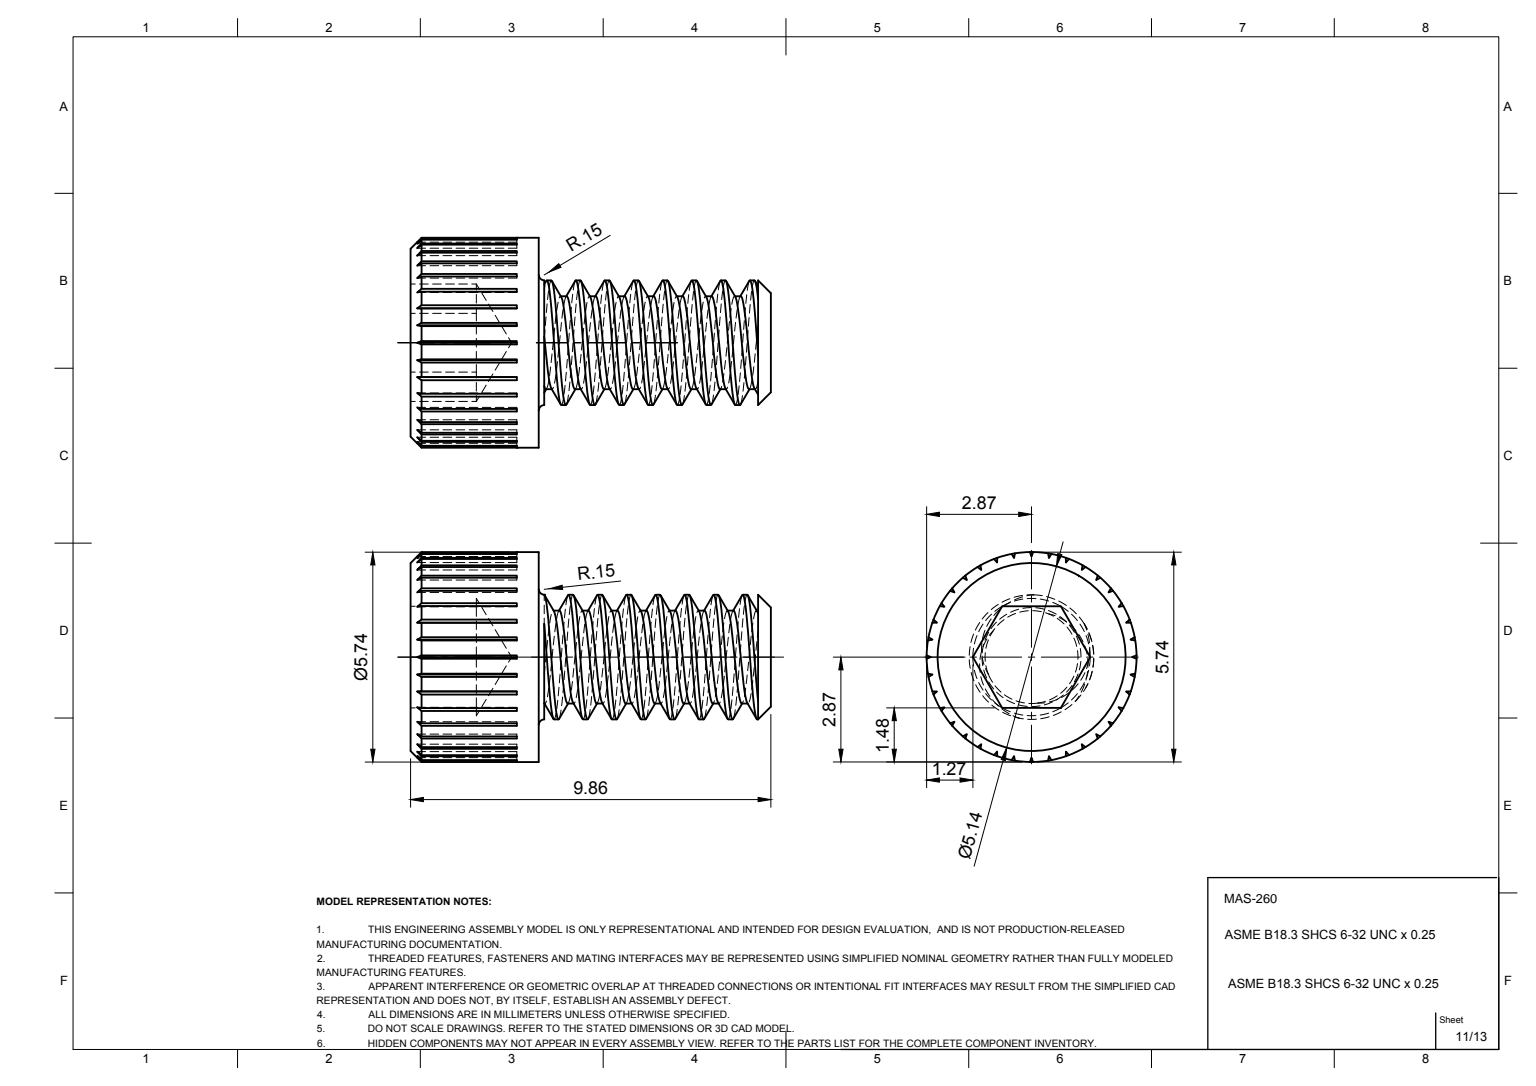
ISO-10303-21;
HEADER;
/* Generated by software containing ST-Developer
 * from STEP Tools, Inc. (www.steptools.com) 
 */

FILE_DESCRIPTION(
/* description */ (''),
/* implementation_level */ '2;1');

FILE_NAME(
/* name */ 'ASME B18.3 SHCS 6-32 UNC x 0.25.step',
/* time_stamp */ '2026-10-15T13:29:10-07:00',
/* author */ (''),
/* organization */ (''),
/* preprocessor_version */ 'ST-DEVELOPER v20.2',
/* originating_system */ 'Autodesk Translation Framework v15.15.0.0',
/* authorisation */ '');

FILE_SCHEMA (('AUTOMOTIVE_DESIGN { 1 0 10303 214 3 1 1 }'));
ENDSEC;

DATA;
#10=MECHANICAL_DESIGN_GEOMETRIC_PRESENTATION_REPRESENTATION('',(#942),#83219);
#281=(
BOUNDED_CURVE()
B_SPLINE_CURVE(2,(#58539,#58540,#58541),.UNSPECIFIED.,.F.,.F.)
B_SPLINE_CURVE_WITH_KNOTS((3,3),(0.,0.0169283274324264),.UNSPECIFIED.)
CURVE()
GEOMETRIC_REPRESENTATION_ITEM()
RATIONAL_B_SPLINE_CURVE((1.,1.00067437544971,1.00082963690249))
REPRESENTATION_ITEM('')
);
#282=(
BOUNDED_CURVE()
B_SPLINE_CURVE(2,(#58546,#58547,#58548),.UNSPECIFIED.,.F.,.F.)
B_SPLINE_CURVE_WITH_KNOTS((3,3),(0.0270544913418749,0.0439828187741895),
 .UNSPECIFIED.)
CURVE()
GEOMETRIC_REPRESENTATION_ITEM()
RATIONAL_B_SPLINE_CURVE((1.00082963691396,1.00067437545903,1.))
REPRESENTATION_ITEM('')
);
#283=(
BOUNDED_CURVE()
B_SPLINE_CURVE(2,(#58555,#58556,#58557),.UNSPECIFIED.,.F.,.F.)
B_SPLINE_CURVE_WITH_KNOTS((3,3),(0.0270544913418551,0.0439828187741901),
 .UNSPECIFIED.)
CURVE()
GEOMETRIC_REPRESENTATION_ITEM()
RATIONAL_B_SPLINE_CURVE((1.0008296369069,1.0006743754533,1.))
REPRESENTATION_ITEM('')
);
#284=(
BOUNDED_CURVE()
B_SPLINE_CURVE(2,(#58561,#58562,#58563),.UNSPECIFIED.,.F.,.F.)
B_SPLINE_CURVE_WITH_KNOTS((3,3),(0.,0.0169283274323742),.UNSPECIFIED.)
CURVE()
GEOMETRIC_REPRESENTATION_ITEM()
RATIONAL_B_SPLINE_CURVE((1.,1.00067437545167,1.0008296369049))
REPRESENTATION_ITEM('')
);
#285=(
BOUNDED_CURVE()
B_SPLINE_CURVE(2,(#58565,#58566,#58567),.UNSPECIFIED.,.F.,.F.)
B_SPLINE_CURVE_WITH_KNOTS((3,3),(0.0270544913418838,0.0439828187741893),
 .UNSPECIFIED.)
CURVE()
GEOMETRIC_REPRESENTATION_ITEM()
RATIONAL_B_SPLINE_CURVE((1.00082963690705,1.00067437545341,1.))
REPRESENTATION_ITEM('')
);
#286=(
BOUNDED_CURVE()
B_SPLINE_CURVE(2,(#58571,#58572,#58573),.UNSPECIFIED.,.F.,.F.)
B_SPLINE_CURVE_WITH_KNOTS((3,3),(0.,0.0169283274323636),.UNSPECIFIED.)
CURVE()
GEOMETRIC_REPRESENTATION_ITEM()
RATIONAL_B_SPLINE_CURVE((1.,1.00067437545192,1.00082963690521))
REPRESENTATION_ITEM('')
);
#287=(
BOUNDED_CURVE()
B_SPLINE_CURVE(2,(#58575,#58576,#58577),.UNSPECIFIED.,.F.,.F.)
B_SPLINE_CURVE_WITH_KNOTS((3,3),(0.0270544913418794,0.0439828187741893),
 .UNSPECIFIED.)
CURVE()
GEOMETRIC_REPRESENTATION_ITEM()
RATIONAL_B_SPLINE_CURVE((1.00082963691317,1.00067437545839,1.))
REPRESENTATION_ITEM('')
);
#288=(
BOUNDED_CURVE()
B_SPLINE_CURVE(2,(#58581,#58582,#58583),.UNSPECIFIED.,.F.,.F.)
B_SPLINE_CURVE_WITH_KNOTS((3,3),(0.,0.0169283274323019),.UNSPECIFIED.)
CURVE()
GEOMETRIC_REPRESENTATION_ITEM()
RATIONAL_B_SPLINE_CURVE((1.,1.0006743754572,1.00082963691171))
REPRESENTATION_ITEM('')
);
#289=(
BOUNDED_CURVE()
B_SPLINE_CURVE(2,(#58585,#58586,#58587),.UNSPECIFIED.,.F.,.F.)
B_SPLINE_CURVE_WITH_KNOTS((3,3),(0.0270544913418195,0.0439828187741896),
 .UNSPECIFIED.)
CURVE()
GEOMETRIC_REPRESENTATION_ITEM()
RATIONAL_B_SPLINE_CURVE((1.00082963691305,1.00067437545829,1.))
REPRESENTATION_ITEM('')
);
#290=(
BOUNDED_CURVE()
B_SPLINE_CURVE(2,(#58591,#58592,#58593),.UNSPECIFIED.,.F.,.F.)
B_SPLINE_CURVE_WITH_KNOTS((3,3),(0.,0.0169283274324256),.UNSPECIFIED.)
CURVE()
GEOMETRIC_REPRESENTATION_ITEM()
RATIONAL_B_SPLINE_CURVE((1.,1.00067437545036,1.00082963690329))
REPRESENTATION_ITEM('')
);
#291=(
BOUNDED_CURVE()
B_SPLINE_CURVE(2,(#58595,#58596,#58597),.UNSPECIFIED.,.F.,.F.)
B_SPLINE_CURVE_WITH_KNOTS((3,3),(0.0270544913418591,0.0439828187741892),
 .UNSPECIFIED.)
CURVE()
GEOMETRIC_REPRESENTATION_ITEM()
RATIONAL_B_SPLINE_CURVE((1.0008296369132,1.00067437545842,1.))
REPRESENTATION_ITEM('')
);
#292=(
BOUNDED_CURVE()
B_SPLINE_CURVE(2,(#58601,#58602,#58603),.UNSPECIFIED.,.F.,.F.)
B_SPLINE_CURVE_WITH_KNOTS((3,3),(0.,0.0169283274324107),.UNSPECIFIED.)
CURVE()
GEOMETRIC_REPRESENTATION_ITEM()
RATIONAL_B_SPLINE_CURVE((1.,1.00067437544792,1.00082963690028))
REPRESENTATION_ITEM('')
);
#293=(
BOUNDED_CURVE()
B_SPLINE_CURVE(2,(#58605,#58606,#58607),.UNSPECIFIED.,.F.,.F.)
B_SPLINE_CURVE_WITH_KNOTS((3,3),(0.0270544913419236,0.0439828187741892),
 .UNSPECIFIED.)
CURVE()
GEOMETRIC_REPRESENTATION_ITEM()
RATIONAL_B_SPLINE_CURVE((1.00082963691831,1.00067437546256,1.))
REPRESENTATION_ITEM('')
);
#294=(
BOUNDED_CURVE()
B_SPLINE_CURVE(2,(#58611,#58612,#58613),.UNSPECIFIED.,.F.,.F.)
B_SPLINE_CURVE_WITH_KNOTS((3,3),(0.,0.0169283274324074),.UNSPECIFIED.)
CURVE()
GEOMETRIC_REPRESENTATION_ITEM()
RATIONAL_B_SPLINE_CURVE((1.,1.00067437544939,1.00082963690209))
REPRESENTATION_ITEM('')
);
#295=(
BOUNDED_CURVE()
B_SPLINE_CURVE(2,(#58615,#58616,#58617),.UNSPECIFIED.,.F.,.F.)
B_SPLINE_CURVE_WITH_KNOTS((3,3),(0.0270544913418797,0.0439828187741898),
 .UNSPECIFIED.)
CURVE()
GEOMETRIC_REPRESENTATION_ITEM()
RATIONAL_B_SPLINE_CURVE((1.00082963691791,1.00067437546225,1.))
REPRESENTATION_ITEM('')
);
#296=(
BOUNDED_CURVE()
B_SPLINE_CURVE(2,(#58621,#58622,#58623),.UNSPECIFIED.,.F.,.F.)
B_SPLINE_CURVE_WITH_KNOTS((3,3),(0.,0.0169283274324609),.UNSPECIFIED.)
CURVE()
GEOMETRIC_REPRESENTATION_ITEM()
RATIONAL_B_SPLINE_CURVE((1.,1.00067437544233,1.00082963689341))
REPRESENTATION_ITEM('')
);
#297=(
BOUNDED_CURVE()
B_SPLINE_CURVE(2,(#58625,#58626,#58627),.UNSPECIFIED.,.F.,.F.)
B_SPLINE_CURVE_WITH_KNOTS((3,3),(0.0270544913417432,0.043982818774189),
 .UNSPECIFIED.)
CURVE()
GEOMETRIC_REPRESENTATION_ITEM()
RATIONAL_B_SPLINE_CURVE((1.00082963689481,1.00067437544347,1.))
REPRESENTATION_ITEM('')
);
#298=(
BOUNDED_CURVE()
B_SPLINE_CURVE(2,(#58631,#58632,#58633),.UNSPECIFIED.,.F.,.F.)
B_SPLINE_CURVE_WITH_KNOTS((3,3),(0.,0.0169283274323957),.UNSPECIFIED.)
CURVE()
GEOMETRIC_REPRESENTATION_ITEM()
RATIONAL_B_SPLINE_CURVE((1.,1.00067437545152,1.00082963690471))
REPRESENTATION_ITEM('')
);
#299=(
BOUNDED_CURVE()
B_SPLINE_CURVE(2,(#58635,#58636,#58637),.UNSPECIFIED.,.F.,.F.)
B_SPLINE_CURVE_WITH_KNOTS((3,3),(0.0270544913418118,0.043982818774189),
 .UNSPECIFIED.)
CURVE()
GEOMETRIC_REPRESENTATION_ITEM()
RATIONAL_B_SPLINE_CURVE((1.0008296369071,1.00067437545346,1.))
REPRESENTATION_ITEM('')
);
#300=(
BOUNDED_CURVE()
B_SPLINE_CURVE(2,(#58641,#58642,#58643),.UNSPECIFIED.,.F.,.F.)
B_SPLINE_CURVE_WITH_KNOTS((3,3),(0.,0.0169283274322737),.UNSPECIFIED.)
CURVE()
GEOMETRIC_REPRESENTATION_ITEM()
RATIONAL_B_SPLINE_CURVE((1.,1.00067437546411,1.00082963692021))
REPRESENTATION_ITEM('')
);
#301=(
BOUNDED_CURVE()
B_SPLINE_CURVE(2,(#58645,#58646,#58647),.UNSPECIFIED.,.F.,.F.)
B_SPLINE_CURVE_WITH_KNOTS((3,3),(0.0270544913418171,0.0439828187741889),
 .UNSPECIFIED.)
CURVE()
GEOMETRIC_REPRESENTATION_ITEM()
RATIONAL_B_SPLINE_CURVE((1.00082963690763,1.00067437545389,1.))
REPRESENTATION_ITEM('')
);
#302=(
BOUNDED_CURVE()
B_SPLINE_CURVE(2,(#58651,#58652,#58653),.UNSPECIFIED.,.F.,.F.)
B_SPLINE_CURVE_WITH_KNOTS((3,3),(0.,0.0169283274324309),.UNSPECIFIED.)
CURVE()
GEOMETRIC_REPRESENTATION_ITEM()
RATIONAL_B_SPLINE_CURVE((1.,1.00067437544897,1.00082963690158))
REPRESENTATION_ITEM('')
);
#303=(
BOUNDED_CURVE()
B_SPLINE_CURVE(2,(#58655,#58656,#58657),.UNSPECIFIED.,.F.,.F.)
B_SPLINE_CURVE_WITH_KNOTS((3,3),(0.0270544913417901,0.0439828187741889),
 .UNSPECIFIED.)
CURVE()
GEOMETRIC_REPRESENTATION_ITEM()
RATIONAL_B_SPLINE_CURVE((1.00082963690151,1.00067437544892,1.))
REPRESENTATION_ITEM('')
);
#304=(
BOUNDED_CURVE()
B_SPLINE_CURVE(2,(#58661,#58662,#58663),.UNSPECIFIED.,.F.,.F.)
B_SPLINE_CURVE_WITH_KNOTS((3,3),(0.,0.0169283274324599),.UNSPECIFIED.)
CURVE()
GEOMETRIC_REPRESENTATION_ITEM()
RATIONAL_B_SPLINE_CURVE((1.,1.00067437544707,1.00082963689925))
REPRESENTATION_ITEM('')
);
#305=(
BOUNDED_CURVE()
B_SPLINE_CURVE(2,(#58665,#58666,#58667),.UNSPECIFIED.,.F.,.F.)
B_SPLINE_CURVE_WITH_KNOTS((3,3),(0.0270544913417598,0.0439828187741897),
 .UNSPECIFIED.)
CURVE()
GEOMETRIC_REPRESENTATION_ITEM()
RATIONAL_B_SPLINE_CURVE((1.00082963689893,1.00067437544681,1.))
REPRESENTATION_ITEM('')
);
#306=(
BOUNDED_CURVE()
B_SPLINE_CURVE(2,(#58671,#58672,#58673),.UNSPECIFIED.,.F.,.F.)
B_SPLINE_CURVE_WITH_KNOTS((3,3),(0.,0.0169283274324799),.UNSPECIFIED.)
CURVE()
GEOMETRIC_REPRESENTATION_ITEM()
RATIONAL_B_SPLINE_CURVE((1.,1.00067437544677,1.00082963689888))
REPRESENTATION_ITEM('')
);
#307=(
BOUNDED_CURVE()
B_SPLINE_CURVE(2,(#58675,#58676,#58677),.UNSPECIFIED.,.F.,.F.)
B_SPLINE_CURVE_WITH_KNOTS((3,3),(0.0270544913418231,0.0439828187741892),
 .UNSPECIFIED.)
CURVE()
GEOMETRIC_REPRESENTATION_ITEM()
RATIONAL_B_SPLINE_CURVE((1.00082963690453,1.00067437545137,1.))
REPRESENTATION_ITEM('')
);
#308=(
BOUNDED_CURVE()
B_SPLINE_CURVE(2,(#58681,#58682,#58683),.UNSPECIFIED.,.F.,.F.)
B_SPLINE_CURVE_WITH_KNOTS((3,3),(0.,0.0169283274323869),.UNSPECIFIED.)
CURVE()
GEOMETRIC_REPRESENTATION_ITEM()
RATIONAL_B_SPLINE_CURVE((1.,1.00067437545224,1.0008296369056))
REPRESENTATION_ITEM('')
);
#309=(
BOUNDED_CURVE()
B_SPLINE_CURVE(2,(#58685,#58686,#58687),.UNSPECIFIED.,.F.,.F.)
B_SPLINE_CURVE_WITH_KNOTS((3,3),(0.0270544913417943,0.0439828187741897),
 .UNSPECIFIED.)
CURVE()
GEOMETRIC_REPRESENTATION_ITEM()
RATIONAL_B_SPLINE_CURVE((1.00082963690791,1.00067437545412,1.))
REPRESENTATION_ITEM('')
);
#310=(
BOUNDED_CURVE()
B_SPLINE_CURVE(2,(#58691,#58692,#58693),.UNSPECIFIED.,.F.,.F.)
B_SPLINE_CURVE_WITH_KNOTS((3,3),(0.,0.0169283274323051),.UNSPECIFIED.)
CURVE()
GEOMETRIC_REPRESENTATION_ITEM()
RATIONAL_B_SPLINE_CURVE((1.,1.00067437546317,1.00082963691906))
REPRESENTATION_ITEM('')
);
#311=(
BOUNDED_CURVE()
B_SPLINE_CURVE(2,(#58695,#58696,#58697),.UNSPECIFIED.,.F.,.F.)
B_SPLINE_CURVE_WITH_KNOTS((3,3),(0.027054491341705,0.0439828187741902),
 .UNSPECIFIED.)
CURVE()
GEOMETRIC_REPRESENTATION_ITEM()
RATIONAL_B_SPLINE_CURVE((1.00082963689389,1.00067437544272,1.))
REPRESENTATION_ITEM('')
);
#312=(
BOUNDED_CURVE()
B_SPLINE_CURVE(2,(#58701,#58702,#58703),.UNSPECIFIED.,.F.,.F.)
B_SPLINE_CURVE_WITH_KNOTS((3,3),(0.,0.0169283274323258),.UNSPECIFIED.)
CURVE()
GEOMETRIC_REPRESENTATION_ITEM()
RATIONAL_B_SPLINE_CURVE((1.,1.00067437545656,1.00082963691092))
REPRESENTATION_ITEM('')
);
#313=(
BOUNDED_CURVE()
B_SPLINE_CURVE(2,(#58705,#58706,#58707),.UNSPECIFIED.,.F.,.F.)
B_SPLINE_CURVE_WITH_KNOTS((3,3),(0.0270544913418574,0.0439828187741888),
 .UNSPECIFIED.)
CURVE()
GEOMETRIC_REPRESENTATION_ITEM()
RATIONAL_B_SPLINE_CURVE((1.00082963691715,1.00067437546163,1.))
REPRESENTATION_ITEM('')
);
#314=(
BOUNDED_CURVE()
B_SPLINE_CURVE(2,(#58711,#58712,#58713),.UNSPECIFIED.,.F.,.F.)
B_SPLINE_CURVE_WITH_KNOTS((3,3),(0.,0.0169283274323776),.UNSPECIFIED.)
CURVE()
GEOMETRIC_REPRESENTATION_ITEM()
RATIONAL_B_SPLINE_CURVE((1.,1.00067437544935,1.00082963690205))
REPRESENTATION_ITEM('')
);
#315=(
BOUNDED_CURVE()
B_SPLINE_CURVE(2,(#58715,#58716,#58717),.UNSPECIFIED.,.F.,.F.)
B_SPLINE_CURVE_WITH_KNOTS((3,3),(0.0270544913418392,0.0439828187741898),
 .UNSPECIFIED.)
CURVE()
GEOMETRIC_REPRESENTATION_ITEM()
RATIONAL_B_SPLINE_CURVE((1.00082963690784,1.00067437545406,1.))
REPRESENTATION_ITEM('')
);
#316=(
BOUNDED_CURVE()
B_SPLINE_CURVE(2,(#58721,#58722,#58723),.UNSPECIFIED.,.F.,.F.)
B_SPLINE_CURVE_WITH_KNOTS((3,3),(0.,0.0169283274323582),.UNSPECIFIED.)
CURVE()
GEOMETRIC_REPRESENTATION_ITEM()
RATIONAL_B_SPLINE_CURVE((1.,1.0006743754544,1.00082963690826))
REPRESENTATION_ITEM('')
);
#317=(
BOUNDED_CURVE()
B_SPLINE_CURVE(2,(#58725,#58726,#58727),.UNSPECIFIED.,.F.,.F.)
B_SPLINE_CURVE_WITH_KNOTS((3,3),(0.0270544913418716,0.0439828187741891),
 .UNSPECIFIED.)
CURVE()
GEOMETRIC_REPRESENTATION_ITEM()
RATIONAL_B_SPLINE_CURVE((1.00082963691279,1.00067437545808,1.))
REPRESENTATION_ITEM('')
);
#318=(
BOUNDED_CURVE()
B_SPLINE_CURVE(2,(#58731,#58732,#58733),.UNSPECIFIED.,.F.,.F.)
B_SPLINE_CURVE_WITH_KNOTS((3,3),(0.,0.0169283274323239),.UNSPECIFIED.)
CURVE()
GEOMETRIC_REPRESENTATION_ITEM()
RATIONAL_B_SPLINE_CURVE((1.,1.00067437545309,1.00082963690665))
REPRESENTATION_ITEM('')
);
#319=(
BOUNDED_CURVE()
B_SPLINE_CURVE(2,(#58735,#58736,#58737),.UNSPECIFIED.,.F.,.F.)
B_SPLINE_CURVE_WITH_KNOTS((3,3),(0.0270544913418909,0.0439828187741894),
 .UNSPECIFIED.)
CURVE()
GEOMETRIC_REPRESENTATION_ITEM()
RATIONAL_B_SPLINE_CURVE((1.00082963691804,1.00067437546234,1.))
REPRESENTATION_ITEM('')
);
#320=(
BOUNDED_CURVE()
B_SPLINE_CURVE(2,(#58741,#58742,#58743),.UNSPECIFIED.,.F.,.F.)
B_SPLINE_CURVE_WITH_KNOTS((3,3),(0.,0.0169283274323187),.UNSPECIFIED.)
CURVE()
GEOMETRIC_REPRESENTATION_ITEM()
RATIONAL_B_SPLINE_CURVE((1.,1.00067437545808,1.00082963691279))
REPRESENTATION_ITEM('')
);
#321=(
BOUNDED_CURVE()
B_SPLINE_CURVE(2,(#58745,#58746,#58747),.UNSPECIFIED.,.F.,.F.)
B_SPLINE_CURVE_WITH_KNOTS((3,3),(0.0270544913417975,0.0439828187741893),
 .UNSPECIFIED.)
CURVE()
GEOMETRIC_REPRESENTATION_ITEM()
RATIONAL_B_SPLINE_CURVE((1.00082963690175,1.00067437544911,1.))
REPRESENTATION_ITEM('')
);
#322=(
BOUNDED_CURVE()
B_SPLINE_CURVE(2,(#58751,#58752,#58753),.UNSPECIFIED.,.F.,.F.)
B_SPLINE_CURVE_WITH_KNOTS((3,3),(0.,0.0169283274323514),.UNSPECIFIED.)
CURVE()
GEOMETRIC_REPRESENTATION_ITEM()
RATIONAL_B_SPLINE_CURVE((1.,1.00067437545079,1.00082963690382))
REPRESENTATION_ITEM('')
);
#323=(
BOUNDED_CURVE()
B_SPLINE_CURVE(2,(#58755,#58756,#58757),.UNSPECIFIED.,.F.,.F.)
B_SPLINE_CURVE_WITH_KNOTS((3,3),(0.0270544913418461,0.043982818774189),
 .UNSPECIFIED.)
CURVE()
GEOMETRIC_REPRESENTATION_ITEM()
RATIONAL_B_SPLINE_CURVE((1.00082963691007,1.00067437545587,1.))
REPRESENTATION_ITEM('')
);
#324=(
BOUNDED_CURVE()
B_SPLINE_CURVE(2,(#58761,#58762,#58763),.UNSPECIFIED.,.F.,.F.)
B_SPLINE_CURVE_WITH_KNOTS((3,3),(0.,0.0169283274323367),.UNSPECIFIED.)
CURVE()
GEOMETRIC_REPRESENTATION_ITEM()
RATIONAL_B_SPLINE_CURVE((1.,1.00067437545527,1.00082963690933))
REPRESENTATION_ITEM('')
);
#325=(
BOUNDED_CURVE()
B_SPLINE_CURVE(2,(#58765,#58766,#58767),.UNSPECIFIED.,.F.,.F.)
B_SPLINE_CURVE_WITH_KNOTS((3,3),(0.0270544913418436,0.0439828187741888),
 .UNSPECIFIED.)
CURVE()
GEOMETRIC_REPRESENTATION_ITEM()
RATIONAL_B_SPLINE_CURVE((1.00082963691215,1.00067437545756,1.))
REPRESENTATION_ITEM('')
);
#326=(
BOUNDED_CURVE()
B_SPLINE_CURVE(2,(#58771,#58772,#58773),.UNSPECIFIED.,.F.,.F.)
B_SPLINE_CURVE_WITH_KNOTS((3,3),(0.,0.0169283274324564),.UNSPECIFIED.)
CURVE()
GEOMETRIC_REPRESENTATION_ITEM()
RATIONAL_B_SPLINE_CURVE((1.,1.00067437544799,1.00082963690037))
REPRESENTATION_ITEM('')
);
#327=(
BOUNDED_CURVE()
B_SPLINE_CURVE(2,(#58775,#58776,#58777),.UNSPECIFIED.,.F.,.F.)
B_SPLINE_CURVE_WITH_KNOTS((3,3),(0.0270544913419147,0.0439828187741882),
 .UNSPECIFIED.)
CURVE()
GEOMETRIC_REPRESENTATION_ITEM()
RATIONAL_B_SPLINE_CURVE((1.00082963691331,1.00067437545851,1.))
REPRESENTATION_ITEM('')
);
#328=(
BOUNDED_CURVE()
B_SPLINE_CURVE(2,(#58781,#58782,#58783),.UNSPECIFIED.,.F.,.F.)
B_SPLINE_CURVE_WITH_KNOTS((3,3),(0.,0.0169283274324423),.UNSPECIFIED.)
CURVE()
GEOMETRIC_REPRESENTATION_ITEM()
RATIONAL_B_SPLINE_CURVE((1.,1.00067437544741,1.00082963689965))
REPRESENTATION_ITEM('')
);
#329=(
BOUNDED_CURVE()
B_SPLINE_CURVE(2,(#58785,#58786,#58787),.UNSPECIFIED.,.F.,.F.)
B_SPLINE_CURVE_WITH_KNOTS((3,3),(0.0270544913418278,0.0439828187741883),
 .UNSPECIFIED.)
CURVE()
GEOMETRIC_REPRESENTATION_ITEM()
RATIONAL_B_SPLINE_CURVE((1.00082963690487,1.00067437545164,1.))
REPRESENTATION_ITEM('')
);
#330=(
BOUNDED_CURVE()
B_SPLINE_CURVE(2,(#58791,#58792,#58793),.UNSPECIFIED.,.F.,.F.)
B_SPLINE_CURVE_WITH_KNOTS((3,3),(0.,0.0169283274324055),.UNSPECIFIED.)
CURVE()
GEOMETRIC_REPRESENTATION_ITEM()
RATIONAL_B_SPLINE_CURVE((1.,1.00067437544812,1.00082963690053))
REPRESENTATION_ITEM('')
);
#331=(
BOUNDED_CURVE()
B_SPLINE_CURVE(2,(#58795,#58796,#58797),.UNSPECIFIED.,.F.,.F.)
B_SPLINE_CURVE_WITH_KNOTS((3,3),(0.0270544913418545,0.0439828187741889),
 .UNSPECIFIED.)
CURVE()
GEOMETRIC_REPRESENTATION_ITEM()
RATIONAL_B_SPLINE_CURVE((1.00082963690979,1.00067437545564,1.))
REPRESENTATION_ITEM('')
);
#332=(
BOUNDED_CURVE()
B_SPLINE_CURVE(2,(#58801,#58802,#58803),.UNSPECIFIED.,.F.,.F.)
B_SPLINE_CURVE_WITH_KNOTS((3,3),(0.,0.016928327432381),.UNSPECIFIED.)
CURVE()
GEOMETRIC_REPRESENTATION_ITEM()
RATIONAL_B_SPLINE_CURVE((1.,1.0006743754549,1.00082963690887))
REPRESENTATION_ITEM('')
);
#333=(
BOUNDED_CURVE()
B_SPLINE_CURVE(2,(#58805,#58806,#58807),.UNSPECIFIED.,.F.,.F.)
B_SPLINE_CURVE_WITH_KNOTS((3,3),(0.0270544913418599,0.043982818774188),
 .UNSPECIFIED.)
CURVE()
GEOMETRIC_REPRESENTATION_ITEM()
RATIONAL_B_SPLINE_CURVE((1.00082963691264,1.00067437545796,1.))
REPRESENTATION_ITEM('')
);
#334=(
BOUNDED_CURVE()
B_SPLINE_CURVE(2,(#58811,#58812,#58813),.UNSPECIFIED.,.F.,.F.)
B_SPLINE_CURVE_WITH_KNOTS((3,3),(0.,0.0169283274323032),.UNSPECIFIED.)
CURVE()
GEOMETRIC_REPRESENTATION_ITEM()
RATIONAL_B_SPLINE_CURVE((1.,1.00067437546434,1.00082963692049))
REPRESENTATION_ITEM('')
);
#335=(
BOUNDED_CURVE()
B_SPLINE_CURVE(2,(#58815,#58816,#58817),.UNSPECIFIED.,.F.,.F.)
B_SPLINE_CURVE_WITH_KNOTS((3,3),(0.0270544913418524,0.0439828187741887),
 .UNSPECIFIED.)
CURVE()
GEOMETRIC_REPRESENTATION_ITEM()
RATIONAL_B_SPLINE_CURVE((1.00082963690961,1.0006743754555,1.))
REPRESENTATION_ITEM('')
);
#336=(
BOUNDED_CURVE()
B_SPLINE_CURVE(2,(#58821,#58822,#58823),.UNSPECIFIED.,.F.,.F.)
B_SPLINE_CURVE_WITH_KNOTS((3,3),(0.,0.0169283274323137),.UNSPECIFIED.)
CURVE()
GEOMETRIC_REPRESENTATION_ITEM()
RATIONAL_B_SPLINE_CURVE((1.,1.00067437546296,1.00082963691879))
REPRESENTATION_ITEM('')
);
#337=(
BOUNDED_CURVE()
B_SPLINE_CURVE(2,(#58825,#58826,#58827),.UNSPECIFIED.,.F.,.F.)
B_SPLINE_CURVE_WITH_KNOTS((3,3),(0.0270544913418263,0.0439828187741885),
 .UNSPECIFIED.)
CURVE()
GEOMETRIC_REPRESENTATION_ITEM()
RATIONAL_B_SPLINE_CURVE((1.00082963691197,1.00067437545741,1.))
REPRESENTATION_ITEM('')
);
#338=(
BOUNDED_CURVE()
B_SPLINE_CURVE(2,(#58832,#58833,#58834),.UNSPECIFIED.,.F.,.F.)
B_SPLINE_CURVE_WITH_KNOTS((3,3),(0.,0.0169283274323449),.UNSPECIFIED.)
CURVE()
GEOMETRIC_REPRESENTATION_ITEM()
RATIONAL_B_SPLINE_CURVE((1.,1.00067437545405,1.00082963690783))
REPRESENTATION_ITEM('')
);
#339=(
BOUNDED_CURVE()
B_SPLINE_CURVE(2,(#58836,#58837,#58838),.UNSPECIFIED.,.F.,.F.)
B_SPLINE_CURVE_WITH_KNOTS((3,3),(0.0270544913417649,0.0439828187741904),
 .UNSPECIFIED.)
CURVE()
GEOMETRIC_REPRESENTATION_ITEM()
RATIONAL_B_SPLINE_CURVE((1.00082963690075,1.0006743754483,1.))
REPRESENTATION_ITEM('')
);
#340=(
BOUNDED_CURVE()
B_SPLINE_CURVE(2,(#58842,#58843,#58844),.UNSPECIFIED.,.F.,.F.)
B_SPLINE_CURVE_WITH_KNOTS((3,3),(0.,0.0169283274323657),.UNSPECIFIED.)
CURVE()
GEOMETRIC_REPRESENTATION_ITEM()
RATIONAL_B_SPLINE_CURVE((1.,1.00067437545132,1.00082963690448))
REPRESENTATION_ITEM('')
);
#341=(
BOUNDED_CURVE()
B_SPLINE_CURVE(2,(#58846,#58847,#58848),.UNSPECIFIED.,.F.,.F.)
B_SPLINE_CURVE_WITH_KNOTS((3,3),(0.0270544913418314,0.0439828187741895),
 .UNSPECIFIED.)
CURVE()
GEOMETRIC_REPRESENTATION_ITEM()
RATIONAL_B_SPLINE_CURVE((1.00082963690259,1.00067437544979,1.))
REPRESENTATION_ITEM('')
);
#342=(
BOUNDED_CURVE()
B_SPLINE_CURVE(2,(#58852,#58853,#58854),.UNSPECIFIED.,.F.,.F.)
B_SPLINE_CURVE_WITH_KNOTS((3,3),(0.,0.0169283274324112),.UNSPECIFIED.)
CURVE()
GEOMETRIC_REPRESENTATION_ITEM()
RATIONAL_B_SPLINE_CURVE((1.,1.00067437544367,1.00082963689506))
REPRESENTATION_ITEM('')
);
#343=(
BOUNDED_CURVE()
B_SPLINE_CURVE(2,(#58856,#58857,#58858),.UNSPECIFIED.,.F.,.F.)
B_SPLINE_CURVE_WITH_KNOTS((3,3),(0.0270544913417055,0.0439828187741905),
 .UNSPECIFIED.)
CURVE()
GEOMETRIC_REPRESENTATION_ITEM()
RATIONAL_B_SPLINE_CURVE((1.00082963689237,1.00067437544149,1.))
REPRESENTATION_ITEM('')
);
#344=(
BOUNDED_CURVE()
B_SPLINE_CURVE(2,(#58862,#58863,#58864),.UNSPECIFIED.,.F.,.F.)
B_SPLINE_CURVE_WITH_KNOTS((3,3),(0.,0.0169283274324376),.UNSPECIFIED.)
CURVE()
GEOMETRIC_REPRESENTATION_ITEM()
RATIONAL_B_SPLINE_CURVE((1.,1.0006743754461,1.00082963689805))
REPRESENTATION_ITEM('')
);
#345=(
BOUNDED_CURVE()
B_SPLINE_CURVE(2,(#58866,#58867,#58868),.UNSPECIFIED.,.F.,.F.)
B_SPLINE_CURVE_WITH_KNOTS((3,3),(0.0270544913417534,0.0439828187741907),
 .UNSPECIFIED.)
CURVE()
GEOMETRIC_REPRESENTATION_ITEM()
RATIONAL_B_SPLINE_CURVE((1.00082963689691,1.00067437544518,1.))
REPRESENTATION_ITEM('')
);
#346=(
BOUNDED_CURVE()
B_SPLINE_CURVE(2,(#58872,#58873,#58874),.UNSPECIFIED.,.F.,.F.)
B_SPLINE_CURVE_WITH_KNOTS((3,3),(0.,0.0169283274323307),.UNSPECIFIED.)
CURVE()
GEOMETRIC_REPRESENTATION_ITEM()
RATIONAL_B_SPLINE_CURVE((1.,1.00067437545699,1.00082963691144))
REPRESENTATION_ITEM('')
);
#347=(
BOUNDED_CURVE()
B_SPLINE_CURVE(2,(#58876,#58877,#58878),.UNSPECIFIED.,.F.,.F.)
B_SPLINE_CURVE_WITH_KNOTS((3,3),(0.0270544913418834,0.0439828187741894),
 .UNSPECIFIED.)
CURVE()
GEOMETRIC_REPRESENTATION_ITEM()
RATIONAL_B_SPLINE_CURVE((1.00082963691786,1.0006743754622,1.))
REPRESENTATION_ITEM('')
);
#348=(
BOUNDED_CURVE()
B_SPLINE_CURVE(2,(#58882,#58883,#58884),.UNSPECIFIED.,.F.,.F.)
B_SPLINE_CURVE_WITH_KNOTS((3,3),(0.,0.0169283274324524),.UNSPECIFIED.)
CURVE()
GEOMETRIC_REPRESENTATION_ITEM()
RATIONAL_B_SPLINE_CURVE((1.,1.000674375448,1.00082963690039))
REPRESENTATION_ITEM('')
);
#349=(
BOUNDED_CURVE()
B_SPLINE_CURVE(2,(#58886,#58887,#58888),.UNSPECIFIED.,.F.,.F.)
B_SPLINE_CURVE_WITH_KNOTS((3,3),(0.027054491341806,0.0439828187741904),
 .UNSPECIFIED.)
CURVE()
GEOMETRIC_REPRESENTATION_ITEM()
RATIONAL_B_SPLINE_CURVE((1.00082963690582,1.00067437545241,1.))
REPRESENTATION_ITEM('')
);
#350=(
BOUNDED_CURVE()
B_SPLINE_CURVE(2,(#58892,#58893,#58894),.UNSPECIFIED.,.F.,.F.)
B_SPLINE_CURVE_WITH_KNOTS((3,3),(0.,0.0169283274324273),.UNSPECIFIED.)
CURVE()
GEOMETRIC_REPRESENTATION_ITEM()
RATIONAL_B_SPLINE_CURVE((1.,1.00067437544657,1.00082963689862))
REPRESENTATION_ITEM('')
);
#351=(
BOUNDED_CURVE()
B_SPLINE_CURVE(2,(#58896,#58897,#58898),.UNSPECIFIED.,.F.,.F.)
B_SPLINE_CURVE_WITH_KNOTS((3,3),(0.0270544913418182,0.04398281877419),
 .UNSPECIFIED.)
CURVE()
GEOMETRIC_REPRESENTATION_ITEM()
RATIONAL_B_SPLINE_CURVE((1.00082963691171,1.0006743754572,1.))
REPRESENTATION_ITEM('')
);
#352=(
BOUNDED_CURVE()
B_SPLINE_CURVE(2,(#58901,#58902,#58903),.UNSPECIFIED.,.F.,.F.)
B_SPLINE_CURVE_WITH_KNOTS((3,3),(0.,0.0169283274324202),.UNSPECIFIED.)
CURVE()
GEOMETRIC_REPRESENTATION_ITEM()
RATIONAL_B_SPLINE_CURVE((1.,1.00067437545079,1.00082963690381))
REPRESENTATION_ITEM('')
);
#505=TOROIDAL_SURFACE('',#28481,1.85434,0.15);
#645=B_SPLINE_CURVE_WITH_KNOTS('',3,(#53163,#53164,#53165,#53166,#53167,
#53168,#53169,#53170,#53171,#53172,#53173,#53174,#53175,#53176,#53177,#53178,
#53179,#53180,#53181,#53182,#53183,#53184,#53185,#53186,#53187,#53188,#53189,
#53190,#53191,#53192,#53193,#53194,#53195,#53196,#53197,#53198,#53199,#53200,
#53201,#53202,#53203,#53204,#53205,#53206,#53207,#53208,#53209,#53210,#53211,
#53212,#53213,#53214,#53215,#53216,#53217,#53218,#53219,#53220,#53221,#53222,
#53223,#53224,#53225,#53226,#53227,#53228,#53229,#53230,#53231,#53232,#53233,
#53234,#53235,#53236,#53237,#53238,#53239,#53240,#53241,#53242,#53243,#53244,
#53245,#53246,#53247,#53248,#53249,#53250,#53251,#53252,#53253,#53254,#53255,
#53256,#53257,#53258,#53259,#53260,#53261,#53262,#53263,#53264,#53265,#53266,
#53267,#53268),.UNSPECIFIED.,.F.,.F.,(4,2,2,2,2,2,2,2,2,2,2,2,2,2,2,2,2,
2,2,2,2,2,2,2,2,2,2,2,2,2,2,2,2,2,2,2,2,2,2,2,2,2,2,2,2,2,2,2,2,2,2,2,4),
(-0.578057800930158,-0.576907658226536,-0.568154833588687,-0.561138999497065,
-0.552272437437979,-0.542064916508128,-0.517889363717969,-0.507443620840254,
-0.5026023411279,-0.498401345318794,-0.491060740642357,-0.469791252118237,
-0.451026489857121,-0.442347794318625,-0.435320724528266,-0.426342970288697,
-0.415944588322965,-0.390451736003233,-0.380837795881047,-0.376307614792867,
-0.371965237536568,-0.363532324173621,-0.350556965963959,-0.324775865056773,
-0.316215461473166,-0.309236126491577,-0.30027545529445,-0.289876340707482,
-0.264214578438879,-0.254775349788872,-0.250280578846039,-0.245883566264983,
-0.237234369709441,-0.223717989369306,-0.199058992042047,-0.190354569511272,
-0.1833018149302,-0.174278579622026,-0.163807016827302,-0.137775149213679,
-0.12869300762222,-0.124216054466084,-0.119638119348461,-0.109986931187581,
-0.0934027038767481,-0.0743184018899234,-0.0656129882769852,-0.0585836505909147,
-0.0494613038761158,-0.0260871743460905,-0.0069322348740228,-0.00303082776048378,
-0.00159986386543374),.UNSPECIFIED.);
#646=B_SPLINE_CURVE_WITH_KNOTS('',3,(#53271,#53272,#53273,#53274,#53275,
#53276,#53277,#53278,#53279,#53280,#53281,#53282,#53283,#53284,#53285,#53286,
#53287,#53288,#53289,#53290,#53291,#53292,#53293,#53294,#53295,#53296,#53297,
#53298,#53299,#53300,#53301,#53302,#53303,#53304,#53305,#53306,#53307,#53308,
#53309,#53310,#53311,#53312,#53313,#53314,#53315,#53316,#53317,#53318,#53319,
#53320,#53321,#53322,#53323,#53324,#53325,#53326,#53327,#53328,#53329,#53330,
#53331,#53332,#53333,#53334,#53335,#53336,#53337,#53338,#53339,#53340,#53341,
#53342,#53343,#53344),.UNSPECIFIED.,.F.,.F.,(4,2,2,2,2,2,2,2,2,2,2,2,2,
2,2,2,2,2,2,2,2,2,2,2,2,2,2,2,2,2,2,2,2,2,2,2,4),(-1.31816221225193,-1.31512894288896,
-1.31135704736811,-1.29605024055882,-1.27729638040057,-1.26581126211065,
-1.25797720490834,-1.2490398174757,-1.2250784758911,-1.20789126545402,-1.20072619108313,
-1.19494117273146,-1.19093691780624,-1.18558492912948,-1.16407570760206,
-1.14133523638755,-1.13327775490148,-1.12654658814491,-1.11792602250525,
-1.09490240366976,-1.07980411050715,-1.07323777199083,-1.06788103747146,
-1.06394552068814,-1.05828956237135,-1.03953710342389,-1.01571751125415,
-1.00661207639585,-0.999520056879496,-0.990771470388567,-0.97089804755582,
-0.954929106573042,-0.945466425191204,-0.940915981340912,-0.936417949046409,
-0.927487378930933,-0.911920807669219),.UNSPECIFIED.);
#647=B_SPLINE_CURVE_WITH_KNOTS('',3,(#53349,#53350,#53351,#53352,#53353,
#53354,#53355,#53356,#53357,#53358,#53359,#53360,#53361,#53362,#53363,#53364,
#53365,#53366,#53367,#53368,#53369,#53370,#53371,#53372,#53373,#53374,#53375,
#53376,#53377,#53378,#53379,#53380,#53381,#53382,#53383,#53384,#53385,#53386,
#53387,#53388,#53389,#53390,#53391,#53392,#53393,#53394,#53395,#53396,#53397,
#53398,#53399,#53400,#53401,#53402,#53403,#53404,#53405,#53406,#53407,#53408,
#53409,#53410,#53411,#53412,#53413,#53414,#53415,#53416,#53417,#53418,#53419,
#53420,#53421,#53422,#53423,#53424,#53425,#53426,#53427,#53428,#53429,#53430,
#53431,#53432,#53433,#53434,#53435,#53436,#53437,#53438,#53439,#53440,#53441,
#53442,#53443,#53444,#53445,#53446,#53447,#53448,#53449,#53450,#53451,#53452,
#53453,#53454,#53455,#53456,#53457,#53458,#53459,#53460,#53461,#53462,#53463,
#53464,#53465,#53466,#53467,#53468,#53469,#53470,#53471,#53472,#53473,#53474,
#53475,#53476,#53477,#53478,#53479,#53480,#53481,#53482,#53483,#53484,#53485,
#53486,#53487,#53488,#53489,#53490,#53491,#53492,#53493,#53494,#53495,#53496),
 .UNSPECIFIED.,.F.,.F.,(4,2,2,2,2,2,2,2,2,2,2,2,2,2,2,2,2,2,2,2,2,2,2,2,
2,2,2,2,2,2,2,2,2,2,2,2,2,2,2,2,2,2,2,2,2,2,2,2,2,2,2,2,2,2,2,2,2,2,2,2,
2,2,2,2,2,2,2,2,2,2,2,2,2,4),(-1.37994316952968,-1.37689311227225,-1.36682573652866,
-1.34228042207965,-1.33202475129869,-1.32313094817597,-1.31611795587767,
-1.30739915888195,-1.28345678192069,-1.26961972562278,-1.26086349964075,
-1.25645905792183,-1.25196785707959,-1.2426230896204,-1.22097924337118,
-1.2087485365401,-1.19879870812078,-1.19171700533154,-1.18367974843681,
-1.1651250047271,-1.14612917760861,-1.13877225267984,-1.13292305703663,
-1.12887646598579,-1.12323947896202,-1.10319838297259,-1.08670439419831,
-1.08108591203388,-1.07194741411961,-1.06492766049471,-1.05641623486836,
-1.03001574518196,-1.01736420210715,-1.00905268906645,-1.00471540075752,
-1.00014327199197,-0.990211241284662,-0.965107144749355,-0.954773421513134,
-0.94583592876078,-0.938822168802323,-0.930143076508692,-0.91133644834229,
-0.890012183713333,-0.882655960278845,-0.878459217734409,-0.873639573360281,
-0.862318089220826,-0.838779608238446,-0.828672057832893,-0.819861300618453,
-0.812847681281455,-0.804045278229529,-0.782707006762665,-0.767297417203463,
-0.760610652389874,-0.755136771563515,-0.751084486821065,-0.745045636921343,
-0.737339368803087,-0.716084657156016,-0.700217472411605,-0.692285062837235,
-0.685183498483941,-0.675005742963352,-0.66834101175725,-0.645395392510605,
-0.633855154214012,-0.628786809333242,-0.624674683771948,-0.617965940192248,
-0.613254767023967,-0.596707640675902,-0.578057800930158),.UNSPECIFIED.);
#648=B_SPLINE_CURVE_WITH_KNOTS('',3,(#53497,#53498,#53499,#53500,#53501,
#53502,#53503,#53504,#53505,#53506,#53507,#53508,#53509,#53510,#53511,#53512,
#53513,#53514,#53515,#53516,#53517,#53518,#53519,#53520,#53521,#53522,#53523,
#53524,#53525,#53526,#53527,#53528,#53529,#53530,#53531,#53532,#53533,#53534,
#53535,#53536,#53537,#53538,#53539,#53540,#53541,#53542,#53543,#53544,#53545,
#53546,#53547,#53548,#53549,#53550,#53551,#53552,#53553,#53554,#53555,#53556,
#53557,#53558,#53559,#53560,#53561,#53562,#53563,#53564,#53565,#53566,#53567,
#53568,#53569,#53570,#53571,#53572,#53573,#53574,#53575,#53576,#53577,#53578,
#53579,#53580,#53581,#53582,#53583,#53584,#53585,#53586,#53587,#53588,#53589,
#53590,#53591,#53592,#53593,#53594,#53595,#53596,#53597,#53598,#53599,#53600,
#53601,#53602,#53603,#53604,#53605,#53606,#53607,#53608,#53609,#53610,#53611,
#53612,#53613,#53614,#53615,#53616,#53617,#53618,#53619,#53620,#53621,#53622,
#53623,#53624,#53625,#53626,#53627,#53628,#53629,#53630,#53631,#53632,#53633,
#53634,#53635,#53636,#53637,#53638,#53639,#53640,#53641,#53642),
 .UNSPECIFIED.,.F.,.F.,(4,2,2,2,2,2,2,2,2,2,2,2,2,2,2,2,2,2,2,2,2,2,2,2,
2,2,2,2,2,2,2,2,2,2,2,2,2,2,2,2,2,2,2,2,2,2,2,2,2,2,2,2,2,2,2,2,2,2,2,2,
2,2,2,2,2,2,2,2,2,2,2,2,4),(-0.911920807669219,-0.90143765389995,-0.886745109987811,
-0.87905985210302,-0.871885995371558,-0.860765107176676,-0.834212388433582,
-0.824970278238165,-0.818140331658867,-0.814012239618955,-0.809013408073738,
-0.796547838803406,-0.774191110932913,-0.767613995717944,-0.757532710564437,
-0.750470423755175,-0.742567775145225,-0.725784833814838,-0.705083680534938,
-0.697460900871011,-0.691472842001079,-0.687435402051852,-0.682064717154924,
-0.659379246119088,-0.638518233901586,-0.629717651584906,-0.622695306396698,
-0.613856573362942,-0.603699302204386,-0.579837876380211,-0.569131574410963,
-0.564259621347492,-0.560074172934118,-0.552823844565205,-0.531588824368177,
-0.512603164050812,-0.503909708727391,-0.496894653818284,-0.487968840160277,
-0.477656051512273,-0.452752791453641,-0.442968809586499,-0.438234994374704,
-0.434001687320285,-0.426379261067704,-0.404707709530608,-0.386580270569894,
-0.377961326143986,-0.370950953858479,-0.361959900002634,-0.351525889175323,
-0.32570200703561,-0.316397229918055,-0.311913413010029,-0.307505901145109,
-0.298730296056676,-0.284840018172648,-0.261030113633416,-0.252304893487327,
-0.245290405886381,-0.236399180714257,-0.22614706440424,-0.201660461140628,
-0.191511997882101,-0.186716411225593,-0.18250846607308,-0.175076221179508,
-0.153660023347993,-0.135060083361694,-0.126397217303569,-0.119382399277055,
-0.110425404253977,-0.109945337718666),.UNSPECIFIED.);
#649=B_SPLINE_CURVE_WITH_KNOTS('',3,(#53648,#53649,#53650,#53651,#53652,
#53653,#53654,#53655,#53656,#53657,#53658,#53659,#53660,#53661,#53662,#53663,
#53664,#53665,#53666,#53667,#53668,#53669,#53670,#53671,#53672,#53673,#53674,
#53675,#53676,#53677,#53678,#53679,#53680,#53681,#53682,#53683,#53684,#53685,
#53686,#53687,#53688,#53689,#53690,#53691,#53692,#53693,#53694,#53695,#53696,
#53697,#53698,#53699,#53700,#53701,#53702,#53703,#53704,#53705,#53706,#53707,
#53708,#53709,#53710,#53711,#53712,#53713,#53714,#53715,#53716,#53717,#53718,
#53719,#53720,#53721,#53722,#53723,#53724,#53725,#53726,#53727,#53728,#53729,
#53730,#53731,#53732,#53733,#53734,#53735,#53736,#53737,#53738,#53739,#53740,
#53741,#53742,#53743,#53744,#53745,#53746,#53747,#53748,#53749,#53750,#53751,
#53752,#53753,#53754,#53755,#53756,#53757,#53758,#53759,#53760,#53761,#53762,
#53763,#53764,#53765,#53766,#53767,#53768,#53769,#53770,#53771,#53772,#53773,
#53774,#53775),.UNSPECIFIED.,.F.,.F.,(4,2,2,2,2,2,2,2,2,2,2,2,2,2,2,2,2,
2,2,2,2,2,2,2,2,2,2,2,2,2,2,2,2,2,2,2,2,2,2,2,2,2,2,2,2,2,2,2,2,2,2,2,2,
2,2,2,2,2,2,2,2,2,2,4),(-0.692748904775942,-0.676235309369303,-0.655372660470089,
-0.650315787459615,-0.646259718221949,-0.640812265724851,-0.634173194557436,
-0.618984651933166,-0.597360118129836,-0.588560296236878,-0.581547764742262,
-0.572737879990665,-0.562630022829078,-0.539120743771452,-0.527740193202501,
-0.522907197061913,-0.518716905154737,-0.511406980074506,-0.490157957161306,
-0.471257269792631,-0.4625702665497,-0.455555889274502,-0.446625224036467,
-0.436302467964124,-0.411315222304172,-0.401241893275841,-0.396650497196789,
-0.392325644017379,-0.384101172600747,-0.371673130043542,-0.344795779003007,
-0.336335971889365,-0.32931121992784,-0.320098782696567,-0.314408949318338,
-0.297552164027685,-0.278092449608793,-0.27244341390756,-0.268396189423533,
-0.262557550460827,-0.255221878535237,-0.236343058018277,-0.217665150549581,
-0.209627240224955,-0.20254426624099,-0.192592103284861,-0.180356641550837,
-0.158693095351688,-0.149324985386529,-0.144829869066863,-0.14042736650238,
-0.131688630949153,-0.117901398543954,-0.093898367928125,-0.0851856038670745,
-0.078170904286919,-0.0692664536942175,-0.0589912320322845,-0.0343493501421503,
-0.0243368999663489,-0.0195631100818421,-0.0157376569658423,-0.0113277168243253,
-0.000354962303461684),.UNSPECIFIED.);
#650=B_SPLINE_CURVE_WITH_KNOTS('',3,(#53776,#53777,#53778,#53779,#53780,
#53781,#53782,#53783,#53784,#53785,#53786,#53787,#53788,#53789,#53790,#53791,
#53792,#53793,#53794,#53795),.UNSPECIFIED.,.F.,.F.,(4,2,2,2,2,2,2,2,2,4),
(-1.48962364885331,-1.45799851151838,-1.44903501640883,-1.44202043222367,
-1.43336373572573,-1.41483556482368,-1.39335690597027,-1.38588751118161,
-1.38167498118498,-1.37994316952968),.UNSPECIFIED.);
#651=B_SPLINE_CURVE_WITH_KNOTS('',3,(#53797,#53798,#53799,#53800,#53801,
#53802,#53803,#53804,#53805,#53806,#53807,#53808,#53809,#53810,#53811,#53812,
#53813,#53814,#53815,#53816,#53817,#53818),.UNSPECIFIED.,.F.,.F.,(4,2,2,
2,2,2,2,2,2,2,4),(-0.109945337718666,-0.10005578303786,-0.0747324452225718,
-0.0649691927664568,-0.0604191866905936,-0.0560641058015071,-0.0476381350691081,
-0.0267483071399664,-0.00932637088096731,-0.00429109630289761,-0.000368170222445954),
 .UNSPECIFIED.);
#652=B_SPLINE_CURVE_WITH_KNOTS('',3,(#53819,#53820,#53821,#53822,#53823,
#53824,#53825,#53826,#53827,#53828,#53829,#53830,#53831,#53832,#53833,#53834,
#53835,#53836,#53837,#53838,#53839,#53840,#53841,#53842,#53843,#53844,#53845,
#53846,#53847,#53848,#53849,#53850,#53851,#53852,#53853,#53854,#53855,#53856,
#53857,#53858,#53859,#53860,#53861,#53862,#53863,#53864,#53865,#53866,#53867,
#53868,#53869,#53870,#53871,#53872,#53873,#53874,#53875,#53876,#53877,#53878,
#53879,#53880,#53881,#53882,#53883,#53884,#53885,#53886,#53887,#53888,#53889,
#53890,#53891,#53892,#53893,#53894,#53895,#53896,#53897,#53898,#53899,#53900,
#53901,#53902,#53903,#53904,#53905,#53906,#53907,#53908,#53909,#53910,#53911,
#53912,#53913,#53914,#53915,#53916,#53917,#53918,#53919,#53920,#53921,#53922,
#53923,#53924,#53925,#53926,#53927,#53928,#53929,#53930,#53931,#53932,#53933,
#53934,#53935,#53936,#53937,#53938,#53939,#53940,#53941,#53942),
 .UNSPECIFIED.,.F.,.F.,(4,2,2,2,2,2,2,2,2,2,2,2,2,2,2,2,2,2,2,2,2,2,2,2,
2,2,2,2,2,2,2,2,2,2,2,2,2,2,2,2,2,2,2,2,2,2,2,2,2,2,2,2,2,2,2,2,2,2,2,2,
2,4),(-1.60425228271969,-1.59886013992911,-1.59205050840229,-1.57668909305917,
-1.55163274571425,-1.54516388062916,-1.53981565161675,-1.53575173853546,
-1.52953672881361,-1.49971361789063,-1.48882279238098,-1.47957891257316,
-1.47255508515753,-1.46412392192429,-1.43695756392477,-1.42463775983764,
-1.41645729461622,-1.41214023795018,-1.4075422475674,-1.39740830220192,
-1.37252090057192,-1.3622183989205,-1.35329913441885,-1.34628765064055,
-1.33759730143691,-1.31863032565473,-1.29739385218365,-1.29010208755001,
-1.28591564218491,-1.28107972329177,-1.27063707299661,-1.24648612495446,
-1.23628861420684,-1.22742829918159,-1.22041800907575,-1.21167392727818,
-1.18819396703073,-1.17410960785412,-1.16526566989882,-1.16084904835453,
-1.15637469403923,-1.14714002177405,-1.12128598147573,-1.11085387246229,
-1.10186259577961,-1.09484992074297,-1.08622397677135,-1.0610803947368,
-1.04785444369528,-1.03932397932077,-1.03495446472101,-1.0304264937904,
-1.02115547325627,-0.999527691664109,-0.987315547425084,-0.977376206019699,
-0.97029781675934,-0.962260986410504,-0.943572063283242,-0.924684858362288,
-0.917347152536238,-0.911889189294514),.UNSPECIFIED.);
#653=B_SPLINE_CURVE_WITH_KNOTS('',3,(#53947,#53948,#53949,#53950,#53951,
#53952,#53953,#53954,#53955,#53956,#53957,#53958,#53959,#53960,#53961,#53962,
#53963,#53964,#53965,#53966,#53967,#53968,#53969,#53970,#53971,#53972,#53973,
#53974,#53975,#53976,#53977,#53978,#53979,#53980,#53981,#53982,#53983,#53984,
#53985,#53986,#53987,#53988,#53989,#53990,#53991,#53992,#53993,#53994,#53995,
#53996,#53997,#53998,#53999,#54000,#54001,#54002,#54003,#54004,#54005,#54006,
#54007,#54008,#54009,#54010,#54011,#54012,#54013,#54014,#54015,#54016,#54017,
#54018,#54019,#54020,#54021,#54022,#54023,#54024,#54025,#54026,#54027,#54028,
#54029,#54030,#54031,#54032,#54033,#54034,#54035,#54036,#54037,#54038,#54039,
#54040,#54041,#54042,#54043,#54044,#54045,#54046,#54047,#54048,#54049,#54050,
#54051,#54052,#54053,#54054,#54055,#54056,#54057,#54058,#54059,#54060,#54061,
#54062,#54063,#54064,#54065,#54066,#54067,#54068,#54069,#54070,#54071,#54072,
#54073,#54074,#54075,#54076,#54077,#54078,#54079,#54080,#54081,#54082,#54083,
#54084,#54085,#54086,#54087,#54088,#54089,#54090),.UNSPECIFIED.,.F.,.F.,
(4,2,2,2,2,2,2,2,2,2,2,2,2,2,2,2,2,2,2,2,2,2,2,2,2,2,2,2,2,2,2,2,2,2,2,
2,2,2,2,2,2,2,2,2,2,2,2,2,2,2,2,2,2,2,2,2,2,2,2,2,2,2,2,2,2,2,2,2,2,2,2,
4),(-1.49476463800755,-1.48836283425702,-1.47815618240204,-1.46928940850674,
-1.46227574437302,-1.45352914248273,-1.43002798940522,-1.41594785976451,
-1.40710406107762,-1.40268609286647,-1.39820862769885,-1.38896181796712,
-1.36311125633698,-1.35267711303315,-1.34368338708279,-1.33666748747283,
-1.32803561667801,-1.30291645266522,-1.2896715676271,-1.28113273027181,
-1.27676060817156,-1.27223100329919,-1.26295809711477,-1.24132188353044,
-1.22910655670356,-1.21916411766478,-1.21208258222925,-1.20404093868875,
-1.18522779054724,-1.16642677328903,-1.15910211910383,-1.15327044009174,
-1.14922358911303,-1.14356877698806,-1.12480200505867,-1.10141500565614,
-1.09228486896798,-1.08526435230261,-1.07674370509638,-1.05042155416237,
-1.03773291367076,-1.029406520026,-1.02506650580339,-1.02049633727313,-1.01058180054215,
-0.985458006045474,-0.975121199619371,-0.96618178387084,-0.959167407854628,
-0.950488622450764,-0.931694661572718,-0.910359596671632,-0.902996519478991,
-0.898798954452685,-0.893983371337442,-0.882678899523297,-0.85910920678493,
-0.848996118363765,-0.840182229711628,-0.833169552047423,-0.824373351557158,
-0.802189847399198,-0.781147227975423,-0.776102968175805,-0.772047802141666,
-0.766586745367916,-0.748623777043322,-0.722381009183814,-0.713858665508179,
-0.706906093943008,-0.69782471877296,-0.692748904775942),.UNSPECIFIED.);
#654=B_SPLINE_CURVE_WITH_KNOTS('',3,(#54091,#54092,#54093,#54094,#54095,
#54096,#54097,#54098,#54099,#54100,#54101,#54102,#54103,#54104,#54105,#54106,
#54107,#54108,#54109,#54110,#54111,#54112,#54113,#54114,#54115,#54116,#54117,
#54118,#54119,#54120,#54121,#54122,#54123,#54124,#54125,#54126,#54127,#54128,
#54129,#54130,#54131,#54132,#54133,#54134,#54135,#54136,#54137,#54138,#54139,
#54140,#54141,#54142,#54143,#54144,#54145,#54146,#54147,#54148,#54149,#54150,
#54151,#54152,#54153,#54154,#54155,#54156,#54157,#54158,#54159,#54160,#54161,
#54162,#54163,#54164,#54165,#54166,#54167,#54168,#54169,#54170,#54171,#54172,
#54173,#54174,#54175,#54176,#54177,#54178,#54179,#54180,#54181,#54182,#54183,
#54184,#54185,#54186,#54187,#54188,#54189,#54190,#54191,#54192,#54193,#54194,
#54195,#54196,#54197,#54198,#54199,#54200,#54201,#54202,#54203,#54204,#54205,
#54206,#54207,#54208,#54209,#54210,#54211,#54212,#54213,#54214,#54215,#54216,
#54217,#54218,#54219,#54220,#54221,#54222,#54223,#54224,#54225,#54226,#54227,
#54228,#54229,#54230,#54231,#54232),.UNSPECIFIED.,.F.,.F.,(4,2,2,2,2,2,
2,2,2,2,2,2,2,2,2,2,2,2,2,2,2,2,2,2,2,2,2,2,2,2,2,2,2,2,2,2,2,2,2,2,2,2,
2,2,2,2,2,2,2,2,2,2,2,2,2,2,2,2,2,2,2,2,2,2,2,2,2,2,2,2,4),(-0.911889189294514,
-0.911509021238188,-0.907463936454965,-0.901820872826992,-0.882103655125236,
-0.865432657612678,-0.859780367354239,-0.850607735719611,-0.843588278481432,
-0.835107194877428,-0.802257725779036,-0.789648542908412,-0.784638848655905,
-0.780511371089536,-0.77367121735012,-0.764396930434076,-0.737911044533359,
-0.726905439794408,-0.719774643262872,-0.712119822207256,-0.697483263531707,
-0.671707457677322,-0.662370562293857,-0.657880924998617,-0.653476747435654,
-0.644720012579152,-0.630880408782948,-0.60698447819079,-0.598267345681839,
-0.591255327990508,-0.582362763519045,-0.572107028998137,-0.547590577072453,
-0.537466800267108,-0.532676157949429,-0.528468360085987,-0.521031249194516,
-0.499609516124549,-0.481025527176616,-0.472364888537303,-0.465351039047699,
-0.456394174244022,-0.446023860311508,-0.420686670931562,-0.410942775532298,
-0.406395765569983,-0.402038832467301,-0.3935991511728,-0.380616214766329,
-0.354985428610164,-0.34640363022741,-0.340089024820618,-0.331461731902421,
-0.311556433860089,-0.287013662178649,-0.28176010244523,-0.277682212034723,
-0.271312588381915,-0.262979796614335,-0.236810207268542,-0.224616300761729,
-0.217259226853215,-0.209810514071386,-0.196906743140633,-0.17756139961699,
-0.162185110323441,-0.156490685368601,-0.15244452025261,-0.146655911311739,
-0.129475000774062,-0.109828012290715),.UNSPECIFIED.);
#655=B_SPLINE_CURVE_WITH_KNOTS('',3,(#54238,#54239,#54240,#54241,#54242,
#54243,#54244,#54245,#54246,#54247,#54248,#54249,#54250,#54251,#54252,#54253,
#54254,#54255,#54256,#54257,#54258,#54259,#54260,#54261,#54262,#54263,#54264,
#54265,#54266,#54267,#54268,#54269,#54270,#54271,#54272,#54273,#54274,#54275,
#54276,#54277,#54278,#54279,#54280,#54281,#54282,#54283,#54284,#54285,#54286,
#54287,#54288,#54289,#54290,#54291,#54292,#54293,#54294,#54295,#54296,#54297,
#54298,#54299,#54300,#54301,#54302,#54303,#54304,#54305,#54306,#54307,#54308,
#54309,#54310,#54311,#54312,#54313,#54314,#54315,#54316,#54317,#54318,#54319,
#54320,#54321,#54322,#54323,#54324,#54325,#54326,#54327,#54328,#54329,#54330,
#54331,#54332,#54333,#54334,#54335,#54336,#54337,#54338,#54339,#54340,#54341,
#54342,#54343,#54344,#54345,#54346,#54347,#54348,#54349,#54350,#54351,#54352,
#54353,#54354,#54355,#54356,#54357),.UNSPECIFIED.,.F.,.F.,(4,2,2,2,2,2,
2,2,2,2,2,2,2,2,2,2,2,2,2,2,2,2,2,2,2,2,2,2,2,2,2,2,2,2,2,2,2,2,2,2,2,2,
2,2,2,2,2,2,2,2,2,2,2,2,2,2,2,2,2,4),(-0.692980815119166,-0.685166320873275,
-0.680335305981931,-0.676143495922616,-0.668825199462455,-0.64756357223643,
-0.628679844563148,-0.619993388537569,-0.612978204666185,-0.604044878487092,
-0.593717982150457,-0.568706253487832,-0.558652593707495,-0.554063412592961,
-0.549736118811309,-0.541497731425997,-0.529035365321838,-0.502232072768898,
-0.493763353775518,-0.486738369859774,-0.477535834761316,-0.45764479787291,
-0.435017091219731,-0.429635808864119,-0.425580845449889,-0.419542627027357,
-0.411840026771538,-0.390626329152909,-0.374776344926731,-0.366816810972062,
-0.359713303272902,-0.349571500041958,-0.328261536242825,-0.309683941244289,
-0.304023235618637,-0.299975454537271,-0.294147216933534,-0.276605034792486,
-0.250865158023303,-0.242290923536331,-0.235338430058862,-0.226314935272215,
-0.215826701332353,-0.189606866256862,-0.180652720165412,-0.176217505888737,
-0.171755875055023,-0.162623290611988,-0.147709817722585,-0.12564556055034,
-0.116846925220763,-0.109831735811192,-0.101013975716215,-0.0908942254530899,
-0.067322851274371,-0.0559813973244607,-0.0511575166530446,-0.0469609964387052,
-0.0396151153015186,-0.000355547063539398),.UNSPECIFIED.);
#656=B_SPLINE_CURVE_WITH_KNOTS('',3,(#54358,#54359,#54360,#54361,#54362,
#54363,#54364,#54365,#54366,#54367,#54368,#54369,#54370,#54371,#54372,#54373,
#54374,#54375,#54376,#54377,#54378,#54379,#54380,#54381),.UNSPECIFIED.,
 .F.,.F.,(4,2,2,2,2,2,2,2,2,2,2,4),(-1.60439037716061,-1.59945122675283,
-1.59462474263139,-1.58821321942477,-1.57953987078498,-1.56057235854575,
-1.53930317729267,-1.53198957109054,-1.5277986145673,-1.52296607692686,
-1.51256007779002,-1.49476463800755),.UNSPECIFIED.);
#657=B_SPLINE_CURVE_WITH_KNOTS('',3,(#54383,#54384,#54385,#54386,#54387,
#54388,#54389,#54390,#54391,#54392,#54393,#54394,#54395,#54396,#54397,#54398,
#54399,#54400,#54401,#54402,#54403,#54404,#54405,#54406),.UNSPECIFIED.,
 .F.,.F.,(4,2,2,2,2,2,2,2,2,2,2,4),(-0.109828012290715,-0.103125880268508,
-0.0946120250454899,-0.0875913270661589,-0.078453506773865,-0.0550782175137834,
-0.0362647231901379,-0.0306079282228981,-0.0265611633896067,-0.0224960035305987,
-0.0162949183073028,-0.0003552119044235),.UNSPECIFIED.);
#658=B_SPLINE_CURVE_WITH_KNOTS('',3,(#54407,#54408,#54409,#54410,#54411,
#54412,#54413,#54414,#54415,#54416,#54417,#54418,#54419,#54420,#54421,#54422,
#54423,#54424,#54425,#54426,#54427,#54428,#54429,#54430,#54431,#54432,#54433,
#54434,#54435,#54436,#54437,#54438,#54439,#54440,#54441,#54442,#54443,#54444,
#54445,#54446,#54447,#54448,#54449,#54450,#54451,#54452,#54453,#54454,#54455,
#54456,#54457,#54458,#54459,#54460,#54461,#54462,#54463,#54464,#54465,#54466,
#54467,#54468,#54469,#54470,#54471,#54472,#54473,#54474,#54475,#54476,#54477,
#54478,#54479,#54480,#54481,#54482,#54483,#54484,#54485,#54486,#54487,#54488,
#54489,#54490,#54491,#54492,#54493,#54494,#54495,#54496,#54497,#54498,#54499,
#54500,#54501,#54502,#54503,#54504,#54505,#54506,#54507,#54508,#54509,#54510,
#54511,#54512,#54513,#54514,#54515,#54516,#54517,#54518,#54519,#54520,#54521,
#54522,#54523,#54524,#54525,#54526,#54527,#54528,#54529,#54530),
 .UNSPECIFIED.,.F.,.F.,(4,2,2,2,2,2,2,2,2,2,2,2,2,2,2,2,2,2,2,2,2,2,2,2,
2,2,2,2,2,2,2,2,2,2,2,2,2,2,2,2,2,2,2,2,2,2,2,2,2,2,2,2,2,2,2,2,2,2,2,2,
2,4),(-1.60450853446915,-1.58099180905865,-1.5741640089589,-1.56713939792466,
-1.55871752412026,-1.53174949229508,-1.51928866589299,-1.51105219965776,
-1.50672667142175,-1.50214046897003,-1.49209775827369,-1.46711358423613,
-1.45679739873521,-1.44787035341194,-1.44085844057041,-1.43217440865226,
-1.4132911845589,-1.39200871903329,-1.38468329509778,-1.38049199984088,
-1.37566688158213,-1.36530537971552,-1.34107119888107,-1.33086132124443,
-1.32199392559381,-1.31498323409782,-1.30624502641982,-1.28265190155576,
-1.2686288158881,-1.25980651665391,-1.25539298921942,-1.25091490543891,
-1.24165527928765,-1.21582764234192,-1.20539870632091,-1.19640907337983,
-1.18939619545903,-1.18076825971048,-1.15564300664585,-1.14240712476105,
-1.13387279165151,-1.12950258089611,-1.12497509223292,-1.11570809322809,
-1.09407805023255,-1.0818629800975,-1.07192199681267,-1.064843194393,-1.05680658619747,
-1.03815591414222,-1.01923797676905,-1.01189493822598,-1.0060538044972,
-1.00200849647931,-0.996367710829674,-0.976494308524129,-0.959911348274805,
-0.954275992030018,-0.945120733533117,-0.93810181209856,-0.929607066178783,
-0.912048462349294),.UNSPECIFIED.);
#659=B_SPLINE_CURVE_WITH_KNOTS('',3,(#54535,#54536,#54537,#54538,#54539,
#54540,#54541,#54542,#54543,#54544,#54545,#54546,#54547,#54548,#54549,#54550,
#54551,#54552,#54553,#54554,#54555,#54556,#54557,#54558,#54559,#54560,#54561,
#54562,#54563,#54564,#54565,#54566,#54567,#54568,#54569,#54570,#54571,#54572,
#54573,#54574,#54575,#54576,#54577,#54578,#54579,#54580,#54581,#54582,#54583,
#54584,#54585,#54586,#54587,#54588,#54589,#54590,#54591,#54592,#54593,#54594,
#54595,#54596,#54597,#54598,#54599,#54600,#54601,#54602,#54603,#54604,#54605,
#54606,#54607,#54608,#54609,#54610,#54611,#54612,#54613,#54614,#54615,#54616,
#54617,#54618,#54619,#54620,#54621,#54622,#54623,#54624,#54625,#54626,#54627,
#54628,#54629,#54630,#54631,#54632,#54633,#54634,#54635,#54636,#54637,#54638,
#54639,#54640,#54641,#54642,#54643,#54644,#54645,#54646,#54647,#54648,#54649,
#54650,#54651,#54652,#54653,#54654,#54655,#54656,#54657,#54658,#54659,#54660,
#54661,#54662,#54663,#54664,#54665,#54666,#54667,#54668,#54669,#54670,#54671,
#54672,#54673,#54674),.UNSPECIFIED.,.F.,.F.,(4,2,2,2,2,2,2,2,2,2,2,2,2,
2,2,2,2,2,2,2,2,2,2,2,2,2,2,2,2,2,2,2,2,2,2,2,2,2,2,2,2,2,2,2,2,2,2,2,2,
2,2,2,2,2,2,2,2,2,2,2,2,2,2,2,2,2,2,2,2,4),(-1.49497804194698,-1.49377195464921,
-1.48497036929973,-1.46340995305725,-1.44815265604888,-1.43890686622161,
-1.43443033816667,-1.43001345969881,-1.42117329002966,-1.39486737521192,
-1.3843759126987,-1.37535090415026,-1.36840089454909,-1.35983388144816,
-1.33401215177245,-1.31650686283038,-1.31068343962577,-1.30663722384223,
-1.30097604987968,-1.27613725998678,-1.26233461622457,-1.25162005754253,
-1.2444531036937,-1.23669429453869,-1.22108752706174,-1.1990978895747,-1.19128289441049,
-1.18518602246255,-1.18112926827002,-1.17579428831105,-1.14908934226767,
-1.13410421406953,-1.12453803673063,-1.11749152266626,-1.10926230799779,
-1.09293905901445,-1.07275516995505,-1.06520694413741,-1.0592535652122,
-1.05520400211965,-1.04976145591368,-1.02211595613978,-1.00876845741215,
-0.999004378077605,-0.991941117995587,-0.983817616971652,-0.953869524717951,
-0.937524458148364,-0.932408008225162,-0.928305601361065,-0.921687567099786,
-0.893160517076821,-0.882040654014953,-0.872672211123954,-0.865639450498399,
-0.857288980716925,-0.829358768559797,-0.811815809226221,-0.806655485712711,
-0.802561595530425,-0.796026524242121,-0.791496544735808,-0.776054627069269,
-0.754798161548612,-0.7459983635543,-0.738985060043492,-0.730173211738306,
-0.720062477091776,-0.696539000238583,-0.692980815119166),.UNSPECIFIED.);
#660=B_SPLINE_CURVE_WITH_KNOTS('',3,(#54675,#54676,#54677,#54678,#54679,
#54680,#54681,#54682,#54683,#54684,#54685,#54686,#54687,#54688,#54689,#54690,
#54691,#54692,#54693,#54694,#54695,#54696,#54697,#54698,#54699,#54700,#54701,
#54702,#54703,#54704,#54705,#54706,#54707,#54708,#54709,#54710,#54711,#54712,
#54713,#54714,#54715,#54716,#54717,#54718,#54719,#54720,#54721,#54722,#54723,
#54724,#54725,#54726,#54727,#54728,#54729,#54730,#54731,#54732,#54733,#54734,
#54735,#54736,#54737,#54738,#54739,#54740,#54741,#54742,#54743,#54744,#54745,
#54746,#54747,#54748,#54749,#54750,#54751,#54752,#54753,#54754,#54755,#54756,
#54757,#54758,#54759,#54760,#54761,#54762,#54763,#54764,#54765,#54766,#54767,
#54768,#54769,#54770,#54771,#54772,#54773,#54774,#54775,#54776,#54777,#54778,
#54779,#54780,#54781,#54782,#54783,#54784,#54785,#54786,#54787,#54788,#54789,
#54790,#54791,#54792,#54793,#54794,#54795,#54796,#54797,#54798,#54799,#54800,
#54801,#54802,#54803,#54804,#54805,#54806,#54807,#54808,#54809,#54810,#54811,
#54812,#54813,#54814,#54815,#54816,#54817,#54818,#54819,#54820,#54821,#54822),
 .UNSPECIFIED.,.F.,.F.,(4,2,2,2,2,2,2,2,2,2,2,2,2,2,2,2,2,2,2,2,2,2,2,2,
2,2,2,2,2,2,2,2,2,2,2,2,2,2,2,2,2,2,2,2,2,2,2,2,2,2,2,2,2,2,2,2,2,2,2,2,
2,2,2,2,2,2,2,2,2,2,2,2,2,4),(-0.912048462349294,-0.896787479541693,-0.887787252805348,
-0.881082056421924,-0.876970859194697,-0.87189978055317,-0.857601215483016,
-0.836619391417323,-0.826932624675712,-0.818361431293804,-0.811346248886324,
-0.802444281552055,-0.779149796069077,-0.759910889932576,-0.754261356548292,
-0.750215936334087,-0.744383568476121,-0.737058159169312,-0.718232648422221,
-0.699495194346949,-0.691459240057477,-0.684379613022506,-0.674435557334175,
-0.662213489616615,-0.640563554921123,-0.631282436702651,-0.626752510710786,
-0.622383498123253,-0.613859410053045,-0.600651412044106,-0.575508713103071,
-0.566885983404994,-0.559872175480125,-0.550874529020405,-0.54043000366026,
-0.514524808438672,-0.50530430098736,-0.500831460454452,-0.496411887490613,
-0.487552143587483,-0.473424108760431,-0.450057615849071,-0.44130968428607,
-0.434298088548766,-0.42543841115686,-0.415241315385748,-0.391130823378256,
-0.380611376633401,-0.375764561833978,-0.371581111540397,-0.364316991885263,
-0.343096210635845,-0.324106430740163,-0.315413171261473,-0.308400108134927,
-0.299479880692613,-0.289175185267792,-0.264315597332995,-0.254503511936039,
-0.249764492364517,-0.245530918965283,-0.237917195827653,-0.216255864773591,
-0.198101576875409,-0.189476678412823,-0.182461121057872,-0.173461239424339,
-0.163014121479963,-0.137102459672032,-0.127879756796657,-0.12340582189053,
-0.118985177997877,-0.110123264679583,-0.110052644177883),.UNSPECIFIED.);
#661=B_SPLINE_CURVE_WITH_KNOTS('',3,(#54828,#54829,#54830,#54831,#54832,
#54833,#54834,#54835,#54836,#54837,#54838,#54839,#54840,#54841,#54842,#54843,
#54844,#54845,#54846,#54847,#54848,#54849,#54850,#54851,#54852,#54853,#54854,
#54855,#54856,#54857,#54858,#54859,#54860,#54861,#54862,#54863,#54864,#54865,
#54866,#54867,#54868,#54869,#54870,#54871,#54872,#54873,#54874,#54875,#54876,
#54877,#54878,#54879,#54880,#54881,#54882,#54883,#54884,#54885,#54886,#54887,
#54888,#54889,#54890,#54891,#54892,#54893,#54894,#54895,#54896,#54897,#54898,
#54899,#54900,#54901,#54902,#54903,#54904,#54905,#54906,#54907,#54908,#54909,
#54910,#54911,#54912,#54913,#54914,#54915,#54916,#54917,#54918,#54919,#54920,
#54921,#54922,#54923,#54924,#54925,#54926,#54927,#54928,#54929,#54930,#54931,
#54932,#54933,#54934,#54935,#54936,#54937,#54938,#54939,#54940,#54941,#54942,
#54943,#54944,#54945,#54946,#54947,#54948,#54949),.UNSPECIFIED.,.F.,.F.,
(4,2,2,2,2,2,2,2,2,2,2,2,2,2,2,2,2,2,2,2,2,2,2,2,2,2,2,2,2,2,2,2,2,2,2,
2,2,2,2,2,2,2,2,2,2,2,2,2,2,2,2,2,2,2,2,2,2,2,2,2,4),(-0.692979258838884,
-0.67118995559551,-0.660866191665037,-0.651947318622327,-0.644970789635518,
-0.636378600644057,-0.60727614293275,-0.591512805470871,-0.586376026649255,
-0.582294060180516,-0.575795283599456,-0.553673671159206,-0.534265136420348,
-0.525531505302177,-0.518506056740535,-0.509590314510271,-0.499297170215878,
-0.474501837439696,-0.464694785347564,-0.459951122221414,-0.455704806824037,
-0.448031472572048,-0.425570280093862,-0.406534368994663,-0.398490632978779,
-0.391405509701558,-0.38145487535463,-0.369225695848239,-0.347565766891165,
-0.338273844980115,-0.333740773740727,-0.329373350516715,-0.32085914220195,
-0.307678112406119,-0.282468280722237,-0.273850874445708,-0.266838378502827,
-0.257839628417611,-0.24739307469677,-0.221482207085166,-0.212252537828199,
-0.207778796289508,-0.203359391533404,-0.194509561142105,-0.180413163659739,
-0.156976605719048,-0.14822795622256,-0.141211741118464,-0.132339867458766,
-0.122123580196769,-0.0978938520951423,-0.0874944227269537,-0.0826613397690077,
-0.0784679677917035,-0.071145027051044,-0.049875874748182,-0.0292982719334265,
-0.021178040717596,-0.0143023234670417,-0.00788979083151709,-0.000367801731532991),
 .UNSPECIFIED.);
#662=B_SPLINE_CURVE_WITH_KNOTS('',3,(#54950,#54951,#54952,#54953,#54954,
#54955,#54956,#54957,#54958,#54959,#54960,#54961,#54962,#54963,#54964,#54965,
#54966,#54967,#54968,#54969),.UNSPECIFIED.,.F.,.F.,(4,2,2,2,2,2,2,2,2,4),
(-1.60445172345304,-1.57087287035435,-1.56356495273178,-1.55937554915346,
-1.55454319912385,-1.54316751778459,-1.51968740073871,-1.5095887286719,
-1.50078343146496,-1.49497804194698),.UNSPECIFIED.);
#663=B_SPLINE_CURVE_WITH_KNOTS('',3,(#54971,#54972,#54973,#54974,#54975,
#54976,#54977,#54978,#54979,#54980,#54981,#54982,#54983,#54984,#54985,#54986,
#54987,#54988,#54989,#54990),.UNSPECIFIED.,.F.,.F.,(4,2,2,2,2,2,2,2,2,4),
(-0.110052644177883,-0.0959917623713727,-0.0726194674722937,-0.0638694112349162,
-0.0568561358282353,-0.0479943818297274,-0.037794935835177,-0.0146164749566909,
-0.00527669761352651,-0.000466613313815364),.UNSPECIFIED.);
#664=B_SPLINE_CURVE_WITH_KNOTS('',3,(#54991,#54992,#54993,#54994,#54995,
#54996,#54997,#54998,#54999,#55000,#55001,#55002,#55003,#55004,#55005,#55006,
#55007,#55008,#55009,#55010,#55011,#55012,#55013,#55014,#55015,#55016,#55017,
#55018,#55019,#55020,#55021,#55022,#55023,#55024,#55025,#55026,#55027,#55028,
#55029,#55030,#55031,#55032,#55033,#55034,#55035,#55036,#55037,#55038,#55039,
#55040,#55041,#55042,#55043,#55044,#55045,#55046,#55047,#55048,#55049,#55050,
#55051,#55052,#55053,#55054,#55055,#55056,#55057,#55058,#55059,#55060,#55061,
#55062,#55063,#55064,#55065,#55066,#55067,#55068,#55069,#55070,#55071,#55072,
#55073,#55074,#55075,#55076,#55077,#55078,#55079,#55080,#55081,#55082,#55083,
#55084,#55085,#55086,#55087,#55088,#55089,#55090,#55091,#55092,#55093,#55094,
#55095,#55096,#55097,#55098,#55099,#55100,#55101,#55102,#55103,#55104,#55105,
#55106,#55107,#55108,#55109,#55110,#55111,#55112),.UNSPECIFIED.,.F.,.F.,
(4,2,2,2,2,2,2,2,2,2,2,2,2,2,2,2,2,2,2,2,2,2,2,2,2,2,2,2,2,2,2,2,2,2,2,
2,2,2,2,2,2,2,2,2,2,2,2,2,2,2,2,2,2,2,2,2,2,2,2,2,4),(0.692945632510061,
0.701098988438348,0.725132570721244,0.745998105385564,0.751049440209536,
0.75510289302239,0.760547994319789,0.779389231545661,0.804529776262318,
0.813157989608204,0.820172689985033,0.829167560916291,0.839605347779739,
0.865502248436985,0.87469308324559,0.879162020220886,0.883586501275583,
0.892480291136297,0.906704758420185,0.929935863909063,0.938693251348128,
0.945703972588875,0.954551776009108,0.964726465256555,0.988716782702821,
0.999327278601534,1.00418418488939,1.008362128598,1.01559230609395,1.03687743233692,
1.05589371707847,1.06458793006142,1.07159922945832,1.08051378430896,1.09080779966496,
1.11563242884667,1.12544384119935,1.1301820351341,1.13441431598638,1.1420247916423,
1.16369368387706,1.18187472676576,1.19050111867402,1.19751519322408,1.20650973554747,
1.21694670810894,1.24282929574475,1.25204297954118,1.25651490592208,1.26093552223229,
1.26980250123599,1.28395001924971,1.307324402572,1.31607576538116,1.32308720435612,
1.33194298256497,1.35611708796313,1.37454359712428,1.38020969133085,1.38295740097097,
1.38531635665395),.UNSPECIFIED.);
#665=B_SPLINE_CURVE_WITH_KNOTS('',3,(#55116,#55117,#55118,#55119,#55120,
#55121,#55122,#55123,#55124,#55125,#55126,#55127,#55128,#55129,#55130,#55131,
#55132,#55133,#55134,#55135,#55136,#55137,#55138,#55139,#55140,#55141,#55142,
#55143,#55144,#55145,#55146,#55147,#55148,#55149,#55150,#55151,#55152,#55153,
#55154,#55155,#55156,#55157,#55158,#55159,#55160,#55161,#55162,#55163,#55164,
#55165,#55166,#55167,#55168,#55169,#55170,#55171,#55172,#55173),
 .UNSPECIFIED.,.F.,.F.,(4,3,3,3,3,3,3,3,3,3,3,3,3,3,3,3,3,3,3,4),(-4.04123713824997,
-3.94225244711282,-3.83273628999188,-3.72323042065973,-3.61400708733206,
-3.50484939767286,-3.39571794529748,-3.28596079280676,-3.17669944235086,
-3.06669438884274,-2.95668933533462,-2.84758449988576,-2.73866222057574,
-2.62984168483314,-2.52108273415307,-2.41234529469343,-2.30351145552693,
-2.19463277712453,-2.08555027678977,-1.98505081481724),.UNSPECIFIED.);
#666=B_SPLINE_CURVE_WITH_KNOTS('',3,(#55177,#55178,#55179,#55180,#55181),
 .UNSPECIFIED.,.F.,.F.,(4,1,4),(0.,0.985563111778209,1.08537753955771),
 .UNSPECIFIED.);
#667=B_SPLINE_CURVE_WITH_KNOTS('',3,(#55183,#55184,#55185,#55186,#55187,
#55188,#55189,#55190,#55191,#55192,#55193,#55194,#55195,#55196,#55197,#55198,
#55199,#55200,#55201,#55202,#55203,#55204,#55205,#55206,#55207,#55208,#55209,
#55210,#55211,#55212,#55213,#55214,#55215,#55216,#55217,#55218,#55219,#55220,
#55221,#55222,#55223,#55224,#55225,#55226,#55227,#55228,#55229,#55230,#55231,
#55232,#55233,#55234,#55235,#55236,#55237,#55238,#55239,#55240,#55241,#55242,
#55243,#55244,#55245,#55246,#55247,#55248,#55249,#55250,#55251,#55252,#55253,
#55254,#55255,#55256,#55257,#55258,#55259,#55260,#55261,#55262,#55263,#55264,
#55265,#55266,#55267,#55268,#55269,#55270,#55271,#55272,#55273,#55274,#55275,
#55276,#55277,#55278,#55279,#55280,#55281,#55282,#55283,#55284,#55285,#55286,
#55287,#55288,#55289,#55290,#55291,#55292,#55293,#55294,#55295,#55296,#55297,
#55298,#55299,#55300,#55301,#55302,#55303,#55304,#55305,#55306,#55307,#55308,
#55309,#55310,#55311,#55312,#55313,#55314,#55315,#55316,#55317,#55318,#55319,
#55320,#55321,#55322,#55323,#55324,#55325,#55326,#55327,#55328,#55329,#55330,
#55331,#55332,#55333,#55334,#55335,#55336,#55337,#55338,#55339,#55340,#55341,
#55342,#55343,#55344,#55345,#55346,#55347,#55348,#55349,#55350,#55351,#55352,
#55353,#55354,#55355,#55356,#55357),.UNSPECIFIED.,.F.,.F.,(4,3,3,3,3,3,
3,3,3,3,3,3,3,3,3,3,3,3,3,3,3,3,3,3,3,3,3,3,3,3,3,3,3,3,3,3,3,3,3,3,3,3,
3,3,3,3,3,3,3,3,3,3,3,3,3,3,3,3,4),(1.08537753955771,1.19609612505755,1.30308901533939,
1.40999021783501,1.51684224978507,1.62368754240906,1.73063567937683,1.83764628072714,
1.94483380370644,1.97112622355641,2.08051853033858,2.19003988096308,2.29913778678197,
2.40816980702691,2.51717555233518,2.62705399808504,2.73619094067904,2.84644013800683,
2.95668933533462,3.06618855596474,3.17569654235825,3.28491288691593,3.39406733753621,
3.50319929489951,3.61296258295283,3.72223356492953,3.83224300602117,3.94225244711282,
4.05148995552414,4.161030655945,4.26997382470323,4.37885158765571,4.48770382649441,
4.59773175959356,4.70671885335743,4.81726720612423,4.92781555889103,5.03716800382292,
5.14669433717871,5.25575579897979,5.3647527746709,5.47372494165427,5.58363837390801,
5.69274576144384,5.80306221605654,5.91337867066923,6.02273158896768,6.13225786315265,
6.24132068816919,6.3503193589255,6.45929355088761,6.56920560877757,6.67831581327472,
6.78862879786108,6.89894178244744,7.01634704840949,7.13200788731664,7.25028536680614,
7.36856284629564),.UNSPECIFIED.);
#668=B_SPLINE_CURVE_WITH_KNOTS('',3,(#55359,#55360,#55361,#55362,#55363,
#55364,#55365,#55366,#55367,#55368,#55369,#55370,#55371,#55372,#55373,#55374,
#55375,#55376,#55377,#55378,#55379,#55380,#55381,#55382,#55383,#55384,#55385,
#55386,#55387,#55388,#55389,#55390,#55391,#55392,#55393,#55394,#55395,#55396,
#55397,#55398,#55399,#55400,#55401,#55402,#55403,#55404,#55405,#55406,#55407,
#55408,#55409,#55410,#55411,#55412,#55413,#55414,#55415,#55416,#55417,#55418,
#55419,#55420,#55421,#55422,#55423,#55424,#55425,#55426,#55427,#55428,#55429,
#55430,#55431,#55432,#55433,#55434,#55435,#55436,#55437,#55438,#55439,#55440,
#55441,#55442,#55443,#55444,#55445,#55446,#55447,#55448,#55449,#55450,#55451,
#55452,#55453,#55454,#55455,#55456,#55457,#55458,#55459,#55460,#55461,#55462,
#55463,#55464,#55465,#55466,#55467,#55468,#55469,#55470,#55471,#55472,#55473,
#55474,#55475,#55476,#55477,#55478,#55479,#55480,#55481,#55482,#55483,#55484,
#55485,#55486,#55487,#55488,#55489,#55490,#55491,#55492,#55493,#55494,#55495,
#55496,#55497,#55498,#55499,#55500,#55501,#55502,#55503,#55504,#55505,#55506,
#55507,#55508,#55509,#55510,#55511,#55512,#55513,#55514,#55515,#55516,#55517,
#55518,#55519,#55520,#55521,#55522,#55523,#55524,#55525,#55526,#55527,#55528,
#55529,#55530,#55531,#55532,#55533),.UNSPECIFIED.,.F.,.F.,(4,3,3,3,3,3,
3,3,3,3,3,3,3,3,3,3,3,3,3,3,3,3,3,3,3,3,3,3,3,3,3,3,3,3,3,3,3,3,3,3,3,3,
3,3,3,3,3,3,3,3,3,3,3,3,3,3,3,3,4),(7.3685628467373,7.48153885872925,7.59477484966834,
7.7081490758396,7.82180510018963,7.88450489422564,7.9938449101036,8.10337279709113,
8.21242191116621,8.3214066065219,8.43036658246054,8.54029193834637,8.6493874997913,
8.75972775289758,8.87006800600385,8.97940661138203,9.08893467468203,9.19798242504892,
9.30696577840231,9.41592443647842,9.52585110680433,9.63494542566003,9.74528827172105,
9.85563111778206,9.96496690329824,10.074495319081,10.183540107565,10.2925204542086,
10.4014760658998,10.5114056068149,10.6204968171082,10.7308455233342,10.8411942295603,
10.9505318783152,11.0600600611931,11.1691067785061,11.2780890730194,11.387046648252,
11.4969743215237,11.6060675109473,11.7164124261429,11.8267573413385,11.9360946581711,
12.0456228825393,12.1546692664882,12.2636512280816,12.3726084714257,12.4825364668485,
12.5916293308537,12.7019748919852,12.8123204531167,12.9200463210862,13.0276280771467,
13.1351078843213,13.2425277495154,13.3499863415123,13.4574600064483,13.5650841670389,
13.6517481535604),.UNSPECIFIED.);
#669=B_SPLINE_CURVE_WITH_KNOTS('',3,(#55535,#55536,#55537,#55538,#55539,
#55540,#55541,#55542,#55543,#55544,#55545,#55546,#55547,#55548,#55549,#55550,
#55551,#55552,#55553,#55554,#55555,#55556,#55557,#55558,#55559,#55560,#55561,
#55562,#55563,#55564,#55565,#55566,#55567,#55568,#55569,#55570,#55571,#55572,
#55573,#55574,#55575,#55576,#55577,#55578,#55579,#55580,#55581,#55582,#55583,
#55584,#55585,#55586,#55587,#55588,#55589,#55590,#55591,#55592,#55593,#55594,
#55595,#55596,#55597,#55598,#55599,#55600,#55601,#55602,#55603,#55604,#55605,
#55606,#55607,#55608,#55609,#55610,#55611,#55612,#55613,#55614,#55615,#55616,
#55617,#55618,#55619,#55620,#55621,#55622,#55623,#55624,#55625,#55626,#55627,
#55628,#55629,#55630,#55631,#55632,#55633,#55634,#55635,#55636,#55637,#55638,
#55639,#55640,#55641,#55642,#55643,#55644,#55645,#55646,#55647,#55648,#55649,
#55650,#55651,#55652,#55653,#55654,#55655,#55656,#55657,#55658,#55659,#55660,
#55661,#55662,#55663,#55664,#55665,#55666,#55667,#55668,#55669,#55670,#55671,
#55672,#55673,#55674,#55675,#55676,#55677,#55678,#55679,#55680,#55681,#55682,
#55683,#55684,#55685,#55686,#55687,#55688,#55689,#55690,#55691,#55692,#55693,
#55694,#55695,#55696,#55697,#55698,#55699,#55700,#55701,#55702,#55703,#55704,
#55705,#55706),.UNSPECIFIED.,.F.,.F.,(4,3,3,3,3,3,3,3,3,3,3,3,3,3,3,3,3,
3,3,3,3,3,3,3,3,3,3,3,3,3,3,3,3,3,3,3,3,3,3,3,3,3,3,3,3,3,3,3,3,3,3,3,3,
3,3,3,3,4),(13.6517481539169,13.7978835648949,13.9072208386646,14.0167490684156,
14.1257954027862,14.2347773124886,14.3437345017137,14.4536625454536,14.5627553504665,
14.6731010135698,14.7834466766731,14.8927838932927,15.0023121301875,15.1113584064312,
15.2203402578103,15.3292973886179,15.4392254885762,15.5483182356278,15.6586640120395,
15.7690097884513,15.8783469822886,15.9878752220312,16.0969214740007,16.2059033006146,
16.3148604062078,16.4247885297132,16.5338812507372,16.6442270754833,16.7545729002295,
16.8639101200874,16.9734383565774,17.0824846356086,17.1914664895968,17.3004236228299,
17.4103517201243,17.5194444691187,17.6297902405632,17.7401360120077,17.8494732232515,
17.9590014608183,18.06804773103,18.1770295761472,18.2859867004733,18.3959148063015,
18.5050075464051,18.6153533350955,18.7256991237859,18.8350363334543,18.944564571218,
19.0536108397158,19.1625926830721,19.271549805593,19.3814779130857,19.4905706512962,
19.6009164434301,19.7112622355641,19.8572147419281,19.9349334610965),
 .UNSPECIFIED.);
#670=B_SPLINE_CURVE_WITH_KNOTS('',3,(#55708,#55709,#55710,#55711,#55712,
#55713,#55714,#55715,#55716,#55717,#55718,#55719,#55720,#55721,#55722,#55723,
#55724,#55725,#55726,#55727,#55728,#55729,#55730,#55731,#55732,#55733,#55734,
#55735,#55736,#55737,#55738,#55739,#55740,#55741,#55742,#55743,#55744,#55745,
#55746,#55747,#55748,#55749,#55750,#55751,#55752,#55753,#55754,#55755,#55756,
#55757,#55758,#55759,#55760,#55761,#55762,#55763,#55764,#55765,#55766,#55767,
#55768,#55769,#55770,#55771,#55772,#55773,#55774,#55775,#55776,#55777,#55778,
#55779,#55780,#55781,#55782,#55783,#55784,#55785,#55786,#55787,#55788,#55789,
#55790,#55791,#55792,#55793,#55794,#55795,#55796,#55797,#55798,#55799,#55800,
#55801,#55802,#55803,#55804,#55805,#55806,#55807,#55808,#55809,#55810,#55811,
#55812,#55813,#55814,#55815,#55816,#55817,#55818,#55819,#55820,#55821,#55822,
#55823,#55824,#55825,#55826,#55827,#55828,#55829,#55830,#55831,#55832,#55833,
#55834,#55835,#55836,#55837,#55838,#55839,#55840,#55841,#55842,#55843,#55844,
#55845,#55846,#55847,#55848,#55849,#55850,#55851,#55852,#55853,#55854,#55855,
#55856,#55857,#55858,#55859,#55860,#55861,#55862,#55863,#55864,#55865,#55866,
#55867,#55868,#55869,#55870,#55871,#55872,#55873,#55874,#55875,#55876,#55877,
#55878,#55879,#55880,#55881,#55882),.UNSPECIFIED.,.F.,.F.,(4,3,3,3,3,3,
3,3,3,3,3,3,3,3,3,3,3,3,3,3,3,3,3,3,3,3,3,3,3,3,3,3,3,3,3,3,3,3,3,3,3,3,
3,3,3,3,3,3,3,3,3,3,3,3,3,3,3,3,4),(19.9349334614217,20.0426247475374,20.15023541793,
20.2578072367367,20.3675617643881,20.4752466720914,20.5860360097169,20.6968253473423,
20.8061625587225,20.9156907962723,21.0247370665719,21.1337189117587,21.2426760361357,
21.3526041418819,21.4616968819895,21.572042670555,21.6823884591205,21.7917256704712,
21.9012539080246,22.0103001782835,22.1192820234254,22.2282391477534,22.3381672535397,
22.4472599935889,22.5576057822438,22.6679515708987,22.7772887825285,22.886817020047,
22.9958632905997,23.10484513604,23.2138022606707,23.3237303661722,23.4328231065306,
23.5431688946038,23.6535146826769,23.7628518941414,23.8723801316806,23.9814264020619,
24.0904082473291,24.1993653717851,24.3092934774526,24.4183862176348,24.5287320060449,
24.6390777944551,24.7484150060951,24.8579432436124,24.9669895141692,25.0759713596114,
25.1849284842416,25.2948565897395,25.4039493300921,25.5142951181627,25.6246409062333,
25.7354821569353,25.8461429057937,25.9566374510624,26.0670349562016,26.1773739290343,
26.2181187682761),.UNSPECIFIED.);
#671=B_SPLINE_CURVE_WITH_KNOTS('',3,(#55884,#55885,#55886,#55887,#55888,
#55889,#55890,#55891,#55892,#55893,#55894,#55895,#55896,#55897,#55898,#55899,
#55900,#55901,#55902,#55903,#55904,#55905,#55906,#55907,#55908,#55909,#55910,
#55911,#55912,#55913,#55914,#55915,#55916,#55917,#55918,#55919,#55920,#55921,
#55922,#55923,#55924,#55925,#55926,#55927,#55928,#55929,#55930,#55931,#55932,
#55933,#55934,#55935,#55936,#55937,#55938,#55939,#55940,#55941,#55942,#55943,
#55944,#55945,#55946,#55947,#55948,#55949,#55950,#55951,#55952,#55953,#55954,
#55955,#55956,#55957,#55958,#55959,#55960,#55961,#55962,#55963,#55964,#55965,
#55966,#55967,#55968,#55969,#55970,#55971,#55972,#55973,#55974,#55975,#55976,
#55977,#55978,#55979,#55980,#55981,#55982,#55983,#55984,#55985,#55986,#55987,
#55988,#55989,#55990,#55991,#55992,#55993,#55994,#55995,#55996,#55997,#55998,
#55999,#56000,#56001,#56002,#56003,#56004,#56005,#56006,#56007,#56008,#56009,
#56010,#56011,#56012,#56013,#56014,#56015,#56016,#56017,#56018,#56019,#56020,
#56021,#56022,#56023,#56024,#56025,#56026,#56027,#56028,#56029,#56030,#56031,
#56032,#56033,#56034,#56035,#56036,#56037,#56038,#56039,#56040,#56041,#56042,
#56043,#56044,#56045,#56046,#56047,#56048,#56049,#56050,#56051,#56052,#56053,
#56054,#56055,#56056,#56057,#56058),.UNSPECIFIED.,.F.,.F.,(4,3,3,3,3,3,
3,3,3,3,3,3,3,3,3,3,3,3,3,3,3,3,3,3,3,3,3,3,3,3,3,3,3,3,3,3,3,3,3,3,3,3,
3,3,3,3,3,3,3,3,3,3,3,3,3,3,3,3,4),(26.2181187686548,26.3384959137195,26.4593174082803,
26.5806968286956,26.6102040180115,26.7195412294059,26.8290694669539,26.9381157372594,
27.047097582449,27.1560547068255,27.2659828125666,27.3750755526661,27.4854213412279,
27.5957671297898,27.7051043424275,27.81463257982,27.9236788513792,28.0326606978225,
28.141617823451,28.2515459279802,28.3606386693125,28.4709844554403,28.581330241568,
28.6906674510535,28.8001956888401,28.9092419572624,29.0182238005836,29.1271809231098,
29.2371090306689,29.3462017689833,29.4565475611647,29.5668933533462,29.676230564775,
29.7857588023187,29.8948050726067,30.0037869177593,30.1127440420799,30.222672147841,
30.3317648878394,30.4421106764819,30.5524564651244,30.6617936853272,30.7713219217741,
30.8803682009476,30.9893500550019,31.0983071882249,31.2082352853943,31.3173280341927,
31.4276738055476,31.5380195769026,31.6469506371475,31.7556960802581,31.8643381430127,
31.9729172904604,32.0814739006531,32.1901241097691,32.2988188835178,32.4077120677762,
32.5013040751382),.UNSPECIFIED.);
#672=B_SPLINE_CURVE_WITH_KNOTS('',3,(#56060,#56061,#56062,#56063,#56064,
#56065,#56066,#56067,#56068,#56069,#56070,#56071,#56072,#56073,#56074,#56075,
#56076,#56077,#56078,#56079,#56080,#56081,#56082,#56083,#56084,#56085,#56086,
#56087,#56088,#56089,#56090,#56091,#56092,#56093,#56094,#56095,#56096,#56097,
#56098,#56099,#56100,#56101,#56102,#56103,#56104,#56105,#56106,#56107,#56108,
#56109,#56110,#56111,#56112,#56113,#56114,#56115,#56116,#56117,#56118,#56119,
#56120,#56121,#56122,#56123,#56124,#56125,#56126,#56127,#56128,#56129,#56130,
#56131,#56132,#56133,#56134,#56135,#56136,#56137,#56138,#56139,#56140,#56141,
#56142,#56143,#56144,#56145,#56146,#56147,#56148,#56149,#56150,#56151,#56152,
#56153,#56154,#56155,#56156,#56157,#56158,#56159,#56160,#56161,#56162,#56163,
#56164,#56165,#56166,#56167,#56168,#56169,#56170,#56171,#56172,#56173,#56174,
#56175,#56176,#56177,#56178,#56179,#56180,#56181,#56182,#56183,#56184,#56185,
#56186,#56187,#56188,#56189,#56190,#56191,#56192,#56193,#56194,#56195,#56196,
#56197,#56198,#56199,#56200,#56201,#56202,#56203,#56204,#56205,#56206,#56207,
#56208,#56209,#56210,#56211,#56212,#56213,#56214,#56215,#56216,#56217,#56218,
#56219,#56220,#56221,#56222,#56223,#56224,#56225,#56226,#56227,#56228,#56229,
#56230,#56231,#56232,#56233,#56234),.UNSPECIFIED.,.F.,.F.,(4,3,3,3,3,3,
3,3,3,3,3,3,3,3,3,3,3,3,3,3,3,3,3,3,3,3,3,3,3,3,3,3,3,3,3,3,3,3,3,3,3,3,
3,3,3,3,3,3,3,3,3,3,3,3,3,3,3,3,4),(32.5013040754556,32.5235826886808,32.6329199073593,
32.7424481439968,32.8514944210897,32.9604762728626,33.0694334036092,33.1793615028216,
33.2884542487017,33.3988000245803,33.509145800459,33.6184830760487,33.7280113055722,
33.8370576406939,33.9460395507448,34.0549967399167,34.1649247829968,34.274017586975,
34.3843632496061,34.4947089122372,34.6040459492957,34.7135742086356,34.8226203053257,
34.9316019776638,35.0405589302422,35.1504872036855,35.2595797765364,35.3699259002759,
35.4802720240154,35.5896093619076,35.6991375836433,35.8081839762799,35.9171659419024,
36.0261231846247,36.136051172417,36.2451440244415,36.3554895801176,36.4658351357936,
36.5751727899969,36.6847009721938,36.7937476917544,36.9027299873101,37.0116875623818,
37.1216152336793,37.2307084200033,37.3410533337875,37.4513982475718,37.5607339329457,
37.6702623612463,37.779307108419,37.8882874359025,37.9972430505506,38.1071726277504,
38.216263895013,38.3266126271815,38.43696135935,38.5625537048142,38.6871198019977,
38.7844893822274),.UNSPECIFIED.);
#673=B_SPLINE_CURVE_WITH_KNOTS('',3,(#56236,#56237,#56238,#56239,#56240,
#56241,#56242,#56243,#56244,#56245,#56246,#56247,#56248,#56249,#56250,#56251,
#56252,#56253,#56254,#56255,#56256,#56257,#56258,#56259,#56260,#56261,#56262,
#56263,#56264,#56265,#56266,#56267,#56268,#56269,#56270,#56271,#56272,#56273,
#56274,#56275,#56276,#56277,#56278,#56279,#56280,#56281,#56282,#56283,#56284,
#56285,#56286,#56287,#56288,#56289,#56290,#56291,#56292,#56293,#56294,#56295,
#56296,#56297,#56298,#56299,#56300,#56301,#56302,#56303,#56304,#56305,#56306,
#56307,#56308,#56309,#56310,#56311,#56312,#56313,#56314,#56315,#56316,#56317,
#56318,#56319,#56320,#56321,#56322,#56323,#56324,#56325,#56326,#56327,#56328,
#56329,#56330,#56331,#56332,#56333,#56334,#56335,#56336,#56337,#56338,#56339,
#56340,#56341,#56342,#56343,#56344,#56345,#56346,#56347,#56348,#56349,#56350,
#56351,#56352,#56353,#56354,#56355,#56356,#56357,#56358,#56359,#56360,#56361,
#56362,#56363,#56364,#56365,#56366,#56367,#56368,#56369,#56370,#56371,#56372,
#56373,#56374,#56375,#56376,#56377,#56378,#56379,#56380,#56381,#56382,#56383,
#56384,#56385,#56386,#56387,#56388,#56389,#56390,#56391,#56392,#56393,#56394,
#56395,#56396,#56397,#56398,#56399,#56400,#56401,#56402,#56403,#56404,#56405,
#56406,#56407,#56408,#56409,#56410),.UNSPECIFIED.,.F.,.F.,(4,3,3,3,3,3,
3,3,3,3,3,3,3,3,3,3,3,3,3,3,3,3,3,3,3,3,3,3,3,3,3,3,3,3,3,3,3,3,3,3,3,3,
3,3,3,3,3,3,3,3,3,3,3,3,3,3,3,3,4),(38.7844893826353,38.8937562439304,39.0030205291665,
39.1124040424951,39.2218467620058,39.3315047765829,39.4225244711282,39.531864446128,
39.6413923382253,39.7504414354374,39.8594261229724,39.9683861001188,40.0783114708157,
40.1874070555165,40.2977473192114,40.4080875829064,40.5174118990146,40.6269417484733,
40.7359751200007,40.8449441019264,40.9538884202333,41.0638289888461,41.1729092104048,
41.2832799525447,41.3936506946846,41.5030054920437,41.6125315313461,41.7215951314652,
41.8305941616126,41.9395682978918,42.0494796750345,42.1585888103856,42.2689013084242,
42.3792138064628,42.4885651699356,42.5980916384737,42.707152654175,42.816149423017,
42.9251216220356,43.035035446087,43.1441434489396,43.2544601835903,43.364776918241,
43.4740090834525,43.5835504517734,43.6924914154099,43.8013681540031,43.9102205474251,
44.0202504180736,44.1292405486958,44.2397902893575,44.3503400300192,44.4588741857476,
44.5672556291874,44.6755255492681,44.7837478551205,44.891939875013,45.0001948129805,
45.0676746898148),.UNSPECIFIED.);
#674=B_SPLINE_CURVE_WITH_KNOTS('',3,(#56412,#56413,#56414,#56415,#56416,
#56417,#56418,#56419,#56420,#56421,#56422,#56423,#56424,#56425,#56426,#56427,
#56428,#56429,#56430,#56431,#56432,#56433,#56434,#56435,#56436,#56437,#56438,
#56439,#56440,#56441,#56442,#56443,#56444,#56445),.UNSPECIFIED.,.F.,.F.,
(4,3,3,3,3,3,3,3,3,3,3,4),(45.0676746902223,45.203625675157,45.3359031417975,
45.4450078827114,45.5539300697693,45.6627505143036,45.7715093749702,45.8802467257635,
45.9890804881181,46.0979590906992,46.2070415430544,46.3075704370366),
 .UNSPECIFIED.);
#675=B_SPLINE_CURVE_WITH_KNOTS('',3,(#56449,#56450,#56451,#56452,#56453,
#56454,#56455),.UNSPECIFIED.,.F.,.F.,(4,3,4),(-48.2925924771321,-48.1551961866216,
-48.0235345953958),.UNSPECIFIED.);
#676=B_SPLINE_CURVE_WITH_KNOTS('',3,(#56457,#56458,#56459,#56460,#56461,
#56462,#56463,#56464,#56465,#56466),.UNSPECIFIED.,.F.,.F.,(4,1,1,1,1,1,
1,4),(-48.0235342885071,-47.3070293653539,-46.3214662535757,-45.3359031417975,
-44.3503400300192,-43.364776918241,-42.3792138064628,-41.7403489813275),
 .UNSPECIFIED.);
#677=B_SPLINE_CURVE_WITH_KNOTS('',3,(#56468,#56469,#56470,#56471,#56472,
#56473,#56474,#56475,#56476,#56477,#56478,#56479,#56480,#56481,#56482,#56483,
#56484,#56485,#56486,#56487,#56488,#56489,#56490,#56491,#56492,#56493,#56494,
#56495,#56496,#56497,#56498,#56499,#56500,#56501,#56502,#56503,#56504,#56505,
#56506,#56507,#56508,#56509,#56510,#56511,#56512,#56513,#56514,#56515,#56516,
#56517,#56518,#56519,#56520,#56521,#56522,#56523,#56524,#56525,#56526,#56527,
#56528,#56529,#56530,#56531,#56532,#56533,#56534,#56535,#56536,#56537,#56538,
#56539,#56540,#56541,#56542,#56543,#56544,#56545,#56546,#56547,#56548,#56549,
#56550,#56551,#56552,#56553,#56554,#56555,#56556,#56557,#56558,#56559,#56560,
#56561,#56562,#56563,#56564,#56565,#56566,#56567,#56568,#56569,#56570,#56571,
#56572,#56573,#56574,#56575,#56576,#56577,#56578,#56579,#56580,#56581,#56582,
#56583,#56584,#56585,#56586,#56587,#56588,#56589,#56590,#56591,#56592,#56593,
#56594,#56595,#56596,#56597,#56598,#56599,#56600,#56601,#56602,#56603,#56604,
#56605,#56606,#56607,#56608,#56609,#56610,#56611,#56612,#56613,#56614,#56615,
#56616,#56617,#56618,#56619,#56620,#56621,#56622,#56623,#56624,#56625,#56626,
#56627,#56628,#56629,#56630,#56631,#56632,#56633,#56634,#56635,#56636,#56637,
#56638,#56639,#56640,#56641,#56642),.UNSPECIFIED.,.F.,.F.,(4,3,3,3,3,3,
3,3,3,3,3,3,3,3,3,3,3,3,3,3,3,3,3,3,3,3,3,3,3,3,3,3,3,3,3,3,3,3,3,3,3,3,
3,3,3,3,3,3,3,3,3,3,3,3,3,3,3,3,4),(-41.7403485560519,-41.615840513558,
-41.4902535416044,-41.3936506946846,-41.284325628528,-41.1747958728253,
-41.0657621949742,-40.9567930737688,-40.8478487829612,-40.7379084829475,
-40.628828696172,-40.5184581395392,-40.4080875829064,-40.2987475649647,
-40.1892196782351,-40.0801705620444,-39.9711858645597,-39.8622258864825,
-39.7523005326439,-39.6432049690615,-39.5328647200948,-39.4225244711282,
-39.3131858654622,-39.2036578021981,-39.0946100515161,-38.9856266978384,
-38.8766680394291,-38.7667413694093,-38.6576470502025,-38.5473042047762,
-38.43696135935,-38.3276255745887,-38.2180971587116,-38.1090523710127,-38.0000720251634,
-37.8911164142742,-37.7811868725986,-37.6720956631173,-37.5617469553446,
-37.4513982475718,-37.3420605984726,-37.2325324156377,-37.1234856979709,
-37.0145034031013,-36.9055458275105,-36.7956181545813,-36.6865249647992,
-36.5761800502964,-36.4658351357936,-36.3564978189441,-36.246969594578,
-36.1379232106088,-36.0289412489942,-35.9199840056274,-35.8100560102244,
-35.700963146194,-35.5906175851047,-35.4802720240154,-35.4571636741479),
 .UNSPECIFIED.);
#678=B_SPLINE_CURVE_WITH_KNOTS('',3,(#56644,#56645,#56646,#56647,#56648,
#56649,#56650,#56651,#56652,#56653,#56654,#56655,#56656,#56657,#56658,#56659,
#56660,#56661,#56662,#56663,#56664,#56665,#56666,#56667,#56668,#56669,#56670,
#56671,#56672,#56673,#56674,#56675,#56676,#56677,#56678,#56679,#56680,#56681,
#56682,#56683,#56684,#56685,#56686,#56687,#56688,#56689,#56690,#56691,#56692,
#56693,#56694,#56695,#56696,#56697,#56698,#56699,#56700,#56701,#56702,#56703,
#56704,#56705,#56706,#56707,#56708,#56709,#56710,#56711,#56712,#56713,#56714,
#56715,#56716,#56717,#56718,#56719,#56720,#56721,#56722,#56723,#56724,#56725,
#56726,#56727,#56728,#56729,#56730,#56731,#56732,#56733,#56734,#56735,#56736,
#56737,#56738,#56739,#56740,#56741,#56742,#56743,#56744,#56745,#56746,#56747,
#56748,#56749,#56750,#56751,#56752,#56753,#56754,#56755,#56756,#56757,#56758,
#56759,#56760,#56761,#56762,#56763,#56764,#56765,#56766,#56767,#56768,#56769,
#56770,#56771,#56772,#56773,#56774,#56775,#56776,#56777,#56778,#56779,#56780,
#56781,#56782,#56783,#56784,#56785,#56786,#56787,#56788,#56789,#56790,#56791,
#56792,#56793,#56794,#56795,#56796,#56797,#56798,#56799,#56800,#56801,#56802,
#56803,#56804,#56805,#56806,#56807,#56808,#56809,#56810,#56811,#56812,#56813,
#56814,#56815,#56816,#56817,#56818),.UNSPECIFIED.,.F.,.F.,(4,3,3,3,3,3,
3,3,3,3,3,3,3,3,3,3,3,3,3,3,3,3,3,3,3,3,3,3,3,3,3,3,3,3,3,3,3,3,3,3,3,3,
3,3,3,3,3,3,3,3,3,3,3,3,3,3,3,3,4),(-35.4571636738398,-35.3482509468301,
-35.2395222303795,-35.1308958950177,-35.0223314563655,-34.9137885159107,
-34.8051505167586,-34.696467014166,-34.5875841193446,-34.4947089122372,
-34.3853716384126,-34.2758434086684,-34.1667970742412,-34.0578151644816,
-33.948857975199,-33.838929931514,-33.7298371264434,-33.6194914634512,-33.509145800459,
-33.3998085838417,-33.2902803469466,-33.1812340707049,-33.0722522193277,
-32.9632950885218,-32.8533669885615,-32.7442742415114,-32.6339284650961,
-32.5235826886808,-32.4142454948571,-32.3047172551128,-32.1956710031575,
-32.0866891765581,-31.9777320709795,-31.8678039474603,-31.7587112264511,
-31.6483654016769,-31.5380195769026,-31.4286823570365,-31.3191541205475,
-31.2101078415077,-31.1011259875108,-30.9921688542689,-30.8822407569828,
-30.7731480079796,-30.662802236552,-30.5524564651244,-30.4431192538816,
-30.3335910163147,-30.2245447461042,-30.1155629009879,-30.0066057766627,
-29.8966776708336,-29.7875849307311,-29.6772391420386,-29.5668933533462,
-29.4456706023087,-29.3248472979377,-29.2046599751121,-29.1739783673454),
 .UNSPECIFIED.);
#679=B_SPLINE_CURVE_WITH_KNOTS('',3,(#56820,#56821,#56822,#56823,#56824,
#56825,#56826,#56827,#56828,#56829,#56830,#56831,#56832,#56833,#56834,#56835,
#56836,#56837,#56838,#56839,#56840,#56841,#56842,#56843,#56844,#56845,#56846,
#56847,#56848,#56849,#56850,#56851,#56852,#56853,#56854,#56855,#56856,#56857,
#56858,#56859,#56860,#56861,#56862,#56863,#56864,#56865,#56866,#56867,#56868,
#56869,#56870,#56871,#56872,#56873,#56874,#56875,#56876,#56877,#56878,#56879,
#56880,#56881,#56882,#56883,#56884,#56885,#56886,#56887,#56888,#56889,#56890,
#56891,#56892,#56893,#56894,#56895,#56896,#56897,#56898,#56899,#56900,#56901,
#56902,#56903,#56904,#56905,#56906,#56907,#56908,#56909,#56910,#56911,#56912,
#56913,#56914,#56915,#56916,#56917,#56918,#56919,#56920,#56921,#56922,#56923,
#56924,#56925,#56926,#56927,#56928,#56929,#56930,#56931,#56932,#56933,#56934,
#56935,#56936,#56937,#56938,#56939,#56940,#56941,#56942,#56943,#56944,#56945,
#56946,#56947,#56948,#56949,#56950,#56951,#56952,#56953,#56954,#56955,#56956,
#56957,#56958,#56959,#56960,#56961,#56962,#56963,#56964,#56965,#56966,#56967,
#56968,#56969,#56970,#56971,#56972,#56973,#56974,#56975,#56976,#56977,#56978,
#56979,#56980,#56981,#56982,#56983,#56984,#56985,#56986,#56987,#56988,#56989,
#56990,#56991,#56992,#56993,#56994),.UNSPECIFIED.,.F.,.F.,(4,3,3,3,3,3,
3,3,3,3,3,3,3,3,3,3,3,3,3,3,3,3,3,3,3,3,3,3,3,3,3,3,3,3,3,3,3,3,3,3,3,3,
3,3,3,3,3,3,3,3,3,3,3,3,3,3,3,3,4),(-29.1739783669683,-29.0636179975722,
-28.9532180437743,-28.8426593424289,-28.732009659386,-28.6211452081831,
-28.581330241568,-28.4719930289838,-28.3624647915845,-28.2534185200467,
-28.1444366736126,-28.0354795479814,-27.9255514434335,-27.8164587020689,
-27.7061129159293,-27.5957671297898,-27.4864299184101,-27.3769016808603,
-27.2678554105611,-27.1588735653748,-27.0499164409984,-26.9399883352517,
-26.8308955951446,-26.7205498065781,-26.6102040180116,-26.5008668066609,
-26.3913385691074,-26.2822922988486,-26.1733104537067,-26.0643533293788,
-25.9544252235924,-25.8453324835434,-25.7349866948883,-25.6246409062333,
-25.5153036946033,-25.4057754570848,-25.2967291865319,-25.1877473410915,
-25.0787902164607,-24.9688621109593,-24.8597693706007,-24.7494235825279,
-24.6390777944551,-24.5297405829907,-24.4202123454515,-24.3111660750705,
-24.2021842298035,-24.0932271053477,-23.98329899968,-23.8742062594979,-23.7638604710874,
-23.6535146826769,-23.545626041452,-23.4378850553064,-23.3302497285488,
-23.2203855614481,-23.112800792144,-23.0017969261448,-22.8907930601457),
 .UNSPECIFIED.);
#680=B_SPLINE_CURVE_WITH_KNOTS('',3,(#56996,#56997,#56998,#56999,#57000,
#57001,#57002,#57003,#57004,#57005,#57006,#57007,#57008,#57009,#57010,#57011,
#57012,#57013,#57014,#57015,#57016,#57017,#57018,#57019,#57020,#57021,#57022,
#57023,#57024,#57025,#57026,#57027,#57028,#57029,#57030,#57031,#57032,#57033,
#57034,#57035,#57036,#57037,#57038,#57039,#57040,#57041,#57042,#57043,#57044,
#57045,#57046,#57047,#57048,#57049,#57050,#57051,#57052,#57053,#57054,#57055,
#57056,#57057,#57058,#57059,#57060,#57061,#57062,#57063,#57064,#57065,#57066,
#57067,#57068,#57069,#57070,#57071,#57072,#57073,#57074,#57075,#57076,#57077,
#57078,#57079,#57080,#57081,#57082,#57083,#57084,#57085,#57086,#57087,#57088,
#57089,#57090,#57091,#57092,#57093,#57094,#57095,#57096,#57097,#57098,#57099,
#57100,#57101,#57102,#57103,#57104,#57105,#57106,#57107,#57108,#57109,#57110,
#57111,#57112,#57113,#57114,#57115,#57116,#57117,#57118,#57119,#57120,#57121,
#57122,#57123,#57124,#57125,#57126,#57127,#57128,#57129,#57130,#57131,#57132,
#57133,#57134,#57135,#57136,#57137,#57138,#57139,#57140,#57141,#57142,#57143,
#57144,#57145,#57146,#57147,#57148,#57149,#57150,#57151,#57152,#57153,#57154,
#57155,#57156,#57157,#57158,#57159,#57160,#57161,#57162,#57163,#57164,#57165,
#57166,#57167),.UNSPECIFIED.,.F.,.F.,(4,3,3,3,3,3,3,3,3,3,3,3,3,3,3,3,3,
3,3,3,3,3,3,3,3,3,3,3,3,3,3,3,3,3,3,3,3,3,3,3,3,3,3,3,3,3,3,3,3,3,3,3,3,
3,3,3,3,4),(-22.8907930597887,-22.7446120253379,-22.6679515708987,-22.5586143595699,
-22.4490861220137,-22.3400398517639,-22.2310580066262,-22.1221008822976,
-22.0121727765033,-21.9030800364417,-21.7927342477811,-21.6823884591205,
-21.5730512477264,-21.4635230101784,-21.3544767398733,-21.2454948946841,
-21.136537770308,-21.0266096645666,-20.9175169244675,-20.8071711359049,
-20.6968253473423,-20.5874881347035,-20.477959897311,-20.3689136257507,
-20.2599317793062,-20.1509746536766,-20.0410465491485,-19.9319538078151,
-19.8216080216896,-19.7112622355641,-19.6019250260803,-19.4923967882935,
-19.3833505198729,-19.2743686765534,-19.1654115540288,-19.0554834464681,
-18.9463907081554,-18.8360449159706,-18.7256991237859,-18.6163619123579,
-18.5068336748142,-18.3977874045272,-18.2888055593755,-18.1798484350559,
-18.0699203292938,-17.9608275892965,-17.8504818006521,-17.7401360120077,
-17.6307987917964,-17.5212705553506,-17.4122242761684,-17.3032424221055,
-17.1942852888741,-17.0843571917129,-16.9752644429062,-16.8649186715678,
-16.7545729002295,-16.6076077526092),.UNSPECIFIED.);
#681=B_SPLINE_CURVE_WITH_KNOTS('',3,(#57169,#57170,#57171,#57172,#57173,
#57174,#57175,#57176,#57177,#57178,#57179,#57180,#57181,#57182,#57183,#57184,
#57185,#57186,#57187,#57188,#57189,#57190,#57191,#57192,#57193,#57194,#57195,
#57196,#57197,#57198,#57199,#57200,#57201,#57202,#57203,#57204,#57205,#57206,
#57207,#57208,#57209,#57210,#57211,#57212,#57213,#57214,#57215,#57216,#57217,
#57218,#57219,#57220,#57221,#57222,#57223,#57224,#57225,#57226,#57227,#57228,
#57229,#57230,#57231,#57232,#57233,#57234,#57235,#57236,#57237,#57238,#57239,
#57240,#57241,#57242,#57243,#57244,#57245,#57246,#57247,#57248,#57249,#57250,
#57251,#57252,#57253,#57254,#57255,#57256,#57257,#57258,#57259,#57260,#57261,
#57262,#57263,#57264,#57265,#57266,#57267,#57268,#57269,#57270,#57271,#57272,
#57273,#57274,#57275,#57276,#57277,#57278,#57279,#57280,#57281,#57282,#57283,
#57284,#57285,#57286,#57287,#57288,#57289,#57290,#57291,#57292,#57293,#57294,
#57295,#57296,#57297,#57298,#57299,#57300,#57301,#57302,#57303,#57304,#57305,
#57306,#57307,#57308,#57309,#57310,#57311,#57312,#57313,#57314,#57315,#57316,
#57317,#57318,#57319,#57320,#57321,#57322,#57323,#57324,#57325,#57326,#57327,
#57328,#57329,#57330,#57331,#57332,#57333,#57334,#57335,#57336,#57337,#57338,
#57339,#57340,#57341,#57342,#57343),.UNSPECIFIED.,.F.,.F.,(4,3,3,3,3,3,
3,3,3,3,3,3,3,3,3,3,3,3,3,3,3,3,3,3,3,3,3,3,3,3,3,3,3,3,3,3,3,3,3,3,3,3,
3,3,3,3,3,3,3,3,3,3,3,3,3,3,3,3,4),(-16.6076077522586,-16.4999871317891,
-16.3924795284533,-16.2850428992939,-16.1776353106626,-16.0701415239761,
-15.9626061582257,-15.8548783947035,-15.7690097884513,-15.6596725697738,
-15.5501443331362,-15.4410980560447,-15.3321162042733,-15.2231590735284,
-15.1132309743146,-15.0041382284364,-14.8937924525548,-14.7834466766731,
-14.6741094010268,-14.5645811715103,-14.4555348363317,-14.3465529262237,
-14.2375957369949,-14.1276676939699,-14.0185748899357,-13.9082292274153,
-13.7978835648949,-13.6885465279501,-13.579018268596,-13.4699721720189,
-13.3609904997933,-13.2520335473263,-13.1421052737739,-13.0330127010316,
-12.9226665770742,-12.8123204531167,-12.7029831151977,-12.5934548934653,
-12.4844085008043,-12.3754265351588,-12.2664692924144,-12.1565413046455,
-12.0474484526016,-11.93710289697,-11.8267573413385,-11.7174196867805,-11.6078915046279,
-11.4988447847093,-11.3898624887953,-11.2809049133659,-11.1709772424145,
-11.061884055738,-10.9515391426491,-10.8411942295603,-10.7275265913945,
-10.6141543120805,-10.5009590036298,-10.3879603830256,-10.3244224454296),
 .UNSPECIFIED.);
#682=B_SPLINE_CURVE_WITH_KNOTS('',3,(#57344,#57345,#57346,#57347,#57348,
#57349,#57350,#57351,#57352,#57353,#57354,#57355,#57356,#57357,#57358,#57359,
#57360,#57361,#57362,#57363,#57364,#57365,#57366,#57367,#57368,#57369,#57370,
#57371,#57372,#57373,#57374,#57375,#57376,#57377,#57378,#57379,#57380,#57381,
#57382,#57383,#57384,#57385,#57386,#57387,#57388,#57389,#57390,#57391,#57392,
#57393,#57394,#57395,#57396,#57397,#57398,#57399,#57400,#57401,#57402,#57403,
#57404,#57405,#57406,#57407,#57408,#57409,#57410,#57411,#57412,#57413,#57414,
#57415,#57416,#57417,#57418,#57419,#57420,#57421,#57422,#57423,#57424,#57425,
#57426,#57427,#57428,#57429,#57430,#57431,#57432,#57433,#57434,#57435,#57436,
#57437,#57438,#57439,#57440,#57441,#57442,#57443,#57444,#57445,#57446,#57447,
#57448,#57449,#57450,#57451,#57452,#57453,#57454,#57455,#57456,#57457,#57458,
#57459,#57460,#57461,#57462,#57463,#57464,#57465,#57466,#57467,#57468,#57469,
#57470,#57471,#57472,#57473,#57474,#57475,#57476,#57477,#57478,#57479,#57480,
#57481,#57482,#57483,#57484,#57485,#57486,#57487,#57488,#57489,#57490,#57491,
#57492,#57493,#57494,#57495,#57496,#57497,#57498,#57499,#57500,#57501,#57502,
#57503,#57504,#57505,#57506,#57507,#57508,#57509,#57510,#57511,#57512,#57513,
#57514,#57515,#57516,#57517,#57518),.UNSPECIFIED.,.F.,.F.,(4,3,3,3,3,3,
3,3,3,3,3,3,3,3,3,3,3,3,3,3,3,3,3,3,3,3,3,3,3,3,3,3,3,3,3,3,3,3,3,3,3,3,
3,3,3,3,3,3,3,3,3,3,3,3,3,3,3,3,4),(-10.3244224449722,-10.2072246131747,
-10.09165085566,-9.97364098672105,-9.85563111778205,-9.74629230873417,-9.63676427089288,
-9.52771643631158,-9.41873304372302,-9.30977439132236,-9.19984779499273,
-9.09075359148984,-8.98041079874685,-8.87006800600385,-8.76072802889233,
-8.651200137059,-8.5421510377115,-8.43316634803825,-8.32420636875443,-8.21428100012223,
-8.10518541331124,-7.99484515376844,-7.88450489422564,-7.7751805834152,
-7.66565073329423,-7.55661736705702,-7.44764839040374,-7.33870407734288,
-7.22876350361902,-7.11968328718189,-7.00931253481466,-6.89894178244744,
-6.78958698223486,-6.68006094328916,-6.57099734040682,-6.46199830753732,
-6.35302416858155,-6.24311279410347,-6.13400365621582,-6.02369116344252,
-5.91337867066923,-5.80402729489106,-5.69450082789106,-5.58543979974154,
-5.47644301843349,-5.36747080695317,-5.25755699493764,-5.14844897977771,
-5.03813226933437,-4.92781555889103,-4.81699325636299,-4.70927521869757,
-4.60165774558959,-4.49409900115545,-4.3865572407147,-4.27893084714527,
-4.17125183227785,-4.06341456574977,-4.04123713866671),.UNSPECIFIED.);
#683=B_SPLINE_CURVE_WITH_KNOTS('',3,(#57521,#57522,#57523,#57524,#57525,
#57526,#57527,#57528,#57529,#57530,#57531,#57532,#57533,#57534,#57535,#57536,
#57537,#57538,#57539,#57540,#57541,#57542,#57543,#57544,#57545,#57546,#57547,
#57548,#57549,#57550,#57551,#57552,#57553,#57554,#57555,#57556,#57557,#57558,
#57559,#57560,#57561,#57562,#57563,#57564,#57565,#57566,#57567,#57568,#57569,
#57570,#57571,#57572,#57573,#57574,#57575,#57576,#57577,#57578,#57579,#57580,
#57581,#57582,#57583,#57584,#57585,#57586,#57587,#57588,#57589,#57590,#57591,
#57592,#57593,#57594,#57595,#57596,#57597,#57598,#57599,#57600,#57601,#57602,
#57603,#57604,#57605,#57606,#57607,#57608,#57609,#57610,#57611,#57612,#57613,
#57614,#57615,#57616,#57617,#57618,#57619,#57620,#57621,#57622,#57623,#57624,
#57625,#57626,#57627,#57628,#57629,#57630,#57631,#57632,#57633,#57634,#57635,
#57636,#57637,#57638,#57639,#57640,#57641,#57642,#57643,#57644,#57645,#57646,
#57647,#57648),.UNSPECIFIED.,.F.,.F.,(4,2,2,2,2,2,2,2,2,2,2,2,2,2,2,2,2,
2,2,2,2,2,2,2,2,2,2,2,2,2,2,2,2,2,2,2,2,2,2,2,2,2,2,2,2,2,2,2,2,2,2,2,2,
2,2,2,2,2,2,2,2,2,2,4),(0.00160705595523008,0.00303069816735615,0.00693180054122098,
0.0260766323320663,0.049420593346507,0.0585609139609525,0.0656560107037017,
0.0743798200061914,0.0937641513165261,0.110101325445735,0.116979872190794,
0.122577131094358,0.12669519364253,0.131828585845873,0.150504578641132,
0.171476070898076,0.181712855199548,0.188854962153091,0.196843599860368,
0.212713122807251,0.234001272043188,0.241725383518611,0.247779851098417,
0.251833409216635,0.257185321475974,0.279991783609909,0.300899892154916,
0.309621683637536,0.316596312965283,0.325374349979552,0.347715335888014,
0.362524271249563,0.366943856318463,0.373364630364573,0.377399670873743,
0.382562133593276,0.407999153711683,0.422135731944411,0.43300947728638,
0.440204992883985,0.447938215265115,0.463241281223814,0.485457419866072,
0.493300190134225,0.499414348024838,0.503479248067671,0.508826310319265,
0.520139301900781,0.542675515758242,0.549285889728129,0.559413689495879,
0.566515011404271,0.574479153561681,0.590378227251692,0.61154715707313,
0.619242701470622,0.625276697613685,0.629328686156107,0.634703608039514,
0.661162014958273,0.676255444956648,0.685857530307112,0.692902189979643,
0.692945632510061),.UNSPECIFIED.);
#684=B_SPLINE_CURVE_WITH_KNOTS('',3,(#57651,#57652,#57653,#57654,#57655,
#57656,#57657,#57658,#57659,#57660,#57661,#57662,#57663,#57664,#57665,#57666,
#57667,#57668,#57669,#57670,#57671,#57672,#57673,#57674,#57675,#57676,#57677,
#57678,#57679,#57680,#57681,#57682,#57683,#57684,#57685,#57686,#57687,#57688,
#57689,#57690,#57691,#57692,#57693,#57694,#57695,#57696,#57697,#57698,#57699,
#57700,#57701,#57702,#57703,#57704,#57705,#57706,#57707,#57708,#57709,#57710,
#57711,#57712,#57713,#57714,#57715,#57716,#57717,#57718,#57719,#57720,#57721,
#57722,#57723,#57724,#57725,#57726,#57727,#57728,#57729,#57730,#57731,#57732,
#57733,#57734,#57735,#57736,#57737,#57738,#57739,#57740,#57741,#57742,#57743,
#57744,#57745,#57746),.UNSPECIFIED.,.F.,.F.,(4,2,2,2,2,2,2,2,2,2,2,2,2,
2,2,2,2,2,2,2,2,2,2,2,2,2,2,2,2,2,2,2,2,2,2,2,2,2,2,2,2,2,2,2,2,2,2,4),
(-1.21411811178252,-1.2110857626649,-1.20731545990233,-1.19202931788252,
-1.17330458064623,-1.16179203960238,-1.15395453653068,-1.14502478488769,
-1.12157541088363,-1.10401260242507,-1.09677384268193,-1.09094703605413,
-1.08731588903907,-1.08218585926128,-1.05768297439084,-1.03820959597564,
-1.02983271989945,-1.02311177806054,-1.01470975413155,-0.987446417451232,
-0.969965930718606,-0.964241892128248,-0.960312323131805,-0.955083467613174,
-0.930824734090043,-0.910628930123118,-0.901912198549083,-0.895527290220546,
-0.88680947190823,-0.867508963456092,-0.851083530299997,-0.844187046522863,
-0.83858083305714,-0.834463814367659,-0.829339717316834,-0.809974114266387,
-0.793130709011167,-0.787441919427184,-0.77821947502899,-0.771161585226906,
-0.762622592226985,-0.736096321326291,-0.723439689399553,-0.715117650593693,
-0.71077175182725,-0.706217361616685,-0.696338002095026,-0.692979258838884),
 .UNSPECIFIED.);
#685=B_SPLINE_CURVE_WITH_KNOTS('',3,(#57751,#57752,#57753,#57754,#57755,
#57756,#57757,#57758,#57759,#57760,#57761,#57762,#57763,#57764,#57765,#57766,
#57767,#57768,#57769,#57770,#57771,#57772,#57773,#57774,#57775,#57776,#57777,
#57778,#57779,#57780,#57781,#57782,#57783,#57784,#57785,#57786,#57787,#57788,
#57789,#57790,#57791,#57792,#57793,#57794,#57795,#57796,#57797,#57798,#57799,
#57800,#57801,#57802,#57803,#57804,#57805,#57806,#57807,#57808,#57809,#57810,
#57811,#57812,#57813,#57814,#57815,#57816,#57817,#57818,#57819,#57820,#57821,
#57822,#57823,#57824,#57825,#57826,#57827,#57828,#57829),.UNSPECIFIED.,
 .F.,.F.,(4,3,3,3,3,3,3,3,3,3,3,3,3,3,3,3,3,3,3,3,3,3,3,3,3,3,4),(-0.295872322228609,
-0.295800390457621,-0.276373981843977,-0.263250378750487,-0.258528391455822,
-0.239527378274684,-0.226792705152952,-0.222168728339882,-0.218676032022988,
-0.200352145245616,-0.182496347188838,-0.171319424938723,-0.161265355966744,
-0.15793468747543,-0.140841510700994,-0.137688493100165,-0.120125890536754,
-0.104799833849173,-0.101813032456204,-0.0849744272046009,-0.0684432950696122,
-0.0520509361631049,-0.0483399571277156,-0.032301942455842,-0.0162639277839685,
-0.00121618693710043,0.),.UNSPECIFIED.);
#686=B_SPLINE_CURVE_WITH_KNOTS('',3,(#57831,#57832,#57833,#57834),
 .UNSPECIFIED.,.F.,.F.,(4,4),(0.,0.00985912010464335),.UNSPECIFIED.);
#687=B_SPLINE_CURVE_WITH_KNOTS('',3,(#57835,#57836,#57837,#57838,#57839,
#57840,#57841,#57842,#57843,#57844,#57845,#57846,#57847,#57848,#57849,#57850,
#57851,#57852,#57853,#57854,#57855,#57856,#57857,#57858,#57859,#57860,#57861,
#57862,#57863,#57864,#57865,#57866,#57867,#57868,#57869,#57870,#57871,#57872,
#57873,#57874,#57875,#57876,#57877,#57878,#57879,#57880,#57881,#57882,#57883,
#57884,#57885,#57886,#57887,#57888,#57889,#57890,#57891,#57892,#57893,#57894,
#57895,#57896,#57897,#57898,#57899,#57900,#57901,#57902,#57903,#57904,#57905,
#57906,#57907,#57908,#57909,#57910,#57911,#57912,#57913,#57914,#57915,#57916,
#57917,#57918,#57919),.UNSPECIFIED.,.F.,.F.,(4,3,3,3,3,3,3,3,3,3,3,3,3,
3,3,3,3,3,3,3,3,3,3,3,3,3,3,3,4),(-0.300067541140097,-0.298264687041868,
-0.283066149434729,-0.274573360236698,-0.270084926663162,-0.266149262121986,
-0.250029687161801,-0.240714412789918,-0.236187237775089,-0.219496198515433,
-0.202395854960078,-0.191718287929847,-0.186414128238179,-0.183367582668388,
-0.165564985377019,-0.159558822602046,-0.142340885891246,-0.133217270038284,
-0.128037713880546,-0.12353774143095,-0.105513692533452,-0.086987532383811,
-0.0684672685495456,-0.0648082422231501,-0.0612577277857387,-0.0420101474320933,
-0.0227205645652813,-0.00360078115333159,0.),.UNSPECIFIED.);
#688=B_SPLINE_CURVE_WITH_KNOTS('',3,(#58129,#58130,#58131,#58132),
 .UNSPECIFIED.,.F.,.F.,(4,4),(-0.0228279319091498,0.),.UNSPECIFIED.);
#689=B_SPLINE_CURVE_WITH_KNOTS('',3,(#58134,#58135,#58136,#58137,#58138,
#58139,#58140,#58141,#58142,#58143,#58144,#58145,#58146,#58147,#58148,#58149,
#58150,#58151,#58152,#58153,#58154,#58155,#58156,#58157,#58158,#58159,#58160,
#58161,#58162,#58163,#58164,#58165,#58166,#58167,#58168,#58169,#58170,#58171,
#58172,#58173,#58174,#58175,#58176,#58177,#58178,#58179,#58180,#58181,#58182,
#58183,#58184,#58185,#58186,#58187,#58188,#58189,#58190,#58191,#58192,#58193,
#58194,#58195,#58196,#58197,#58198,#58199,#58200,#58201,#58202,#58203,#58204,
#58205,#58206,#58207,#58208,#58209,#58210,#58211,#58212,#58213,#58214,#58215,
#58216,#58217,#58218),.UNSPECIFIED.,.F.,.F.,(4,3,3,3,3,3,3,3,3,3,3,3,3,
3,3,3,3,3,3,3,3,3,3,3,3,3,3,3,4),(-0.300067541140124,-0.298264687041895,
-0.28306614612428,-0.274573356605969,-0.270084902423893,-0.266149257077711,
-0.250012130634623,-0.240714394402588,-0.236187236421063,-0.219545451825803,
-0.202445276722714,-0.191718285618554,-0.186414122583878,-0.183367577486661,
-0.165564980231119,-0.159558822602065,-0.14234088543558,-0.133217269957808,
-0.128037714183407,-0.123537741563047,-0.105564719399351,-0.0870159929477358,
-0.0684672664961207,-0.0648082516194149,-0.0612577300642884,-0.0419353127656361,
-0.022623645419663,-0.00360078661868575,0.),.UNSPECIFIED.);
#690=B_SPLINE_CURVE_WITH_KNOTS('',3,(#58219,#58220,#58221,#58222),
 .UNSPECIFIED.,.F.,.F.,(4,4),(-0.0098305480153634,0.),.UNSPECIFIED.);
#691=B_SPLINE_CURVE_WITH_KNOTS('',3,(#58227,#58228,#58229,#58230,#58231,
#58232,#58233,#58234,#58235,#58236,#58237,#58238,#58239,#58240,#58241,#58242,
#58243,#58244,#58245,#58246,#58247,#58248,#58249,#58250,#58251,#58252,#58253,
#58254,#58255,#58256,#58257,#58258,#58259,#58260,#58261,#58262,#58263,#58264,
#58265,#58266,#58267,#58268,#58269,#58270,#58271,#58272,#58273,#58274,#58275,
#58276,#58277,#58278,#58279,#58280,#58281,#58282,#58283,#58284,#58285,#58286,
#58287,#58288,#58289,#58290,#58291,#58292,#58293,#58294,#58295,#58296,#58297,
#58298,#58299,#58300,#58301,#58302,#58303,#58304,#58305),.UNSPECIFIED.,
 .F.,.F.,(4,3,3,3,3,3,3,3,3,3,3,3,3,3,3,3,3,3,3,3,3,3,3,3,3,3,4),(-0.295872351833489,
-0.295800390457537,-0.276036403287862,-0.263250379555454,-0.258528391470647,
-0.239521878863702,-0.226792705643256,-0.222168753783715,-0.21867604574408,
-0.200368561394637,-0.18251252301445,-0.171319438031604,-0.1612653787683,
-0.157934691378101,-0.140841517786507,-0.137688493100138,-0.120477431462621,
-0.104799834548055,-0.101813033019031,-0.0849850954960385,-0.0683039566266225,
-0.0520509292305863,-0.0483399545671687,-0.0325278496633223,-0.0162639248316611,
-0.00121617927212471,0.),.UNSPECIFIED.);
#692=B_SPLINE_CURVE_WITH_KNOTS('',3,(#58515,#58516,#58517,#58518),
 .UNSPECIFIED.,.F.,.F.,(4,4),(-0.0228763908153357,0.),.UNSPECIFIED.);
#899=B_SPLINE_SURFACE_WITH_KNOTS('',3,3,((#57921,#57922,#57923,#57924,#57925,
#57926,#57927,#57928,#57929,#57930,#57931,#57932,#57933,#57934,#57935,#57936,
#57937,#57938,#57939,#57940,#57941,#57942,#57943,#57944,#57945,#57946,#57947,
#57948,#57949,#57950,#57951,#57952,#57953,#57954,#57955,#57956,#57957,#57958,
#57959,#57960,#57961,#57962,#57963,#57964,#57965,#57966,#57967,#57968,#57969,
#57970,#57971,#57972),(#57973,#57974,#57975,#57976,#57977,#57978,#57979,
#57980,#57981,#57982,#57983,#57984,#57985,#57986,#57987,#57988,#57989,#57990,
#57991,#57992,#57993,#57994,#57995,#57996,#57997,#57998,#57999,#58000,#58001,
#58002,#58003,#58004,#58005,#58006,#58007,#58008,#58009,#58010,#58011,#58012,
#58013,#58014,#58015,#58016,#58017,#58018,#58019,#58020,#58021,#58022,#58023,
#58024),(#58025,#58026,#58027,#58028,#58029,#58030,#58031,#58032,#58033,
#58034,#58035,#58036,#58037,#58038,#58039,#58040,#58041,#58042,#58043,#58044,
#58045,#58046,#58047,#58048,#58049,#58050,#58051,#58052,#58053,#58054,#58055,
#58056,#58057,#58058,#58059,#58060,#58061,#58062,#58063,#58064,#58065,#58066,
#58067,#58068,#58069,#58070,#58071,#58072,#58073,#58074,#58075,#58076),
(#58077,#58078,#58079,#58080,#58081,#58082,#58083,#58084,#58085,#58086,
#58087,#58088,#58089,#58090,#58091,#58092,#58093,#58094,#58095,#58096,#58097,
#58098,#58099,#58100,#58101,#58102,#58103,#58104,#58105,#58106,#58107,#58108,
#58109,#58110,#58111,#58112,#58113,#58114,#58115,#58116,#58117,#58118,#58119,
#58120,#58121,#58122,#58123,#58124,#58125,#58126,#58127,#58128)),
 .UNSPECIFIED.,.F.,.F.,.F.,(4,4),(4,1,1,1,1,1,1,1,1,1,1,1,1,1,1,1,1,1,1,
1,1,1,1,1,1,1,1,1,1,1,1,1,1,1,1,1,1,1,1,1,1,1,1,1,1,1,1,1,1,4),(-0.000256380190589609,
0.0503983527946267),(8.33940042121162,9.32496353298982,10.310526644768,
11.2960897565462,12.2816528683244,13.2672159801026,14.2527790918808,15.2383422036591,
16.2239053154373,17.2094684272155,18.1950315389937,19.1805946507719,20.1661577625501,
21.1517208743283,22.1372839861065,23.1228470978847,24.1084102096629,25.0939733214411,
26.0795364332193,27.0650995449975,28.0506626567757,29.0362257685539,30.0217888803321,
31.0073519921103,31.9929151038885,32.9784782156668,33.964041327445,34.9496044392232,
35.9351675510014,36.9207306627796,37.9062937745578,38.891856886336,39.8774199981142,
40.8629831098924,41.8485462216706,42.8341093334488,43.819672445227,44.8052355570052,
45.7907986687834,46.7763617805616,47.7619248923398,48.747488004118,49.7330511158962,
50.7186142276745,51.7041773394527,52.6897404512309,53.6753035630091,54.6608666747873,
55.6464297865655,56.6322492785343),.UNSPECIFIED.);
#900=B_SPLINE_SURFACE_WITH_KNOTS('',3,3,((#58307,#58308,#58309,#58310,#58311,
#58312,#58313,#58314,#58315,#58316,#58317,#58318,#58319,#58320,#58321,#58322,
#58323,#58324,#58325,#58326,#58327,#58328,#58329,#58330,#58331,#58332,#58333,
#58334,#58335,#58336,#58337,#58338,#58339,#58340,#58341,#58342,#58343,#58344,
#58345,#58346,#58347,#58348,#58349,#58350,#58351,#58352,#58353,#58354,#58355,
#58356,#58357,#58358),(#58359,#58360,#58361,#58362,#58363,#58364,#58365,
#58366,#58367,#58368,#58369,#58370,#58371,#58372,#58373,#58374,#58375,#58376,
#58377,#58378,#58379,#58380,#58381,#58382,#58383,#58384,#58385,#58386,#58387,
#58388,#58389,#58390,#58391,#58392,#58393,#58394,#58395,#58396,#58397,#58398,
#58399,#58400,#58401,#58402,#58403,#58404,#58405,#58406,#58407,#58408,#58409,
#58410),(#58411,#58412,#58413,#58414,#58415,#58416,#58417,#58418,#58419,
#58420,#58421,#58422,#58423,#58424,#58425,#58426,#58427,#58428,#58429,#58430,
#58431,#58432,#58433,#58434,#58435,#58436,#58437,#58438,#58439,#58440,#58441,
#58442,#58443,#58444,#58445,#58446,#58447,#58448,#58449,#58450,#58451,#58452,
#58453,#58454,#58455,#58456,#58457,#58458,#58459,#58460,#58461,#58462),
(#58463,#58464,#58465,#58466,#58467,#58468,#58469,#58470,#58471,#58472,
#58473,#58474,#58475,#58476,#58477,#58478,#58479,#58480,#58481,#58482,#58483,
#58484,#58485,#58486,#58487,#58488,#58489,#58490,#58491,#58492,#58493,#58494,
#58495,#58496,#58497,#58498,#58499,#58500,#58501,#58502,#58503,#58504,#58505,
#58506,#58507,#58508,#58509,#58510,#58511,#58512,#58513,#58514)),
 .UNSPECIFIED.,.F.,.F.,.F.,(4,4),(4,1,1,1,1,1,1,1,1,1,1,1,1,1,1,1,1,1,1,
1,1,1,1,1,1,1,1,1,1,1,1,1,1,1,1,1,1,1,1,1,1,1,1,1,1,1,1,1,1,4),(-0.000235021283989965,
0.05040963628664),(11.6664697565963,12.6522892414772,13.6378523532554,14.6234154650336,
15.6089785768118,16.59454168859,17.5801048003682,18.5656679121464,19.5512310239246,
20.5367941357028,21.522357247481,22.5079203592592,23.4934834710374,24.4790465828156,
25.4646096945938,26.450172806372,27.4357359181503,28.4212990299285,29.4068621417067,
30.3924252534849,31.3779883652631,32.3635514770413,33.3491145888195,34.3346777005977,
35.3202408123759,36.3058039241541,37.2913670359323,38.2769301477105,39.2624932594887,
40.2480563712669,41.2336194830451,42.2191825948233,43.2047457066015,44.1903088183797,
45.175871930158,46.1614350419362,47.1469981537144,48.1325612654926,49.1181243772708,
50.103687489049,51.0892506008272,52.0748137126054,53.0603768243836,54.0459399361618,
55.03150304794,56.0170661597182,57.0026292714964,57.9881923832746,58.9737554950528,
59.959318606831),.UNSPECIFIED.);
#914=SHAPE_REPRESENTATION_RELATIONSHIP('SRR','None',#83309,#928);
#928=ADVANCED_BREP_SHAPE_REPRESENTATION('',(#956),#83214);
#942=STYLED_ITEM('',(#83388),#956);
#956=MANIFOLD_SOLID_BREP('Body1',#26938);
#1111=FACE_BOUND('',#4821,.T.);
#1112=FACE_BOUND('',#4935,.T.);
#1755=PLANE('',#28475);
#1756=PLANE('',#28478);
#1757=PLANE('',#28484);
#1758=PLANE('',#28488);
#1759=PLANE('',#28489);
#1760=PLANE('',#28490);
#1761=PLANE('',#28491);
#1762=PLANE('',#28531);
#1763=PLANE('',#28532);
#1764=PLANE('',#28533);
#1765=PLANE('',#28535);
#1766=PLANE('',#28536);
#1767=PLANE('',#28537);
#1768=PLANE('',#28539);
#1769=PLANE('',#28540);
#1770=PLANE('',#28541);
#1771=PLANE('',#28543);
#1772=PLANE('',#28544);
#1773=PLANE('',#28545);
#1774=PLANE('',#28547);
#1775=PLANE('',#28548);
#1776=PLANE('',#28549);
#1777=PLANE('',#28551);
#1778=PLANE('',#28552);
#1779=PLANE('',#28553);
#1780=PLANE('',#28555);
#1781=PLANE('',#28556);
#1782=PLANE('',#28557);
#1783=PLANE('',#28559);
#1784=PLANE('',#28560);
#1785=PLANE('',#28561);
#1786=PLANE('',#28564);
#1787=PLANE('',#28565);
#1788=PLANE('',#28566);
#1789=PLANE('',#28568);
#1790=PLANE('',#28569);
#1791=PLANE('',#28570);
#1792=PLANE('',#28572);
#1793=PLANE('',#28573);
#1794=PLANE('',#28574);
#1795=PLANE('',#28576);
#1796=PLANE('',#28577);
#1797=PLANE('',#28578);
#1798=PLANE('',#28580);
#1799=PLANE('',#28581);
#1800=PLANE('',#28582);
#1801=PLANE('',#28584);
#1802=PLANE('',#28585);
#1803=PLANE('',#28586);
#1804=PLANE('',#28588);
#1805=PLANE('',#28589);
#1806=PLANE('',#28590);
#1807=PLANE('',#28592);
#1808=PLANE('',#28593);
#1809=PLANE('',#28594);
#1810=PLANE('',#28596);
#1811=PLANE('',#28597);
#1812=PLANE('',#28598);
#1813=PLANE('',#28600);
#1814=PLANE('',#28601);
#1815=PLANE('',#28602);
#1816=PLANE('',#28604);
#1817=PLANE('',#28605);
#1818=PLANE('',#28606);
#1819=PLANE('',#28608);
#1820=PLANE('',#28609);
#1821=PLANE('',#28610);
#1822=PLANE('',#28612);
#1823=PLANE('',#28613);
#1824=PLANE('',#28614);
#1825=PLANE('',#28616);
#1826=PLANE('',#28617);
#1827=PLANE('',#28618);
#1828=PLANE('',#28620);
#1829=PLANE('',#28621);
#1830=PLANE('',#28622);
#1831=PLANE('',#28624);
#1832=PLANE('',#28625);
#1833=PLANE('',#28626);
#1834=PLANE('',#28628);
#1835=PLANE('',#28629);
#1836=PLANE('',#28630);
#1837=PLANE('',#28632);
#1838=PLANE('',#28633);
#1839=PLANE('',#28634);
#1840=PLANE('',#28636);
#1841=PLANE('',#28637);
#1842=PLANE('',#28638);
#1843=PLANE('',#28640);
#1844=PLANE('',#28641);
#1845=PLANE('',#28642);
#1846=PLANE('',#28644);
#1847=PLANE('',#28645);
#1848=PLANE('',#28646);
#1849=PLANE('',#28648);
#1850=PLANE('',#28649);
#1851=PLANE('',#28650);
#1852=PLANE('',#28652);
#1853=PLANE('',#28653);
#1854=PLANE('',#28654);
#1855=PLANE('',#28656);
#1856=PLANE('',#28657);
#1857=PLANE('',#28658);
#1858=PLANE('',#28660);
#1859=PLANE('',#28661);
#1860=PLANE('',#28662);
#1861=PLANE('',#28664);
#1862=PLANE('',#28665);
#1863=PLANE('',#28666);
#1864=PLANE('',#28668);
#1865=PLANE('',#28669);
#1866=PLANE('',#28670);
#1867=PLANE('',#28673);
#1868=PLANE('',#28674);
#1869=PLANE('',#28676);
#1870=PLANE('',#28678);
#1871=PLANE('',#28680);
#1872=PLANE('',#28682);
#1873=PLANE('',#28684);
#1874=PLANE('',#28687);
#1875=PLANE('',#28688);
#1876=PLANE('',#28689);
#1877=PLANE('',#28690);
#1878=PLANE('',#28691);
#1879=PLANE('',#28692);
#2308=CYLINDRICAL_SURFACE('',#28462,1.27);
#2309=CYLINDRICAL_SURFACE('',#28464,1.27);
#2310=CYLINDRICAL_SURFACE('',#28465,1.27);
#2311=CYLINDRICAL_SURFACE('',#28466,1.27);
#2312=CYLINDRICAL_SURFACE('',#28467,1.27);
#2313=CYLINDRICAL_SURFACE('',#28468,1.27);
#2314=CYLINDRICAL_SURFACE('',#28469,1.27);
#2315=CYLINDRICAL_SURFACE('',#28470,1.70434);
#2316=CYLINDRICAL_SURFACE('',#28473,1.27);
#2317=CYLINDRICAL_SURFACE('',#28672,2.8702);
#3277=FACE_OUTER_BOUND('',#4806,.T.);
#3278=FACE_OUTER_BOUND('',#4807,.T.);
#3279=FACE_OUTER_BOUND('',#4808,.T.);
#3280=FACE_OUTER_BOUND('',#4809,.T.);
#3281=FACE_OUTER_BOUND('',#4810,.T.);
#3282=FACE_OUTER_BOUND('',#4811,.T.);
#3283=FACE_OUTER_BOUND('',#4812,.T.);
#3284=FACE_OUTER_BOUND('',#4813,.T.);
#3285=FACE_OUTER_BOUND('',#4814,.T.);
#3286=FACE_OUTER_BOUND('',#4815,.T.);
#3287=FACE_OUTER_BOUND('',#4816,.T.);
#3288=FACE_OUTER_BOUND('',#4817,.T.);
#3289=FACE_OUTER_BOUND('',#4818,.T.);
#3290=FACE_OUTER_BOUND('',#4819,.T.);
#3291=FACE_OUTER_BOUND('',#4820,.T.);
#3292=FACE_OUTER_BOUND('',#4822,.T.);
#3293=FACE_OUTER_BOUND('',#4823,.T.);
#3294=FACE_OUTER_BOUND('',#4824,.T.);
#3295=FACE_OUTER_BOUND('',#4825,.T.);
#3296=FACE_OUTER_BOUND('',#4826,.T.);
#3297=FACE_OUTER_BOUND('',#4827,.T.);
#3298=FACE_OUTER_BOUND('',#4828,.T.);
#3299=FACE_OUTER_BOUND('',#4829,.T.);
#3300=FACE_OUTER_BOUND('',#4830,.T.);
#3301=FACE_OUTER_BOUND('',#4831,.T.);
#3302=FACE_OUTER_BOUND('',#4832,.T.);
#3303=FACE_OUTER_BOUND('',#4833,.T.);
#3304=FACE_OUTER_BOUND('',#4834,.T.);
#3305=FACE_OUTER_BOUND('',#4835,.T.);
#3306=FACE_OUTER_BOUND('',#4836,.T.);
#3307=FACE_OUTER_BOUND('',#4837,.T.);
#3308=FACE_OUTER_BOUND('',#4838,.T.);
#3309=FACE_OUTER_BOUND('',#4839,.T.);
#3310=FACE_OUTER_BOUND('',#4840,.T.);
#3311=FACE_OUTER_BOUND('',#4841,.T.);
#3312=FACE_OUTER_BOUND('',#4842,.T.);
#3313=FACE_OUTER_BOUND('',#4843,.T.);
#3314=FACE_OUTER_BOUND('',#4844,.T.);
#3315=FACE_OUTER_BOUND('',#4845,.T.);
#3316=FACE_OUTER_BOUND('',#4846,.T.);
#3317=FACE_OUTER_BOUND('',#4847,.T.);
#3318=FACE_OUTER_BOUND('',#4848,.T.);
#3319=FACE_OUTER_BOUND('',#4849,.T.);
#3320=FACE_OUTER_BOUND('',#4850,.T.);
#3321=FACE_OUTER_BOUND('',#4851,.T.);
#3322=FACE_OUTER_BOUND('',#4852,.T.);
#3323=FACE_OUTER_BOUND('',#4853,.T.);
#3324=FACE_OUTER_BOUND('',#4854,.T.);
#3325=FACE_OUTER_BOUND('',#4855,.T.);
#3326=FACE_OUTER_BOUND('',#4856,.T.);
#3327=FACE_OUTER_BOUND('',#4857,.T.);
#3328=FACE_OUTER_BOUND('',#4858,.T.);
#3329=FACE_OUTER_BOUND('',#4859,.T.);
#3330=FACE_OUTER_BOUND('',#4860,.T.);
#3331=FACE_OUTER_BOUND('',#4861,.T.);
#3332=FACE_OUTER_BOUND('',#4862,.T.);
#3333=FACE_OUTER_BOUND('',#4863,.T.);
#3334=FACE_OUTER_BOUND('',#4864,.T.);
#3335=FACE_OUTER_BOUND('',#4865,.T.);
#3336=FACE_OUTER_BOUND('',#4866,.T.);
#3337=FACE_OUTER_BOUND('',#4867,.T.);
#3338=FACE_OUTER_BOUND('',#4868,.T.);
#3339=FACE_OUTER_BOUND('',#4869,.T.);
#3340=FACE_OUTER_BOUND('',#4870,.T.);
#3341=FACE_OUTER_BOUND('',#4871,.T.);
#3342=FACE_OUTER_BOUND('',#4872,.T.);
#3343=FACE_OUTER_BOUND('',#4873,.T.);
#3344=FACE_OUTER_BOUND('',#4874,.T.);
#3345=FACE_OUTER_BOUND('',#4875,.T.);
#3346=FACE_OUTER_BOUND('',#4876,.T.);
#3347=FACE_OUTER_BOUND('',#4877,.T.);
#3348=FACE_OUTER_BOUND('',#4878,.T.);
#3349=FACE_OUTER_BOUND('',#4879,.T.);
#3350=FACE_OUTER_BOUND('',#4880,.T.);
#3351=FACE_OUTER_BOUND('',#4881,.T.);
#3352=FACE_OUTER_BOUND('',#4882,.T.);
#3353=FACE_OUTER_BOUND('',#4883,.T.);
#3354=FACE_OUTER_BOUND('',#4884,.T.);
#3355=FACE_OUTER_BOUND('',#4885,.T.);
#3356=FACE_OUTER_BOUND('',#4886,.T.);
#3357=FACE_OUTER_BOUND('',#4887,.T.);
#3358=FACE_OUTER_BOUND('',#4888,.T.);
#3359=FACE_OUTER_BOUND('',#4889,.T.);
#3360=FACE_OUTER_BOUND('',#4890,.T.);
#3361=FACE_OUTER_BOUND('',#4891,.T.);
#3362=FACE_OUTER_BOUND('',#4892,.T.);
#3363=FACE_OUTER_BOUND('',#4893,.T.);
#3364=FACE_OUTER_BOUND('',#4894,.T.);
#3365=FACE_OUTER_BOUND('',#4895,.T.);
#3366=FACE_OUTER_BOUND('',#4896,.T.);
#3367=FACE_OUTER_BOUND('',#4897,.T.);
#3368=FACE_OUTER_BOUND('',#4898,.T.);
#3369=FACE_OUTER_BOUND('',#4899,.T.);
#3370=FACE_OUTER_BOUND('',#4900,.T.);
#3371=FACE_OUTER_BOUND('',#4901,.T.);
#3372=FACE_OUTER_BOUND('',#4902,.T.);
#3373=FACE_OUTER_BOUND('',#4903,.T.);
#3374=FACE_OUTER_BOUND('',#4904,.T.);
#3375=FACE_OUTER_BOUND('',#4905,.T.);
#3376=FACE_OUTER_BOUND('',#4906,.T.);
#3377=FACE_OUTER_BOUND('',#4907,.T.);
#3378=FACE_OUTER_BOUND('',#4908,.T.);
#3379=FACE_OUTER_BOUND('',#4909,.T.);
#3380=FACE_OUTER_BOUND('',#4910,.T.);
#3381=FACE_OUTER_BOUND('',#4911,.T.);
#3382=FACE_OUTER_BOUND('',#4912,.T.);
#3383=FACE_OUTER_BOUND('',#4913,.T.);
#3384=FACE_OUTER_BOUND('',#4914,.T.);
#3385=FACE_OUTER_BOUND('',#4915,.T.);
#3386=FACE_OUTER_BOUND('',#4916,.T.);
#3387=FACE_OUTER_BOUND('',#4917,.T.);
#3388=FACE_OUTER_BOUND('',#4918,.T.);
#3389=FACE_OUTER_BOUND('',#4919,.T.);
#3390=FACE_OUTER_BOUND('',#4920,.T.);
#3391=FACE_OUTER_BOUND('',#4921,.T.);
#3392=FACE_OUTER_BOUND('',#4922,.T.);
#3393=FACE_OUTER_BOUND('',#4923,.T.);
#3394=FACE_OUTER_BOUND('',#4924,.T.);
#3395=FACE_OUTER_BOUND('',#4925,.T.);
#3396=FACE_OUTER_BOUND('',#4926,.T.);
#3397=FACE_OUTER_BOUND('',#4927,.T.);
#3398=FACE_OUTER_BOUND('',#4928,.T.);
#3399=FACE_OUTER_BOUND('',#4929,.T.);
#3400=FACE_OUTER_BOUND('',#4930,.T.);
#3401=FACE_OUTER_BOUND('',#4931,.T.);
#3402=FACE_OUTER_BOUND('',#4932,.T.);
#3403=FACE_OUTER_BOUND('',#4933,.T.);
#3404=FACE_OUTER_BOUND('',#4934,.T.);
#3405=FACE_OUTER_BOUND('',#4936,.T.);
#3406=FACE_OUTER_BOUND('',#4937,.T.);
#3407=FACE_OUTER_BOUND('',#4938,.T.);
#3408=FACE_OUTER_BOUND('',#4939,.T.);
#3409=FACE_OUTER_BOUND('',#4940,.T.);
#3410=FACE_OUTER_BOUND('',#4941,.T.);
#3411=FACE_OUTER_BOUND('',#4942,.T.);
#3412=FACE_OUTER_BOUND('',#4943,.T.);
#3413=FACE_OUTER_BOUND('',#4944,.T.);
#3414=FACE_OUTER_BOUND('',#4945,.T.);
#3415=FACE_OUTER_BOUND('',#4946,.T.);
#3416=FACE_OUTER_BOUND('',#4947,.T.);
#3417=FACE_OUTER_BOUND('',#4948,.T.);
#4806=EDGE_LOOP('',(#22658,#22659,#22660,#22661));
#4807=EDGE_LOOP('',(#22662,#22663,#22664,#22665));
#4808=EDGE_LOOP('',(#22666,#22667,#22668,#22669,#22670,#22671));
#4809=EDGE_LOOP('',(#22672,#22673,#22674,#22675));
#4810=EDGE_LOOP('',(#22676,#22677,#22678,#22679,#22680,#22681));
#4811=EDGE_LOOP('',(#22682,#22683,#22684,#22685));
#4812=EDGE_LOOP('',(#22686,#22687,#22688,#22689,#22690,#22691));
#4813=EDGE_LOOP('',(#22692,#22693,#22694,#22695,#22696,#22697,#22698,#22699,
#22700,#22701,#22702,#22703,#22704,#22705,#22706,#22707,#22708,#22709,#22710,
#22711));
#4814=EDGE_LOOP('',(#22712,#22713,#22714,#22715));
#4815=EDGE_LOOP('',(#22716,#22717,#22718,#22719,#22720,#22721));
#4816=EDGE_LOOP('',(#22722,#22723,#22724,#22725,#22726,#22727,#22728,#22729,
#22730,#22731,#22732,#22733,#22734,#22735,#22736,#22737,#22738,#22739,#22740,
#22741,#22742,#22743,#22744,#22745));
#4817=EDGE_LOOP('',(#22746,#22747,#22748,#22749,#22750,#22751));
#4818=EDGE_LOOP('',(#22752,#22753,#22754,#22755,#22756,#22757,#22758,#22759,
#22760,#22761,#22762,#22763,#22764,#22765,#22766,#22767,#22768,#22769,#22770,
#22771,#22772,#22773,#22774,#22775));
#4819=EDGE_LOOP('',(#22776,#22777,#22778,#22779,#22780,#22781,#22782));
#4820=EDGE_LOOP('',(#22783));
#4821=EDGE_LOOP('',(#22784));
#4822=EDGE_LOOP('',(#22785,#22786,#22787,#22788,#22789,#22790,#22791));
#4823=EDGE_LOOP('',(#22792));
#4824=EDGE_LOOP('',(#22793,#22794,#22795,#22796));
#4825=EDGE_LOOP('',(#22797,#22798,#22799,#22800));
#4826=EDGE_LOOP('',(#22801,#22802,#22803));
#4827=EDGE_LOOP('',(#22804,#22805,#22806,#22807,#22808,#22809,#22810,#22811,
#22812,#22813,#22814,#22815,#22816,#22817,#22818,#22819,#22820,#22821,#22822,
#22823,#22824,#22825,#22826,#22827,#22828,#22829,#22830,#22831,#22832,#22833,
#22834,#22835,#22836,#22837,#22838,#22839,#22840,#22841,#22842,#22843,#22844,
#22845,#22846,#22847,#22848,#22849,#22850,#22851,#22852,#22853,#22854,#22855,
#22856,#22857,#22858,#22859,#22860,#22861,#22862,#22863,#22864,#22865,#22866,
#22867,#22868,#22869,#22870,#22871,#22872,#22873,#22874,#22875,#22876,#22877,
#22878,#22879,#22880,#22881,#22882,#22883,#22884,#22885,#22886,#22887,#22888,
#22889,#22890,#22891,#22892,#22893,#22894,#22895,#22896,#22897,#22898,#22899,
#22900,#22901,#22902,#22903,#22904,#22905,#22906,#22907,#22908,#22909,#22910,
#22911,#22912,#22913,#22914));
#4828=EDGE_LOOP('',(#22915,#22916,#22917,#22918));
#4829=EDGE_LOOP('',(#22919,#22920,#22921,#22922));
#4830=EDGE_LOOP('',(#22923,#22924,#22925));
#4831=EDGE_LOOP('',(#22926,#22927,#22928,#22929));
#4832=EDGE_LOOP('',(#22930,#22931,#22932,#22933));
#4833=EDGE_LOOP('',(#22934,#22935,#22936));
#4834=EDGE_LOOP('',(#22937,#22938,#22939,#22940));
#4835=EDGE_LOOP('',(#22941,#22942,#22943,#22944));
#4836=EDGE_LOOP('',(#22945,#22946,#22947));
#4837=EDGE_LOOP('',(#22948,#22949,#22950,#22951));
#4838=EDGE_LOOP('',(#22952,#22953,#22954,#22955));
#4839=EDGE_LOOP('',(#22956,#22957,#22958));
#4840=EDGE_LOOP('',(#22959,#22960,#22961,#22962));
#4841=EDGE_LOOP('',(#22963,#22964,#22965,#22966));
#4842=EDGE_LOOP('',(#22967,#22968,#22969));
#4843=EDGE_LOOP('',(#22970,#22971,#22972,#22973));
#4844=EDGE_LOOP('',(#22974,#22975,#22976,#22977));
#4845=EDGE_LOOP('',(#22978,#22979,#22980));
#4846=EDGE_LOOP('',(#22981,#22982,#22983,#22984));
#4847=EDGE_LOOP('',(#22985,#22986,#22987,#22988));
#4848=EDGE_LOOP('',(#22989,#22990,#22991));
#4849=EDGE_LOOP('',(#22992,#22993,#22994,#22995));
#4850=EDGE_LOOP('',(#22996,#22997,#22998,#22999));
#4851=EDGE_LOOP('',(#23000,#23001,#23002,#23003));
#4852=EDGE_LOOP('',(#23004,#23005,#23006,#23007));
#4853=EDGE_LOOP('',(#23008,#23009,#23010,#23011));
#4854=EDGE_LOOP('',(#23012,#23013,#23014));
#4855=EDGE_LOOP('',(#23015,#23016,#23017,#23018));
#4856=EDGE_LOOP('',(#23019,#23020,#23021,#23022));
#4857=EDGE_LOOP('',(#23023,#23024,#23025));
#4858=EDGE_LOOP('',(#23026,#23027,#23028,#23029));
#4859=EDGE_LOOP('',(#23030,#23031,#23032,#23033));
#4860=EDGE_LOOP('',(#23034,#23035,#23036));
#4861=EDGE_LOOP('',(#23037,#23038,#23039,#23040));
#4862=EDGE_LOOP('',(#23041,#23042,#23043,#23044));
#4863=EDGE_LOOP('',(#23045,#23046,#23047));
#4864=EDGE_LOOP('',(#23048,#23049,#23050,#23051));
#4865=EDGE_LOOP('',(#23052,#23053,#23054,#23055));
#4866=EDGE_LOOP('',(#23056,#23057,#23058));
#4867=EDGE_LOOP('',(#23059,#23060,#23061,#23062));
#4868=EDGE_LOOP('',(#23063,#23064,#23065,#23066));
#4869=EDGE_LOOP('',(#23067,#23068,#23069));
#4870=EDGE_LOOP('',(#23070,#23071,#23072,#23073));
#4871=EDGE_LOOP('',(#23074,#23075,#23076,#23077));
#4872=EDGE_LOOP('',(#23078,#23079,#23080));
#4873=EDGE_LOOP('',(#23081,#23082,#23083,#23084));
#4874=EDGE_LOOP('',(#23085,#23086,#23087,#23088));
#4875=EDGE_LOOP('',(#23089,#23090,#23091));
#4876=EDGE_LOOP('',(#23092,#23093,#23094,#23095));
#4877=EDGE_LOOP('',(#23096,#23097,#23098,#23099));
#4878=EDGE_LOOP('',(#23100,#23101,#23102));
#4879=EDGE_LOOP('',(#23103,#23104,#23105,#23106));
#4880=EDGE_LOOP('',(#23107,#23108,#23109,#23110));
#4881=EDGE_LOOP('',(#23111,#23112,#23113));
#4882=EDGE_LOOP('',(#23114,#23115,#23116,#23117));
#4883=EDGE_LOOP('',(#23118,#23119,#23120,#23121));
#4884=EDGE_LOOP('',(#23122,#23123,#23124));
#4885=EDGE_LOOP('',(#23125,#23126,#23127,#23128));
#4886=EDGE_LOOP('',(#23129,#23130,#23131,#23132));
#4887=EDGE_LOOP('',(#23133,#23134,#23135));
#4888=EDGE_LOOP('',(#23136,#23137,#23138,#23139));
#4889=EDGE_LOOP('',(#23140,#23141,#23142,#23143));
#4890=EDGE_LOOP('',(#23144,#23145,#23146));
#4891=EDGE_LOOP('',(#23147,#23148,#23149,#23150));
#4892=EDGE_LOOP('',(#23151,#23152,#23153,#23154));
#4893=EDGE_LOOP('',(#23155,#23156,#23157));
#4894=EDGE_LOOP('',(#23158,#23159,#23160,#23161));
#4895=EDGE_LOOP('',(#23162,#23163,#23164,#23165));
#4896=EDGE_LOOP('',(#23166,#23167,#23168));
#4897=EDGE_LOOP('',(#23169,#23170,#23171,#23172));
#4898=EDGE_LOOP('',(#23173,#23174,#23175,#23176));
#4899=EDGE_LOOP('',(#23177,#23178,#23179));
#4900=EDGE_LOOP('',(#23180,#23181,#23182,#23183));
#4901=EDGE_LOOP('',(#23184,#23185,#23186,#23187));
#4902=EDGE_LOOP('',(#23188,#23189,#23190));
#4903=EDGE_LOOP('',(#23191,#23192,#23193,#23194));
#4904=EDGE_LOOP('',(#23195,#23196,#23197,#23198));
#4905=EDGE_LOOP('',(#23199,#23200,#23201));
#4906=EDGE_LOOP('',(#23202,#23203,#23204,#23205));
#4907=EDGE_LOOP('',(#23206,#23207,#23208,#23209));
#4908=EDGE_LOOP('',(#23210,#23211,#23212));
#4909=EDGE_LOOP('',(#23213,#23214,#23215,#23216));
#4910=EDGE_LOOP('',(#23217,#23218,#23219,#23220));
#4911=EDGE_LOOP('',(#23221,#23222,#23223));
#4912=EDGE_LOOP('',(#23224,#23225,#23226,#23227));
#4913=EDGE_LOOP('',(#23228,#23229,#23230,#23231));
#4914=EDGE_LOOP('',(#23232,#23233,#23234));
#4915=EDGE_LOOP('',(#23235,#23236,#23237,#23238));
#4916=EDGE_LOOP('',(#23239,#23240,#23241,#23242));
#4917=EDGE_LOOP('',(#23243,#23244,#23245));
#4918=EDGE_LOOP('',(#23246,#23247,#23248,#23249));
#4919=EDGE_LOOP('',(#23250,#23251,#23252,#23253));
#4920=EDGE_LOOP('',(#23254,#23255,#23256));
#4921=EDGE_LOOP('',(#23257,#23258,#23259,#23260));
#4922=EDGE_LOOP('',(#23261,#23262,#23263,#23264));
#4923=EDGE_LOOP('',(#23265,#23266,#23267));
#4924=EDGE_LOOP('',(#23268,#23269,#23270,#23271));
#4925=EDGE_LOOP('',(#23272,#23273,#23274,#23275));
#4926=EDGE_LOOP('',(#23276,#23277,#23278));
#4927=EDGE_LOOP('',(#23279,#23280,#23281,#23282));
#4928=EDGE_LOOP('',(#23283,#23284,#23285,#23286));
#4929=EDGE_LOOP('',(#23287,#23288,#23289));
#4930=EDGE_LOOP('',(#23290,#23291,#23292,#23293));
#4931=EDGE_LOOP('',(#23294,#23295,#23296,#23297));
#4932=EDGE_LOOP('',(#23298,#23299,#23300));
#4933=EDGE_LOOP('',(#23301,#23302,#23303,#23304,#23305,#23306,#23307,#23308,
#23309,#23310,#23311,#23312,#23313,#23314,#23315,#23316,#23317,#23318,#23319,
#23320,#23321,#23322,#23323,#23324,#23325,#23326,#23327,#23328,#23329,#23330,
#23331,#23332,#23333,#23334,#23335,#23336,#23337,#23338,#23339,#23340,#23341,
#23342,#23343,#23344,#23345,#23346,#23347,#23348,#23349,#23350,#23351,#23352,
#23353,#23354,#23355,#23356,#23357,#23358,#23359,#23360,#23361,#23362,#23363,
#23364,#23365,#23366,#23367,#23368,#23369,#23370,#23371,#23372,#23373,#23374,
#23375,#23376,#23377,#23378,#23379,#23380,#23381,#23382,#23383,#23384,#23385,
#23386,#23387,#23388,#23389,#23390,#23391,#23392,#23393,#23394,#23395,#23396,
#23397,#23398,#23399,#23400,#23401,#23402,#23403,#23404,#23405,#23406,#23407,
#23408,#23409,#23410,#23411,#23412,#23413,#23414,#23415,#23416,#23417,#23418,
#23419,#23420,#23421,#23422,#23423,#23424,#23425,#23426,#23427,#23428,#23429,
#23430,#23431,#23432,#23433,#23434,#23435,#23436,#23437,#23438,#23439,#23440,
#23441,#23442,#23443,#23444,#23445,#23446,#23447,#23448));
#4934=EDGE_LOOP('',(#23449));
#4935=EDGE_LOOP('',(#23450,#23451,#23452,#23453,#23454,#23455));
#4936=EDGE_LOOP('',(#23456,#23457));
#4937=EDGE_LOOP('',(#23458,#23459));
#4938=EDGE_LOOP('',(#23460,#23461));
#4939=EDGE_LOOP('',(#23462,#23463));
#4940=EDGE_LOOP('',(#23464,#23465));
#4941=EDGE_LOOP('',(#23466,#23467));
#4942=EDGE_LOOP('',(#23468,#23469,#23470,#23471,#23472,#23473,#23474,#23475));
#4943=EDGE_LOOP('',(#23476,#23477,#23478,#23479));
#4944=EDGE_LOOP('',(#23480,#23481,#23482,#23483));
#4945=EDGE_LOOP('',(#23484,#23485,#23486,#23487));
#4946=EDGE_LOOP('',(#23488,#23489,#23490,#23491));
#4947=EDGE_LOOP('',(#23492,#23493,#23494,#23495));
#4948=EDGE_LOOP('',(#23496,#23497,#23498,#23499));
#7125=LINE('',#53161,#9636);
#7126=LINE('',#53348,#9637);
#7127=LINE('',#53646,#9638);
#7128=LINE('',#53946,#9639);
#7129=LINE('',#54236,#9640);
#7130=LINE('',#54534,#9641);
#7131=LINE('',#54826,#9642);
#7132=LINE('',#58528,#9643);
#7133=LINE('',#58534,#9644);
#7134=LINE('',#58536,#9645);
#7135=LINE('',#58538,#9646);
#7136=LINE('',#58545,#9647);
#7137=LINE('',#58549,#9648);
#7138=LINE('',#58905,#9649);
#7139=LINE('',#58909,#9650);
#7140=LINE('',#58911,#9651);
#7141=LINE('',#58912,#9652);
#7142=LINE('',#58915,#9653);
#7143=LINE('',#58916,#9654);
#7144=LINE('',#58921,#9655);
#7145=LINE('',#58923,#9656);
#7146=LINE('',#58924,#9657);
#7147=LINE('',#58927,#9658);
#7148=LINE('',#58928,#9659);
#7149=LINE('',#58933,#9660);
#7150=LINE('',#58935,#9661);
#7151=LINE('',#58936,#9662);
#7152=LINE('',#58939,#9663);
#7153=LINE('',#58940,#9664);
#7154=LINE('',#58945,#9665);
#7155=LINE('',#58947,#9666);
#7156=LINE('',#58948,#9667);
#7157=LINE('',#58951,#9668);
#7158=LINE('',#58952,#9669);
#7159=LINE('',#58957,#9670);
#7160=LINE('',#58959,#9671);
#7161=LINE('',#58960,#9672);
#7162=LINE('',#58963,#9673);
#7163=LINE('',#58964,#9674);
#7164=LINE('',#58969,#9675);
#7165=LINE('',#58971,#9676);
#7166=LINE('',#58972,#9677);
#7167=LINE('',#58975,#9678);
#7168=LINE('',#58976,#9679);
#7169=LINE('',#58981,#9680);
#7170=LINE('',#58983,#9681);
#7171=LINE('',#58984,#9682);
#7172=LINE('',#58987,#9683);
#7173=LINE('',#58988,#9684);
#7174=LINE('',#58993,#9685);
#7175=LINE('',#58995,#9686);
#7176=LINE('',#58996,#9687);
#7177=LINE('',#58999,#9688);
#7178=LINE('',#59000,#9689);
#7179=LINE('',#59007,#9690);
#7180=LINE('',#59009,#9691);
#7181=LINE('',#59010,#9692);
#7182=LINE('',#59013,#9693);
#7183=LINE('',#59014,#9694);
#7184=LINE('',#59019,#9695);
#7185=LINE('',#59021,#9696);
#7186=LINE('',#59022,#9697);
#7187=LINE('',#59025,#9698);
#7188=LINE('',#59026,#9699);
#7189=LINE('',#59031,#9700);
#7190=LINE('',#59033,#9701);
#7191=LINE('',#59034,#9702);
#7192=LINE('',#59037,#9703);
#7193=LINE('',#59038,#9704);
#7194=LINE('',#59043,#9705);
#7195=LINE('',#59045,#9706);
#7196=LINE('',#59046,#9707);
#7197=LINE('',#59049,#9708);
#7198=LINE('',#59050,#9709);
#7199=LINE('',#59055,#9710);
#7200=LINE('',#59057,#9711);
#7201=LINE('',#59058,#9712);
#7202=LINE('',#59061,#9713);
#7203=LINE('',#59062,#9714);
#7204=LINE('',#59067,#9715);
#7205=LINE('',#59069,#9716);
#7206=LINE('',#59070,#9717);
#7207=LINE('',#59073,#9718);
#7208=LINE('',#59074,#9719);
#7209=LINE('',#59079,#9720);
#7210=LINE('',#59081,#9721);
#7211=LINE('',#59082,#9722);
#7212=LINE('',#59085,#9723);
#7213=LINE('',#59086,#9724);
#7214=LINE('',#59091,#9725);
#7215=LINE('',#59093,#9726);
#7216=LINE('',#59094,#9727);
#7217=LINE('',#59097,#9728);
#7218=LINE('',#59098,#9729);
#7219=LINE('',#59103,#9730);
#7220=LINE('',#59105,#9731);
#7221=LINE('',#59106,#9732);
#7222=LINE('',#59109,#9733);
#7223=LINE('',#59110,#9734);
#7224=LINE('',#59115,#9735);
#7225=LINE('',#59117,#9736);
#7226=LINE('',#59118,#9737);
#7227=LINE('',#59121,#9738);
#7228=LINE('',#59122,#9739);
#7229=LINE('',#59127,#9740);
#7230=LINE('',#59129,#9741);
#7231=LINE('',#59130,#9742);
#7232=LINE('',#59133,#9743);
#7233=LINE('',#59134,#9744);
#7234=LINE('',#59139,#9745);
#7235=LINE('',#59141,#9746);
#7236=LINE('',#59142,#9747);
#7237=LINE('',#59145,#9748);
#7238=LINE('',#59146,#9749);
#7239=LINE('',#59151,#9750);
#7240=LINE('',#59153,#9751);
#7241=LINE('',#59154,#9752);
#7242=LINE('',#59157,#9753);
#7243=LINE('',#59158,#9754);
#7244=LINE('',#59163,#9755);
#7245=LINE('',#59165,#9756);
#7246=LINE('',#59166,#9757);
#7247=LINE('',#59169,#9758);
#7248=LINE('',#59170,#9759);
#7249=LINE('',#59175,#9760);
#7250=LINE('',#59177,#9761);
#7251=LINE('',#59178,#9762);
#7252=LINE('',#59181,#9763);
#7253=LINE('',#59182,#9764);
#7254=LINE('',#59187,#9765);
#7255=LINE('',#59189,#9766);
#7256=LINE('',#59190,#9767);
#7257=LINE('',#59193,#9768);
#7258=LINE('',#59194,#9769);
#7259=LINE('',#59199,#9770);
#7260=LINE('',#59201,#9771);
#7261=LINE('',#59202,#9772);
#7262=LINE('',#59205,#9773);
#7263=LINE('',#59206,#9774);
#7264=LINE('',#59211,#9775);
#7265=LINE('',#59213,#9776);
#7266=LINE('',#59214,#9777);
#7267=LINE('',#59217,#9778);
#7268=LINE('',#59218,#9779);
#7269=LINE('',#59223,#9780);
#7270=LINE('',#59225,#9781);
#7271=LINE('',#59226,#9782);
#7272=LINE('',#59229,#9783);
#7273=LINE('',#59230,#9784);
#7274=LINE('',#59235,#9785);
#7275=LINE('',#59237,#9786);
#7276=LINE('',#59238,#9787);
#7277=LINE('',#59241,#9788);
#7278=LINE('',#59242,#9789);
#7279=LINE('',#59247,#9790);
#7280=LINE('',#59249,#9791);
#7281=LINE('',#59250,#9792);
#7282=LINE('',#59253,#9793);
#7283=LINE('',#59254,#9794);
#7284=LINE('',#59259,#9795);
#7285=LINE('',#59261,#9796);
#7286=LINE('',#59262,#9797);
#7287=LINE('',#59265,#9798);
#7288=LINE('',#59266,#9799);
#7289=LINE('',#59271,#9800);
#7290=LINE('',#59273,#9801);
#7291=LINE('',#59274,#9802);
#7292=LINE('',#59277,#9803);
#7293=LINE('',#59278,#9804);
#7294=LINE('',#59283,#9805);
#7295=LINE('',#59285,#9806);
#7296=LINE('',#59286,#9807);
#7297=LINE('',#59289,#9808);
#7298=LINE('',#59290,#9809);
#7299=LINE('',#59295,#9810);
#7300=LINE('',#59297,#9811);
#7301=LINE('',#59298,#9812);
#7302=LINE('',#59301,#9813);
#7303=LINE('',#59302,#9814);
#7304=LINE('',#59307,#9815);
#7305=LINE('',#59309,#9816);
#7306=LINE('',#59310,#9817);
#7307=LINE('',#59313,#9818);
#7308=LINE('',#59314,#9819);
#7309=LINE('',#59319,#9820);
#7310=LINE('',#59321,#9821);
#7311=LINE('',#59322,#9822);
#7312=LINE('',#59325,#9823);
#7313=LINE('',#59326,#9824);
#7314=LINE('',#59330,#9825);
#7315=LINE('',#59334,#9826);
#7316=LINE('',#59336,#9827);
#7317=LINE('',#59338,#9828);
#7318=LINE('',#59340,#9829);
#7319=LINE('',#59342,#9830);
#7320=LINE('',#59343,#9831);
#7321=LINE('',#59347,#9832);
#7322=LINE('',#59351,#9833);
#7323=LINE('',#59355,#9834);
#7324=LINE('',#59359,#9835);
#7325=LINE('',#59363,#9836);
#7326=LINE('',#59366,#9837);
#7327=LINE('',#59370,#9838);
#7328=LINE('',#59372,#9839);
#7329=LINE('',#59373,#9840);
#7330=LINE('',#59375,#9841);
#7331=LINE('',#59377,#9842);
#7332=LINE('',#59379,#9843);
#7333=LINE('',#59381,#9844);
#9636=VECTOR('',#33833,1.27);
#9637=VECTOR('',#33838,1.27);
#9638=VECTOR('',#33841,1.27);
#9639=VECTOR('',#33844,1.27);
#9640=VECTOR('',#33847,1.27);
#9641=VECTOR('',#33850,1.27);
#9642=VECTOR('',#33853,1.27);
#9643=VECTOR('',#33888,1.52934);
#9644=VECTOR('',#33895,10.);
#9645=VECTOR('',#33896,9.99999999999999);
#9646=VECTOR('',#33897,10.);
#9647=VECTOR('',#33900,10.);
#9648=VECTOR('',#33901,10.);
#9649=VECTOR('',#33980,2.7202);
#9650=VECTOR('',#33985,10.);
#9651=VECTOR('',#33986,10.);
#9652=VECTOR('',#33987,10.);
#9653=VECTOR('',#33990,10.);
#9654=VECTOR('',#33991,10.);
#9655=VECTOR('',#33998,10.);
#9656=VECTOR('',#33999,10.);
#9657=VECTOR('',#34000,10.);
#9658=VECTOR('',#34003,10.);
#9659=VECTOR('',#34004,10.);
#9660=VECTOR('',#34011,10.);
#9661=VECTOR('',#34012,10.);
#9662=VECTOR('',#34013,10.);
#9663=VECTOR('',#34016,10.);
#9664=VECTOR('',#34017,10.);
#9665=VECTOR('',#34024,10.);
#9666=VECTOR('',#34025,10.);
#9667=VECTOR('',#34026,10.);
#9668=VECTOR('',#34029,10.);
#9669=VECTOR('',#34030,10.);
#9670=VECTOR('',#34037,10.);
#9671=VECTOR('',#34038,9.99999999999999);
#9672=VECTOR('',#34039,10.);
#9673=VECTOR('',#34042,10.);
#9674=VECTOR('',#34043,10.);
#9675=VECTOR('',#34050,10.);
#9676=VECTOR('',#34051,10.);
#9677=VECTOR('',#34052,10.);
#9678=VECTOR('',#34055,10.);
#9679=VECTOR('',#34056,10.);
#9680=VECTOR('',#34063,10.);
#9681=VECTOR('',#34064,10.);
#9682=VECTOR('',#34065,10.);
#9683=VECTOR('',#34068,10.);
#9684=VECTOR('',#34069,9.99999999999999);
#9685=VECTOR('',#34076,10.);
#9686=VECTOR('',#34077,10.);
#9687=VECTOR('',#34078,10.);
#9688=VECTOR('',#34081,10.);
#9689=VECTOR('',#34082,10.);
#9690=VECTOR('',#34091,10.);
#9691=VECTOR('',#34092,10.);
#9692=VECTOR('',#34093,10.);
#9693=VECTOR('',#34096,10.);
#9694=VECTOR('',#34097,10.);
#9695=VECTOR('',#34104,10.);
#9696=VECTOR('',#34105,10.);
#9697=VECTOR('',#34106,10.);
#9698=VECTOR('',#34109,10.);
#9699=VECTOR('',#34110,10.);
#9700=VECTOR('',#34117,10.);
#9701=VECTOR('',#34118,10.);
#9702=VECTOR('',#34119,10.);
#9703=VECTOR('',#34122,10.);
#9704=VECTOR('',#34123,10.);
#9705=VECTOR('',#34130,10.);
#9706=VECTOR('',#34131,10.);
#9707=VECTOR('',#34132,10.);
#9708=VECTOR('',#34135,10.);
#9709=VECTOR('',#34136,10.);
#9710=VECTOR('',#34143,10.);
#9711=VECTOR('',#34144,10.);
#9712=VECTOR('',#34145,10.);
#9713=VECTOR('',#34148,10.);
#9714=VECTOR('',#34149,10.);
#9715=VECTOR('',#34156,10.);
#9716=VECTOR('',#34157,9.99999999999999);
#9717=VECTOR('',#34158,10.);
#9718=VECTOR('',#34161,10.);
#9719=VECTOR('',#34162,10.);
#9720=VECTOR('',#34169,10.);
#9721=VECTOR('',#34170,10.);
#9722=VECTOR('',#34171,10.);
#9723=VECTOR('',#34174,10.);
#9724=VECTOR('',#34175,10.);
#9725=VECTOR('',#34182,10.);
#9726=VECTOR('',#34183,10.);
#9727=VECTOR('',#34184,10.);
#9728=VECTOR('',#34187,10.);
#9729=VECTOR('',#34188,10.);
#9730=VECTOR('',#34195,10.);
#9731=VECTOR('',#34196,10.);
#9732=VECTOR('',#34197,10.);
#9733=VECTOR('',#34200,10.);
#9734=VECTOR('',#34201,10.);
#9735=VECTOR('',#34208,10.);
#9736=VECTOR('',#34209,10.);
#9737=VECTOR('',#34210,10.);
#9738=VECTOR('',#34213,10.);
#9739=VECTOR('',#34214,10.);
#9740=VECTOR('',#34221,10.);
#9741=VECTOR('',#34222,10.);
#9742=VECTOR('',#34223,10.);
#9743=VECTOR('',#34226,10.);
#9744=VECTOR('',#34227,10.);
#9745=VECTOR('',#34234,10.);
#9746=VECTOR('',#34235,10.);
#9747=VECTOR('',#34236,10.);
#9748=VECTOR('',#34239,10.);
#9749=VECTOR('',#34240,9.99999999999999);
#9750=VECTOR('',#34247,10.);
#9751=VECTOR('',#34248,10.);
#9752=VECTOR('',#34249,10.);
#9753=VECTOR('',#34252,10.);
#9754=VECTOR('',#34253,10.);
#9755=VECTOR('',#34260,10.);
#9756=VECTOR('',#34261,10.);
#9757=VECTOR('',#34262,10.);
#9758=VECTOR('',#34265,10.);
#9759=VECTOR('',#34266,10.);
#9760=VECTOR('',#34273,10.);
#9761=VECTOR('',#34274,9.99999999999999);
#9762=VECTOR('',#34275,10.);
#9763=VECTOR('',#34278,10.);
#9764=VECTOR('',#34279,10.);
#9765=VECTOR('',#34286,10.);
#9766=VECTOR('',#34287,10.);
#9767=VECTOR('',#34288,10.);
#9768=VECTOR('',#34291,10.);
#9769=VECTOR('',#34292,10.);
#9770=VECTOR('',#34299,10.);
#9771=VECTOR('',#34300,10.);
#9772=VECTOR('',#34301,10.);
#9773=VECTOR('',#34304,10.);
#9774=VECTOR('',#34305,10.);
#9775=VECTOR('',#34312,10.);
#9776=VECTOR('',#34313,10.);
#9777=VECTOR('',#34314,10.);
#9778=VECTOR('',#34317,10.);
#9779=VECTOR('',#34318,10.);
#9780=VECTOR('',#34325,10.);
#9781=VECTOR('',#34326,10.);
#9782=VECTOR('',#34327,10.);
#9783=VECTOR('',#34330,10.);
#9784=VECTOR('',#34331,10.);
#9785=VECTOR('',#34338,10.);
#9786=VECTOR('',#34339,10.);
#9787=VECTOR('',#34340,10.);
#9788=VECTOR('',#34343,10.);
#9789=VECTOR('',#34344,10.);
#9790=VECTOR('',#34351,10.);
#9791=VECTOR('',#34352,10.);
#9792=VECTOR('',#34353,10.);
#9793=VECTOR('',#34356,10.);
#9794=VECTOR('',#34357,9.99999999999999);
#9795=VECTOR('',#34364,10.);
#9796=VECTOR('',#34365,10.);
#9797=VECTOR('',#34366,10.);
#9798=VECTOR('',#34369,10.);
#9799=VECTOR('',#34370,10.);
#9800=VECTOR('',#34377,10.);
#9801=VECTOR('',#34378,10.);
#9802=VECTOR('',#34379,10.);
#9803=VECTOR('',#34382,10.);
#9804=VECTOR('',#34383,10.);
#9805=VECTOR('',#34390,10.);
#9806=VECTOR('',#34391,9.99999999999999);
#9807=VECTOR('',#34392,10.);
#9808=VECTOR('',#34395,10.);
#9809=VECTOR('',#34396,10.);
#9810=VECTOR('',#34403,10.);
#9811=VECTOR('',#34404,10.);
#9812=VECTOR('',#34405,10.);
#9813=VECTOR('',#34408,10.);
#9814=VECTOR('',#34409,10.);
#9815=VECTOR('',#34416,10.);
#9816=VECTOR('',#34417,10.);
#9817=VECTOR('',#34418,10.);
#9818=VECTOR('',#34421,10.);
#9819=VECTOR('',#34422,10.);
#9820=VECTOR('',#34429,10.);
#9821=VECTOR('',#34430,10.);
#9822=VECTOR('',#34431,10.);
#9823=VECTOR('',#34434,10.);
#9824=VECTOR('',#34435,10.);
#9825=VECTOR('',#34442,2.8702);
#9826=VECTOR('',#34445,10.);
#9827=VECTOR('',#34446,10.);
#9828=VECTOR('',#34447,10.);
#9829=VECTOR('',#34448,10.);
#9830=VECTOR('',#34449,10.);
#9831=VECTOR('',#34450,10.);
#9832=VECTOR('',#34453,10.);
#9833=VECTOR('',#34458,10.);
#9834=VECTOR('',#34463,10.);
#9835=VECTOR('',#34468,10.);
#9836=VECTOR('',#34473,10.);
#9837=VECTOR('',#34478,10.);
#9838=VECTOR('',#34483,0.801975608296219);
#9839=VECTOR('',#34486,10.);
#9840=VECTOR('',#34487,10.);
#9841=VECTOR('',#34490,10.);
#9842=VECTOR('',#34493,10.);
#9843=VECTOR('',#34496,10.);
#9844=VECTOR('',#34499,10.);
#10760=CIRCLE('',#28463,1.27);
#10761=CIRCLE('',#28471,1.70434);
#10762=CIRCLE('',#28472,1.70434);
#10763=CIRCLE('',#28474,1.27);
#10764=CIRCLE('',#28476,1.70434);
#10765=CIRCLE('',#28477,1.70434);
#10766=CIRCLE('',#28479,1.70434);
#10767=CIRCLE('',#28480,1.70434);
#10768=CIRCLE('',#28482,1.85434);
#10769=CIRCLE('',#28483,0.15);
#10770=CIRCLE('',#28485,2.8702);
#10771=CIRCLE('',#28487,1.35434);
#10772=CIRCLE('',#28492,2.8702);
#10773=CIRCLE('',#28494,2.8702);
#10774=CIRCLE('',#28495,2.8702);
#10775=CIRCLE('',#28496,2.8702);
#10776=CIRCLE('',#28497,2.8702);
#10777=CIRCLE('',#28498,2.8702);
#10778=CIRCLE('',#28499,2.8702);
#10779=CIRCLE('',#28500,2.8702);
#10780=CIRCLE('',#28501,2.8702);
#10781=CIRCLE('',#28502,2.8702);
#10782=CIRCLE('',#28503,2.8702);
#10783=CIRCLE('',#28504,2.8702);
#10784=CIRCLE('',#28505,2.8702);
#10785=CIRCLE('',#28506,2.8702);
#10786=CIRCLE('',#28507,2.8702);
#10787=CIRCLE('',#28508,2.8702);
#10788=CIRCLE('',#28509,2.8702);
#10789=CIRCLE('',#28510,2.8702);
#10790=CIRCLE('',#28511,2.8702);
#10791=CIRCLE('',#28512,2.8702);
#10792=CIRCLE('',#28513,2.8702);
#10793=CIRCLE('',#28514,2.8702);
#10794=CIRCLE('',#28515,2.8702);
#10795=CIRCLE('',#28516,2.8702);
#10796=CIRCLE('',#28517,2.8702);
#10797=CIRCLE('',#28518,2.8702);
#10798=CIRCLE('',#28519,2.8702);
#10799=CIRCLE('',#28520,2.8702);
#10800=CIRCLE('',#28521,2.8702);
#10801=CIRCLE('',#28522,2.8702);
#10802=CIRCLE('',#28523,2.8702);
#10803=CIRCLE('',#28524,2.8702);
#10804=CIRCLE('',#28525,2.8702);
#10805=CIRCLE('',#28526,2.8702);
#10806=CIRCLE('',#28527,2.8702);
#10807=CIRCLE('',#28528,2.8702);
#10808=CIRCLE('',#28529,2.8702);
#10809=CIRCLE('',#28530,2.5702);
#10810=CIRCLE('',#28534,2.8702);
#10811=CIRCLE('',#28538,2.8702);
#10812=CIRCLE('',#28542,2.8702);
#10813=CIRCLE('',#28546,2.8702);
#10814=CIRCLE('',#28550,2.8702);
#10815=CIRCLE('',#28554,2.8702);
#10816=CIRCLE('',#28558,2.8702);
#10817=CIRCLE('',#28562,2.8702);
#10818=CIRCLE('',#28563,2.8702);
#10819=CIRCLE('',#28567,2.8702);
#10820=CIRCLE('',#28571,2.8702);
#10821=CIRCLE('',#28575,2.8702);
#10822=CIRCLE('',#28579,2.8702);
#10823=CIRCLE('',#28583,2.8702);
#10824=CIRCLE('',#28587,2.8702);
#10825=CIRCLE('',#28591,2.8702);
#10826=CIRCLE('',#28595,2.8702);
#10827=CIRCLE('',#28599,2.8702);
#10828=CIRCLE('',#28603,2.8702);
#10829=CIRCLE('',#28607,2.8702);
#10830=CIRCLE('',#28611,2.8702);
#10831=CIRCLE('',#28615,2.8702);
#10832=CIRCLE('',#28619,2.8702);
#10833=CIRCLE('',#28623,2.8702);
#10834=CIRCLE('',#28627,2.8702);
#10835=CIRCLE('',#28631,2.8702);
#10836=CIRCLE('',#28635,2.8702);
#10837=CIRCLE('',#28639,2.8702);
#10838=CIRCLE('',#28643,2.8702);
#10839=CIRCLE('',#28647,2.8702);
#10840=CIRCLE('',#28651,2.8702);
#10841=CIRCLE('',#28655,2.8702);
#10842=CIRCLE('',#28659,2.8702);
#10843=CIRCLE('',#28663,2.8702);
#10844=CIRCLE('',#28667,2.8702);
#10845=CIRCLE('',#28671,2.8702);
#10846=CIRCLE('',#28675,1.60395121659243);
#10847=CIRCLE('',#28677,1.60395121659243);
#10848=CIRCLE('',#28679,1.60395121659243);
#10849=CIRCLE('',#28681,1.60395121659243);
#10850=CIRCLE('',#28683,1.60395121659243);
#10851=CIRCLE('',#28685,1.60395121659243);
#12699=VERTEX_POINT('',#53159);
#12700=VERTEX_POINT('',#53160);
#12701=VERTEX_POINT('',#53162);
#12702=VERTEX_POINT('',#53269);
#12703=VERTEX_POINT('',#53346);
#12704=VERTEX_POINT('',#53347);
#12705=VERTEX_POINT('',#53644);
#12706=VERTEX_POINT('',#53645);
#12707=VERTEX_POINT('',#53647);
#12708=VERTEX_POINT('',#53796);
#12709=VERTEX_POINT('',#53944);
#12710=VERTEX_POINT('',#53945);
#12711=VERTEX_POINT('',#54234);
#12712=VERTEX_POINT('',#54235);
#12713=VERTEX_POINT('',#54237);
#12714=VERTEX_POINT('',#54382);
#12715=VERTEX_POINT('',#54532);
#12716=VERTEX_POINT('',#54533);
#12717=VERTEX_POINT('',#54824);
#12718=VERTEX_POINT('',#54825);
#12719=VERTEX_POINT('',#54827);
#12720=VERTEX_POINT('',#54970);
#12721=VERTEX_POINT('',#55114);
#12722=VERTEX_POINT('',#55115);
#12723=VERTEX_POINT('',#55174);
#12724=VERTEX_POINT('',#55176);
#12725=VERTEX_POINT('',#55182);
#12726=VERTEX_POINT('',#55358);
#12727=VERTEX_POINT('',#55534);
#12728=VERTEX_POINT('',#55707);
#12729=VERTEX_POINT('',#55883);
#12730=VERTEX_POINT('',#56059);
#12731=VERTEX_POINT('',#56235);
#12732=VERTEX_POINT('',#56411);
#12733=VERTEX_POINT('',#56446);
#12734=VERTEX_POINT('',#56448);
#12735=VERTEX_POINT('',#56456);
#12736=VERTEX_POINT('',#56467);
#12737=VERTEX_POINT('',#56643);
#12738=VERTEX_POINT('',#56819);
#12739=VERTEX_POINT('',#56995);
#12740=VERTEX_POINT('',#57168);
#12741=VERTEX_POINT('',#57520);
#12742=VERTEX_POINT('',#57649);
#12743=VERTEX_POINT('',#57748);
#12744=VERTEX_POINT('',#57749);
#12745=VERTEX_POINT('',#57830);
#12746=VERTEX_POINT('',#58133);
#12747=VERTEX_POINT('',#58224);
#12748=VERTEX_POINT('',#58225);
#12749=VERTEX_POINT('',#58520);
#12750=VERTEX_POINT('',#58524);
#12751=VERTEX_POINT('',#58527);
#12752=VERTEX_POINT('',#58532);
#12753=VERTEX_POINT('',#58533);
#12754=VERTEX_POINT('',#58535);
#12755=VERTEX_POINT('',#58537);
#12756=VERTEX_POINT('',#58543);
#12757=VERTEX_POINT('',#58544);
#12758=VERTEX_POINT('',#58553);
#12759=VERTEX_POINT('',#58554);
#12760=VERTEX_POINT('',#58558);
#12761=VERTEX_POINT('',#58560);
#12762=VERTEX_POINT('',#58564);
#12763=VERTEX_POINT('',#58568);
#12764=VERTEX_POINT('',#58570);
#12765=VERTEX_POINT('',#58574);
#12766=VERTEX_POINT('',#58578);
#12767=VERTEX_POINT('',#58580);
#12768=VERTEX_POINT('',#58584);
#12769=VERTEX_POINT('',#58588);
#12770=VERTEX_POINT('',#58590);
#12771=VERTEX_POINT('',#58594);
#12772=VERTEX_POINT('',#58598);
#12773=VERTEX_POINT('',#58600);
#12774=VERTEX_POINT('',#58604);
#12775=VERTEX_POINT('',#58608);
#12776=VERTEX_POINT('',#58610);
#12777=VERTEX_POINT('',#58614);
#12778=VERTEX_POINT('',#58618);
#12779=VERTEX_POINT('',#58620);
#12780=VERTEX_POINT('',#58624);
#12781=VERTEX_POINT('',#58628);
#12782=VERTEX_POINT('',#58630);
#12783=VERTEX_POINT('',#58634);
#12784=VERTEX_POINT('',#58638);
#12785=VERTEX_POINT('',#58640);
#12786=VERTEX_POINT('',#58644);
#12787=VERTEX_POINT('',#58648);
#12788=VERTEX_POINT('',#58650);
#12789=VERTEX_POINT('',#58654);
#12790=VERTEX_POINT('',#58658);
#12791=VERTEX_POINT('',#58660);
#12792=VERTEX_POINT('',#58664);
#12793=VERTEX_POINT('',#58668);
#12794=VERTEX_POINT('',#58670);
#12795=VERTEX_POINT('',#58674);
#12796=VERTEX_POINT('',#58678);
#12797=VERTEX_POINT('',#58680);
#12798=VERTEX_POINT('',#58684);
#12799=VERTEX_POINT('',#58688);
#12800=VERTEX_POINT('',#58690);
#12801=VERTEX_POINT('',#58694);
#12802=VERTEX_POINT('',#58698);
#12803=VERTEX_POINT('',#58700);
#12804=VERTEX_POINT('',#58704);
#12805=VERTEX_POINT('',#58708);
#12806=VERTEX_POINT('',#58710);
#12807=VERTEX_POINT('',#58714);
#12808=VERTEX_POINT('',#58718);
#12809=VERTEX_POINT('',#58720);
#12810=VERTEX_POINT('',#58724);
#12811=VERTEX_POINT('',#58728);
#12812=VERTEX_POINT('',#58730);
#12813=VERTEX_POINT('',#58734);
#12814=VERTEX_POINT('',#58738);
#12815=VERTEX_POINT('',#58740);
#12816=VERTEX_POINT('',#58744);
#12817=VERTEX_POINT('',#58748);
#12818=VERTEX_POINT('',#58750);
#12819=VERTEX_POINT('',#58754);
#12820=VERTEX_POINT('',#58758);
#12821=VERTEX_POINT('',#58760);
#12822=VERTEX_POINT('',#58764);
#12823=VERTEX_POINT('',#58768);
#12824=VERTEX_POINT('',#58770);
#12825=VERTEX_POINT('',#58774);
#12826=VERTEX_POINT('',#58778);
#12827=VERTEX_POINT('',#58780);
#12828=VERTEX_POINT('',#58784);
#12829=VERTEX_POINT('',#58788);
#12830=VERTEX_POINT('',#58790);
#12831=VERTEX_POINT('',#58794);
#12832=VERTEX_POINT('',#58798);
#12833=VERTEX_POINT('',#58800);
#12834=VERTEX_POINT('',#58804);
#12835=VERTEX_POINT('',#58808);
#12836=VERTEX_POINT('',#58810);
#12837=VERTEX_POINT('',#58814);
#12838=VERTEX_POINT('',#58818);
#12839=VERTEX_POINT('',#58820);
#12840=VERTEX_POINT('',#58824);
#12841=VERTEX_POINT('',#58829);
#12842=VERTEX_POINT('',#58831);
#12843=VERTEX_POINT('',#58835);
#12844=VERTEX_POINT('',#58839);
#12845=VERTEX_POINT('',#58841);
#12846=VERTEX_POINT('',#58845);
#12847=VERTEX_POINT('',#58849);
#12848=VERTEX_POINT('',#58851);
#12849=VERTEX_POINT('',#58855);
#12850=VERTEX_POINT('',#58859);
#12851=VERTEX_POINT('',#58861);
#12852=VERTEX_POINT('',#58865);
#12853=VERTEX_POINT('',#58869);
#12854=VERTEX_POINT('',#58871);
#12855=VERTEX_POINT('',#58875);
#12856=VERTEX_POINT('',#58879);
#12857=VERTEX_POINT('',#58881);
#12858=VERTEX_POINT('',#58885);
#12859=VERTEX_POINT('',#58889);
#12860=VERTEX_POINT('',#58891);
#12861=VERTEX_POINT('',#58895);
#12862=VERTEX_POINT('',#58899);
#12863=VERTEX_POINT('',#58904);
#12864=VERTEX_POINT('',#58908);
#12865=VERTEX_POINT('',#58910);
#12866=VERTEX_POINT('',#58914);
#12867=VERTEX_POINT('',#58920);
#12868=VERTEX_POINT('',#58922);
#12869=VERTEX_POINT('',#58926);
#12870=VERTEX_POINT('',#58932);
#12871=VERTEX_POINT('',#58934);
#12872=VERTEX_POINT('',#58938);
#12873=VERTEX_POINT('',#58944);
#12874=VERTEX_POINT('',#58946);
#12875=VERTEX_POINT('',#58950);
#12876=VERTEX_POINT('',#58956);
#12877=VERTEX_POINT('',#58958);
#12878=VERTEX_POINT('',#58962);
#12879=VERTEX_POINT('',#58968);
#12880=VERTEX_POINT('',#58970);
#12881=VERTEX_POINT('',#58974);
#12882=VERTEX_POINT('',#58980);
#12883=VERTEX_POINT('',#58982);
#12884=VERTEX_POINT('',#58986);
#12885=VERTEX_POINT('',#58992);
#12886=VERTEX_POINT('',#58994);
#12887=VERTEX_POINT('',#58998);
#12888=VERTEX_POINT('',#59002);
#12889=VERTEX_POINT('',#59006);
#12890=VERTEX_POINT('',#59008);
#12891=VERTEX_POINT('',#59012);
#12892=VERTEX_POINT('',#59018);
#12893=VERTEX_POINT('',#59020);
#12894=VERTEX_POINT('',#59024);
#12895=VERTEX_POINT('',#59030);
#12896=VERTEX_POINT('',#59032);
#12897=VERTEX_POINT('',#59036);
#12898=VERTEX_POINT('',#59042);
#12899=VERTEX_POINT('',#59044);
#12900=VERTEX_POINT('',#59048);
#12901=VERTEX_POINT('',#59054);
#12902=VERTEX_POINT('',#59056);
#12903=VERTEX_POINT('',#59060);
#12904=VERTEX_POINT('',#59066);
#12905=VERTEX_POINT('',#59068);
#12906=VERTEX_POINT('',#59072);
#12907=VERTEX_POINT('',#59078);
#12908=VERTEX_POINT('',#59080);
#12909=VERTEX_POINT('',#59084);
#12910=VERTEX_POINT('',#59090);
#12911=VERTEX_POINT('',#59092);
#12912=VERTEX_POINT('',#59096);
#12913=VERTEX_POINT('',#59102);
#12914=VERTEX_POINT('',#59104);
#12915=VERTEX_POINT('',#59108);
#12916=VERTEX_POINT('',#59114);
#12917=VERTEX_POINT('',#59116);
#12918=VERTEX_POINT('',#59120);
#12919=VERTEX_POINT('',#59126);
#12920=VERTEX_POINT('',#59128);
#12921=VERTEX_POINT('',#59132);
#12922=VERTEX_POINT('',#59138);
#12923=VERTEX_POINT('',#59140);
#12924=VERTEX_POINT('',#59144);
#12925=VERTEX_POINT('',#59150);
#12926=VERTEX_POINT('',#59152);
#12927=VERTEX_POINT('',#59156);
#12928=VERTEX_POINT('',#59162);
#12929=VERTEX_POINT('',#59164);
#12930=VERTEX_POINT('',#59168);
#12931=VERTEX_POINT('',#59174);
#12932=VERTEX_POINT('',#59176);
#12933=VERTEX_POINT('',#59180);
#12934=VERTEX_POINT('',#59186);
#12935=VERTEX_POINT('',#59188);
#12936=VERTEX_POINT('',#59192);
#12937=VERTEX_POINT('',#59198);
#12938=VERTEX_POINT('',#59200);
#12939=VERTEX_POINT('',#59204);
#12940=VERTEX_POINT('',#59210);
#12941=VERTEX_POINT('',#59212);
#12942=VERTEX_POINT('',#59216);
#12943=VERTEX_POINT('',#59222);
#12944=VERTEX_POINT('',#59224);
#12945=VERTEX_POINT('',#59228);
#12946=VERTEX_POINT('',#59234);
#12947=VERTEX_POINT('',#59236);
#12948=VERTEX_POINT('',#59240);
#12949=VERTEX_POINT('',#59246);
#12950=VERTEX_POINT('',#59248);
#12951=VERTEX_POINT('',#59252);
#12952=VERTEX_POINT('',#59258);
#12953=VERTEX_POINT('',#59260);
#12954=VERTEX_POINT('',#59264);
#12955=VERTEX_POINT('',#59270);
#12956=VERTEX_POINT('',#59272);
#12957=VERTEX_POINT('',#59276);
#12958=VERTEX_POINT('',#59282);
#12959=VERTEX_POINT('',#59284);
#12960=VERTEX_POINT('',#59288);
#12961=VERTEX_POINT('',#59294);
#12962=VERTEX_POINT('',#59296);
#12963=VERTEX_POINT('',#59300);
#12964=VERTEX_POINT('',#59306);
#12965=VERTEX_POINT('',#59308);
#12966=VERTEX_POINT('',#59312);
#12967=VERTEX_POINT('',#59318);
#12968=VERTEX_POINT('',#59320);
#12969=VERTEX_POINT('',#59324);
#12970=VERTEX_POINT('',#59332);
#12971=VERTEX_POINT('',#59333);
#12972=VERTEX_POINT('',#59335);
#12973=VERTEX_POINT('',#59337);
#12974=VERTEX_POINT('',#59339);
#12975=VERTEX_POINT('',#59341);
#12976=VERTEX_POINT('',#59345);
#12977=VERTEX_POINT('',#59346);
#12978=VERTEX_POINT('',#59350);
#12979=VERTEX_POINT('',#59354);
#12980=VERTEX_POINT('',#59358);
#12981=VERTEX_POINT('',#59362);
#12982=VERTEX_POINT('',#59369);
#16190=EDGE_CURVE('',#12699,#12700,#7125,.T.);
#16191=EDGE_CURVE('',#12701,#12699,#645,.F.);
#16192=EDGE_CURVE('',#12702,#12701,#10760,.T.);
#16193=EDGE_CURVE('',#12702,#12700,#646,.T.);
#16194=EDGE_CURVE('',#12703,#12704,#7126,.T.);
#16195=EDGE_CURVE('',#12699,#12703,#647,.F.);
#16196=EDGE_CURVE('',#12700,#12704,#648,.T.);
#16197=EDGE_CURVE('',#12705,#12706,#7127,.T.);
#16198=EDGE_CURVE('',#12707,#12705,#649,.F.);
#16199=EDGE_CURVE('',#12703,#12707,#650,.F.);
#16200=EDGE_CURVE('',#12704,#12708,#651,.T.);
#16201=EDGE_CURVE('',#12708,#12706,#652,.T.);
#16202=EDGE_CURVE('',#12709,#12710,#7128,.T.);
#16203=EDGE_CURVE('',#12705,#12709,#653,.F.);
#16204=EDGE_CURVE('',#12706,#12710,#654,.T.);
#16205=EDGE_CURVE('',#12711,#12712,#7129,.T.);
#16206=EDGE_CURVE('',#12713,#12711,#655,.F.);
#16207=EDGE_CURVE('',#12709,#12713,#656,.F.);
#16208=EDGE_CURVE('',#12710,#12714,#657,.T.);
#16209=EDGE_CURVE('',#12714,#12712,#658,.T.);
#16210=EDGE_CURVE('',#12715,#12716,#7130,.T.);
#16211=EDGE_CURVE('',#12711,#12715,#659,.F.);
#16212=EDGE_CURVE('',#12712,#12716,#660,.T.);
#16213=EDGE_CURVE('',#12717,#12718,#7131,.T.);
#16214=EDGE_CURVE('',#12719,#12717,#661,.F.);
#16215=EDGE_CURVE('',#12715,#12719,#662,.F.);
#16216=EDGE_CURVE('',#12716,#12720,#663,.T.);
#16217=EDGE_CURVE('',#12720,#12718,#664,.F.);
#16218=EDGE_CURVE('',#12721,#12722,#665,.T.);
#16219=EDGE_CURVE('',#12723,#12722,#10761,.T.);
#16220=EDGE_CURVE('',#12723,#12724,#666,.T.);
#16221=EDGE_CURVE('',#12724,#12725,#667,.T.);
#16222=EDGE_CURVE('',#12725,#12726,#668,.T.);
#16223=EDGE_CURVE('',#12726,#12727,#669,.T.);
#16224=EDGE_CURVE('',#12727,#12728,#670,.T.);
#16225=EDGE_CURVE('',#12728,#12729,#671,.T.);
#16226=EDGE_CURVE('',#12729,#12730,#672,.T.);
#16227=EDGE_CURVE('',#12730,#12731,#673,.T.);
#16228=EDGE_CURVE('',#12731,#12732,#674,.T.);
#16229=EDGE_CURVE('',#12733,#12732,#10762,.T.);
#16230=EDGE_CURVE('',#12733,#12734,#675,.T.);
#16231=EDGE_CURVE('',#12734,#12735,#676,.T.);
#16232=EDGE_CURVE('',#12735,#12736,#677,.T.);
#16233=EDGE_CURVE('',#12736,#12737,#678,.T.);
#16234=EDGE_CURVE('',#12737,#12738,#679,.T.);
#16235=EDGE_CURVE('',#12738,#12739,#680,.T.);
#16236=EDGE_CURVE('',#12739,#12740,#681,.T.);
#16237=EDGE_CURVE('',#12740,#12721,#682,.T.);
#16238=EDGE_CURVE('',#12718,#12741,#683,.F.);
#16239=EDGE_CURVE('',#12742,#12741,#10763,.T.);
#16240=EDGE_CURVE('',#12717,#12742,#684,.F.);
#16241=EDGE_CURVE('',#12743,#12744,#10764,.T.);
#16242=EDGE_CURVE('',#12743,#12742,#685,.T.);
#16243=EDGE_CURVE('',#12741,#12745,#686,.T.);
#16244=EDGE_CURVE('',#12745,#12733,#687,.T.);
#16245=EDGE_CURVE('',#12744,#12733,#10765,.T.);
#16246=EDGE_CURVE('',#12732,#12743,#688,.T.);
#16247=EDGE_CURVE('',#12746,#12723,#689,.T.);
#16248=EDGE_CURVE('',#12746,#12701,#690,.T.);
#16249=EDGE_CURVE('',#12747,#12748,#10766,.T.);
#16250=EDGE_CURVE('',#12747,#12702,#691,.T.);
#16251=EDGE_CURVE('',#12748,#12723,#10767,.T.);
#16252=EDGE_CURVE('',#12722,#12747,#692,.T.);
#16253=EDGE_CURVE('',#12749,#12749,#10768,.T.);
#16254=EDGE_CURVE('',#12749,#12748,#10769,.T.);
#16255=EDGE_CURVE('',#12750,#12750,#10770,.T.);
#16256=EDGE_CURVE('',#12744,#12751,#7132,.T.);
#16257=EDGE_CURVE('',#12751,#12751,#10771,.T.);
#16258=EDGE_CURVE('',#12752,#12753,#7133,.T.);
#16259=EDGE_CURVE('',#12752,#12754,#7134,.T.);
#16260=EDGE_CURVE('',#12755,#12754,#7135,.T.);
#16261=EDGE_CURVE('',#12753,#12755,#281,.T.);
#16262=EDGE_CURVE('',#12756,#12757,#7136,.T.);
#16263=EDGE_CURVE('',#12755,#12756,#282,.T.);
#16264=EDGE_CURVE('',#12754,#12757,#7137,.T.);
#16265=EDGE_CURVE('',#12757,#12752,#10772,.T.);
#16266=EDGE_CURVE('',#12758,#12759,#283,.T.);
#16267=EDGE_CURVE('',#12759,#12760,#10773,.T.);
#16268=EDGE_CURVE('',#12760,#12761,#284,.T.);
#16269=EDGE_CURVE('',#12761,#12762,#285,.T.);
#16270=EDGE_CURVE('',#12762,#12763,#10774,.T.);
#16271=EDGE_CURVE('',#12763,#12764,#286,.T.);
#16272=EDGE_CURVE('',#12764,#12765,#287,.T.);
#16273=EDGE_CURVE('',#12765,#12766,#10775,.T.);
#16274=EDGE_CURVE('',#12766,#12767,#288,.T.);
#16275=EDGE_CURVE('',#12767,#12768,#289,.T.);
#16276=EDGE_CURVE('',#12768,#12769,#10776,.T.);
#16277=EDGE_CURVE('',#12769,#12770,#290,.T.);
#16278=EDGE_CURVE('',#12770,#12771,#291,.T.);
#16279=EDGE_CURVE('',#12771,#12772,#10777,.T.);
#16280=EDGE_CURVE('',#12772,#12773,#292,.T.);
#16281=EDGE_CURVE('',#12773,#12774,#293,.T.);
#16282=EDGE_CURVE('',#12774,#12775,#10778,.T.);
#16283=EDGE_CURVE('',#12775,#12776,#294,.T.);
#16284=EDGE_CURVE('',#12776,#12777,#295,.T.);
#16285=EDGE_CURVE('',#12777,#12778,#10779,.T.);
#16286=EDGE_CURVE('',#12778,#12779,#296,.T.);
#16287=EDGE_CURVE('',#12779,#12780,#297,.T.);
#16288=EDGE_CURVE('',#12780,#12781,#10780,.T.);
#16289=EDGE_CURVE('',#12781,#12782,#298,.T.);
#16290=EDGE_CURVE('',#12782,#12783,#299,.T.);
#16291=EDGE_CURVE('',#12783,#12784,#10781,.T.);
#16292=EDGE_CURVE('',#12784,#12785,#300,.T.);
#16293=EDGE_CURVE('',#12785,#12786,#301,.T.);
#16294=EDGE_CURVE('',#12786,#12787,#10782,.T.);
#16295=EDGE_CURVE('',#12787,#12788,#302,.T.);
#16296=EDGE_CURVE('',#12788,#12789,#303,.T.);
#16297=EDGE_CURVE('',#12789,#12790,#10783,.T.);
#16298=EDGE_CURVE('',#12790,#12791,#304,.T.);
#16299=EDGE_CURVE('',#12791,#12792,#305,.T.);
#16300=EDGE_CURVE('',#12792,#12793,#10784,.T.);
#16301=EDGE_CURVE('',#12793,#12794,#306,.T.);
#16302=EDGE_CURVE('',#12794,#12795,#307,.T.);
#16303=EDGE_CURVE('',#12795,#12796,#10785,.T.);
#16304=EDGE_CURVE('',#12796,#12797,#308,.T.);
#16305=EDGE_CURVE('',#12797,#12798,#309,.T.);
#16306=EDGE_CURVE('',#12798,#12799,#10786,.T.);
#16307=EDGE_CURVE('',#12799,#12800,#310,.T.);
#16308=EDGE_CURVE('',#12800,#12801,#311,.T.);
#16309=EDGE_CURVE('',#12801,#12802,#10787,.T.);
#16310=EDGE_CURVE('',#12802,#12803,#312,.T.);
#16311=EDGE_CURVE('',#12803,#12804,#313,.T.);
#16312=EDGE_CURVE('',#12804,#12805,#10788,.T.);
#16313=EDGE_CURVE('',#12805,#12806,#314,.T.);
#16314=EDGE_CURVE('',#12806,#12807,#315,.T.);
#16315=EDGE_CURVE('',#12807,#12808,#10789,.T.);
#16316=EDGE_CURVE('',#12808,#12809,#316,.T.);
#16317=EDGE_CURVE('',#12809,#12810,#317,.T.);
#16318=EDGE_CURVE('',#12810,#12811,#10790,.T.);
#16319=EDGE_CURVE('',#12811,#12812,#318,.T.);
#16320=EDGE_CURVE('',#12812,#12813,#319,.T.);
#16321=EDGE_CURVE('',#12813,#12814,#10791,.T.);
#16322=EDGE_CURVE('',#12814,#12815,#320,.T.);
#16323=EDGE_CURVE('',#12815,#12816,#321,.T.);
#16324=EDGE_CURVE('',#12816,#12817,#10792,.T.);
#16325=EDGE_CURVE('',#12817,#12818,#322,.T.);
#16326=EDGE_CURVE('',#12818,#12819,#323,.T.);
#16327=EDGE_CURVE('',#12819,#12820,#10793,.T.);
#16328=EDGE_CURVE('',#12820,#12821,#324,.T.);
#16329=EDGE_CURVE('',#12821,#12822,#325,.T.);
#16330=EDGE_CURVE('',#12822,#12823,#10794,.T.);
#16331=EDGE_CURVE('',#12823,#12824,#326,.T.);
#16332=EDGE_CURVE('',#12824,#12825,#327,.T.);
#16333=EDGE_CURVE('',#12825,#12826,#10795,.T.);
#16334=EDGE_CURVE('',#12826,#12827,#328,.T.);
#16335=EDGE_CURVE('',#12827,#12828,#329,.T.);
#16336=EDGE_CURVE('',#12828,#12829,#10796,.T.);
#16337=EDGE_CURVE('',#12829,#12830,#330,.T.);
#16338=EDGE_CURVE('',#12830,#12831,#331,.T.);
#16339=EDGE_CURVE('',#12831,#12832,#10797,.T.);
#16340=EDGE_CURVE('',#12832,#12833,#332,.T.);
#16341=EDGE_CURVE('',#12833,#12834,#333,.T.);
#16342=EDGE_CURVE('',#12834,#12835,#10798,.T.);
#16343=EDGE_CURVE('',#12835,#12836,#334,.T.);
#16344=EDGE_CURVE('',#12836,#12837,#335,.T.);
#16345=EDGE_CURVE('',#12837,#12838,#10799,.T.);
#16346=EDGE_CURVE('',#12838,#12839,#336,.T.);
#16347=EDGE_CURVE('',#12839,#12840,#337,.T.);
#16348=EDGE_CURVE('',#12840,#12753,#10800,.T.);
#16349=EDGE_CURVE('',#12756,#12841,#10801,.T.);
#16350=EDGE_CURVE('',#12841,#12842,#338,.T.);
#16351=EDGE_CURVE('',#12842,#12843,#339,.T.);
#16352=EDGE_CURVE('',#12843,#12844,#10802,.T.);
#16353=EDGE_CURVE('',#12844,#12845,#340,.T.);
#16354=EDGE_CURVE('',#12845,#12846,#341,.T.);
#16355=EDGE_CURVE('',#12846,#12847,#10803,.T.);
#16356=EDGE_CURVE('',#12847,#12848,#342,.T.);
#16357=EDGE_CURVE('',#12848,#12849,#343,.T.);
#16358=EDGE_CURVE('',#12849,#12850,#10804,.T.);
#16359=EDGE_CURVE('',#12850,#12851,#344,.T.);
#16360=EDGE_CURVE('',#12851,#12852,#345,.T.);
#16361=EDGE_CURVE('',#12852,#12853,#10805,.T.);
#16362=EDGE_CURVE('',#12853,#12854,#346,.T.);
#16363=EDGE_CURVE('',#12854,#12855,#347,.T.);
#16364=EDGE_CURVE('',#12855,#12856,#10806,.T.);
#16365=EDGE_CURVE('',#12856,#12857,#348,.T.);
#16366=EDGE_CURVE('',#12857,#12858,#349,.T.);
#16367=EDGE_CURVE('',#12858,#12859,#10807,.T.);
#16368=EDGE_CURVE('',#12859,#12860,#350,.T.);
#16369=EDGE_CURVE('',#12860,#12861,#351,.T.);
#16370=EDGE_CURVE('',#12861,#12862,#10808,.T.);
#16371=EDGE_CURVE('',#12862,#12758,#352,.T.);
#16372=EDGE_CURVE('',#12758,#12863,#7138,.T.);
#16373=EDGE_CURVE('',#12863,#12863,#10809,.T.);
#16374=EDGE_CURVE('',#12864,#12841,#7139,.T.);
#16375=EDGE_CURVE('',#12864,#12865,#7140,.T.);
#16376=EDGE_CURVE('',#12842,#12865,#7141,.T.);
#16377=EDGE_CURVE('',#12843,#12866,#7142,.T.);
#16378=EDGE_CURVE('',#12865,#12866,#7143,.T.);
#16379=EDGE_CURVE('',#12866,#12864,#10810,.T.);
#16380=EDGE_CURVE('',#12867,#12844,#7144,.T.);
#16381=EDGE_CURVE('',#12867,#12868,#7145,.T.);
#16382=EDGE_CURVE('',#12845,#12868,#7146,.T.);
#16383=EDGE_CURVE('',#12846,#12869,#7147,.T.);
#16384=EDGE_CURVE('',#12868,#12869,#7148,.T.);
#16385=EDGE_CURVE('',#12869,#12867,#10811,.T.);
#16386=EDGE_CURVE('',#12870,#12847,#7149,.T.);
#16387=EDGE_CURVE('',#12870,#12871,#7150,.T.);
#16388=EDGE_CURVE('',#12848,#12871,#7151,.T.);
#16389=EDGE_CURVE('',#12849,#12872,#7152,.T.);
#16390=EDGE_CURVE('',#12871,#12872,#7153,.T.);
#16391=EDGE_CURVE('',#12872,#12870,#10812,.T.);
#16392=EDGE_CURVE('',#12873,#12850,#7154,.T.);
#16393=EDGE_CURVE('',#12873,#12874,#7155,.T.);
#16394=EDGE_CURVE('',#12851,#12874,#7156,.T.);
#16395=EDGE_CURVE('',#12852,#12875,#7157,.T.);
#16396=EDGE_CURVE('',#12874,#12875,#7158,.T.);
#16397=EDGE_CURVE('',#12875,#12873,#10813,.T.);
#16398=EDGE_CURVE('',#12876,#12853,#7159,.T.);
#16399=EDGE_CURVE('',#12876,#12877,#7160,.T.);
#16400=EDGE_CURVE('',#12854,#12877,#7161,.T.);
#16401=EDGE_CURVE('',#12855,#12878,#7162,.T.);
#16402=EDGE_CURVE('',#12877,#12878,#7163,.T.);
#16403=EDGE_CURVE('',#12878,#12876,#10814,.T.);
#16404=EDGE_CURVE('',#12879,#12856,#7164,.T.);
#16405=EDGE_CURVE('',#12879,#12880,#7165,.T.);
#16406=EDGE_CURVE('',#12857,#12880,#7166,.T.);
#16407=EDGE_CURVE('',#12858,#12881,#7167,.T.);
#16408=EDGE_CURVE('',#12880,#12881,#7168,.T.);
#16409=EDGE_CURVE('',#12881,#12879,#10815,.T.);
#16410=EDGE_CURVE('',#12882,#12859,#7169,.T.);
#16411=EDGE_CURVE('',#12882,#12883,#7170,.T.);
#16412=EDGE_CURVE('',#12860,#12883,#7171,.T.);
#16413=EDGE_CURVE('',#12861,#12884,#7172,.T.);
#16414=EDGE_CURVE('',#12883,#12884,#7173,.T.);
#16415=EDGE_CURVE('',#12884,#12882,#10816,.T.);
#16416=EDGE_CURVE('',#12885,#12862,#7174,.T.);
#16417=EDGE_CURVE('',#12885,#12886,#7175,.T.);
#16418=EDGE_CURVE('',#12758,#12886,#7176,.T.);
#16419=EDGE_CURVE('',#12759,#12887,#7177,.T.);
#16420=EDGE_CURVE('',#12886,#12887,#7178,.T.);
#16421=EDGE_CURVE('',#12887,#12888,#10817,.T.);
#16422=EDGE_CURVE('',#12888,#12885,#10818,.T.);
#16423=EDGE_CURVE('',#12889,#12760,#7179,.T.);
#16424=EDGE_CURVE('',#12889,#12890,#7180,.T.);
#16425=EDGE_CURVE('',#12761,#12890,#7181,.T.);
#16426=EDGE_CURVE('',#12762,#12891,#7182,.T.);
#16427=EDGE_CURVE('',#12890,#12891,#7183,.T.);
#16428=EDGE_CURVE('',#12891,#12889,#10819,.T.);
#16429=EDGE_CURVE('',#12892,#12763,#7184,.T.);
#16430=EDGE_CURVE('',#12892,#12893,#7185,.T.);
#16431=EDGE_CURVE('',#12764,#12893,#7186,.T.);
#16432=EDGE_CURVE('',#12765,#12894,#7187,.T.);
#16433=EDGE_CURVE('',#12893,#12894,#7188,.T.);
#16434=EDGE_CURVE('',#12894,#12892,#10820,.T.);
#16435=EDGE_CURVE('',#12895,#12766,#7189,.T.);
#16436=EDGE_CURVE('',#12895,#12896,#7190,.T.);
#16437=EDGE_CURVE('',#12767,#12896,#7191,.T.);
#16438=EDGE_CURVE('',#12768,#12897,#7192,.T.);
#16439=EDGE_CURVE('',#12896,#12897,#7193,.T.);
#16440=EDGE_CURVE('',#12897,#12895,#10821,.T.);
#16441=EDGE_CURVE('',#12898,#12769,#7194,.T.);
#16442=EDGE_CURVE('',#12898,#12899,#7195,.T.);
#16443=EDGE_CURVE('',#12770,#12899,#7196,.T.);
#16444=EDGE_CURVE('',#12771,#12900,#7197,.T.);
#16445=EDGE_CURVE('',#12899,#12900,#7198,.T.);
#16446=EDGE_CURVE('',#12900,#12898,#10822,.T.);
#16447=EDGE_CURVE('',#12901,#12772,#7199,.T.);
#16448=EDGE_CURVE('',#12901,#12902,#7200,.T.);
#16449=EDGE_CURVE('',#12773,#12902,#7201,.T.);
#16450=EDGE_CURVE('',#12774,#12903,#7202,.T.);
#16451=EDGE_CURVE('',#12902,#12903,#7203,.T.);
#16452=EDGE_CURVE('',#12903,#12901,#10823,.T.);
#16453=EDGE_CURVE('',#12904,#12775,#7204,.T.);
#16454=EDGE_CURVE('',#12904,#12905,#7205,.T.);
#16455=EDGE_CURVE('',#12776,#12905,#7206,.T.);
#16456=EDGE_CURVE('',#12777,#12906,#7207,.T.);
#16457=EDGE_CURVE('',#12905,#12906,#7208,.T.);
#16458=EDGE_CURVE('',#12906,#12904,#10824,.T.);
#16459=EDGE_CURVE('',#12907,#12778,#7209,.T.);
#16460=EDGE_CURVE('',#12907,#12908,#7210,.T.);
#16461=EDGE_CURVE('',#12779,#12908,#7211,.T.);
#16462=EDGE_CURVE('',#12780,#12909,#7212,.T.);
#16463=EDGE_CURVE('',#12908,#12909,#7213,.T.);
#16464=EDGE_CURVE('',#12909,#12907,#10825,.T.);
#16465=EDGE_CURVE('',#12910,#12781,#7214,.T.);
#16466=EDGE_CURVE('',#12910,#12911,#7215,.T.);
#16467=EDGE_CURVE('',#12782,#12911,#7216,.T.);
#16468=EDGE_CURVE('',#12783,#12912,#7217,.T.);
#16469=EDGE_CURVE('',#12911,#12912,#7218,.T.);
#16470=EDGE_CURVE('',#12912,#12910,#10826,.T.);
#16471=EDGE_CURVE('',#12913,#12784,#7219,.T.);
#16472=EDGE_CURVE('',#12913,#12914,#7220,.T.);
#16473=EDGE_CURVE('',#12785,#12914,#7221,.T.);
#16474=EDGE_CURVE('',#12786,#12915,#7222,.T.);
#16475=EDGE_CURVE('',#12914,#12915,#7223,.T.);
#16476=EDGE_CURVE('',#12915,#12913,#10827,.T.);
#16477=EDGE_CURVE('',#12916,#12787,#7224,.T.);
#16478=EDGE_CURVE('',#12916,#12917,#7225,.T.);
#16479=EDGE_CURVE('',#12788,#12917,#7226,.T.);
#16480=EDGE_CURVE('',#12789,#12918,#7227,.T.);
#16481=EDGE_CURVE('',#12917,#12918,#7228,.T.);
#16482=EDGE_CURVE('',#12918,#12916,#10828,.T.);
#16483=EDGE_CURVE('',#12919,#12790,#7229,.T.);
#16484=EDGE_CURVE('',#12919,#12920,#7230,.T.);
#16485=EDGE_CURVE('',#12791,#12920,#7231,.T.);
#16486=EDGE_CURVE('',#12792,#12921,#7232,.T.);
#16487=EDGE_CURVE('',#12920,#12921,#7233,.T.);
#16488=EDGE_CURVE('',#12921,#12919,#10829,.T.);
#16489=EDGE_CURVE('',#12922,#12793,#7234,.T.);
#16490=EDGE_CURVE('',#12922,#12923,#7235,.T.);
#16491=EDGE_CURVE('',#12794,#12923,#7236,.T.);
#16492=EDGE_CURVE('',#12795,#12924,#7237,.T.);
#16493=EDGE_CURVE('',#12923,#12924,#7238,.T.);
#16494=EDGE_CURVE('',#12924,#12922,#10830,.T.);
#16495=EDGE_CURVE('',#12925,#12796,#7239,.T.);
#16496=EDGE_CURVE('',#12925,#12926,#7240,.T.);
#16497=EDGE_CURVE('',#12797,#12926,#7241,.T.);
#16498=EDGE_CURVE('',#12798,#12927,#7242,.T.);
#16499=EDGE_CURVE('',#12926,#12927,#7243,.T.);
#16500=EDGE_CURVE('',#12927,#12925,#10831,.T.);
#16501=EDGE_CURVE('',#12928,#12799,#7244,.T.);
#16502=EDGE_CURVE('',#12928,#12929,#7245,.T.);
#16503=EDGE_CURVE('',#12800,#12929,#7246,.T.);
#16504=EDGE_CURVE('',#12801,#12930,#7247,.T.);
#16505=EDGE_CURVE('',#12929,#12930,#7248,.T.);
#16506=EDGE_CURVE('',#12930,#12928,#10832,.T.);
#16507=EDGE_CURVE('',#12931,#12802,#7249,.T.);
#16508=EDGE_CURVE('',#12931,#12932,#7250,.T.);
#16509=EDGE_CURVE('',#12803,#12932,#7251,.T.);
#16510=EDGE_CURVE('',#12804,#12933,#7252,.T.);
#16511=EDGE_CURVE('',#12932,#12933,#7253,.T.);
#16512=EDGE_CURVE('',#12933,#12931,#10833,.T.);
#16513=EDGE_CURVE('',#12934,#12805,#7254,.T.);
#16514=EDGE_CURVE('',#12934,#12935,#7255,.T.);
#16515=EDGE_CURVE('',#12806,#12935,#7256,.T.);
#16516=EDGE_CURVE('',#12807,#12936,#7257,.T.);
#16517=EDGE_CURVE('',#12935,#12936,#7258,.T.);
#16518=EDGE_CURVE('',#12936,#12934,#10834,.T.);
#16519=EDGE_CURVE('',#12937,#12808,#7259,.T.);
#16520=EDGE_CURVE('',#12937,#12938,#7260,.T.);
#16521=EDGE_CURVE('',#12809,#12938,#7261,.T.);
#16522=EDGE_CURVE('',#12810,#12939,#7262,.T.);
#16523=EDGE_CURVE('',#12938,#12939,#7263,.T.);
#16524=EDGE_CURVE('',#12939,#12937,#10835,.T.);
#16525=EDGE_CURVE('',#12940,#12811,#7264,.T.);
#16526=EDGE_CURVE('',#12940,#12941,#7265,.T.);
#16527=EDGE_CURVE('',#12812,#12941,#7266,.T.);
#16528=EDGE_CURVE('',#12813,#12942,#7267,.T.);
#16529=EDGE_CURVE('',#12941,#12942,#7268,.T.);
#16530=EDGE_CURVE('',#12942,#12940,#10836,.T.);
#16531=EDGE_CURVE('',#12943,#12814,#7269,.T.);
#16532=EDGE_CURVE('',#12943,#12944,#7270,.T.);
#16533=EDGE_CURVE('',#12815,#12944,#7271,.T.);
#16534=EDGE_CURVE('',#12816,#12945,#7272,.T.);
#16535=EDGE_CURVE('',#12944,#12945,#7273,.T.);
#16536=EDGE_CURVE('',#12945,#12943,#10837,.T.);
#16537=EDGE_CURVE('',#12946,#12817,#7274,.T.);
#16538=EDGE_CURVE('',#12946,#12947,#7275,.T.);
#16539=EDGE_CURVE('',#12818,#12947,#7276,.T.);
#16540=EDGE_CURVE('',#12819,#12948,#7277,.T.);
#16541=EDGE_CURVE('',#12947,#12948,#7278,.T.);
#16542=EDGE_CURVE('',#12948,#12946,#10838,.T.);
#16543=EDGE_CURVE('',#12949,#12820,#7279,.T.);
#16544=EDGE_CURVE('',#12949,#12950,#7280,.T.);
#16545=EDGE_CURVE('',#12821,#12950,#7281,.T.);
#16546=EDGE_CURVE('',#12822,#12951,#7282,.T.);
#16547=EDGE_CURVE('',#12950,#12951,#7283,.T.);
#16548=EDGE_CURVE('',#12951,#12949,#10839,.T.);
#16549=EDGE_CURVE('',#12952,#12823,#7284,.T.);
#16550=EDGE_CURVE('',#12952,#12953,#7285,.T.);
#16551=EDGE_CURVE('',#12824,#12953,#7286,.T.);
#16552=EDGE_CURVE('',#12825,#12954,#7287,.T.);
#16553=EDGE_CURVE('',#12953,#12954,#7288,.T.);
#16554=EDGE_CURVE('',#12954,#12952,#10840,.T.);
#16555=EDGE_CURVE('',#12955,#12826,#7289,.T.);
#16556=EDGE_CURVE('',#12955,#12956,#7290,.T.);
#16557=EDGE_CURVE('',#12827,#12956,#7291,.T.);
#16558=EDGE_CURVE('',#12828,#12957,#7292,.T.);
#16559=EDGE_CURVE('',#12956,#12957,#7293,.T.);
#16560=EDGE_CURVE('',#12957,#12955,#10841,.T.);
#16561=EDGE_CURVE('',#12958,#12829,#7294,.T.);
#16562=EDGE_CURVE('',#12958,#12959,#7295,.T.);
#16563=EDGE_CURVE('',#12830,#12959,#7296,.T.);
#16564=EDGE_CURVE('',#12831,#12960,#7297,.T.);
#16565=EDGE_CURVE('',#12959,#12960,#7298,.T.);
#16566=EDGE_CURVE('',#12960,#12958,#10842,.T.);
#16567=EDGE_CURVE('',#12961,#12832,#7299,.T.);
#16568=EDGE_CURVE('',#12961,#12962,#7300,.T.);
#16569=EDGE_CURVE('',#12833,#12962,#7301,.T.);
#16570=EDGE_CURVE('',#12834,#12963,#7302,.T.);
#16571=EDGE_CURVE('',#12962,#12963,#7303,.T.);
#16572=EDGE_CURVE('',#12963,#12961,#10843,.T.);
#16573=EDGE_CURVE('',#12964,#12835,#7304,.T.);
#16574=EDGE_CURVE('',#12964,#12965,#7305,.T.);
#16575=EDGE_CURVE('',#12836,#12965,#7306,.T.);
#16576=EDGE_CURVE('',#12837,#12966,#7307,.T.);
#16577=EDGE_CURVE('',#12965,#12966,#7308,.T.);
#16578=EDGE_CURVE('',#12966,#12964,#10844,.T.);
#16579=EDGE_CURVE('',#12967,#12838,#7309,.T.);
#16580=EDGE_CURVE('',#12967,#12968,#7310,.T.);
#16581=EDGE_CURVE('',#12839,#12968,#7311,.T.);
#16582=EDGE_CURVE('',#12840,#12969,#7312,.T.);
#16583=EDGE_CURVE('',#12968,#12969,#7313,.T.);
#16584=EDGE_CURVE('',#12969,#12967,#10845,.T.);
#16585=EDGE_CURVE('',#12888,#12750,#7314,.T.);
#16586=EDGE_CURVE('',#12970,#12971,#7315,.T.);
#16587=EDGE_CURVE('',#12971,#12972,#7316,.T.);
#16588=EDGE_CURVE('',#12972,#12973,#7317,.T.);
#16589=EDGE_CURVE('',#12973,#12974,#7318,.T.);
#16590=EDGE_CURVE('',#12974,#12975,#7319,.T.);
#16591=EDGE_CURVE('',#12975,#12970,#7320,.T.);
#16592=EDGE_CURVE('',#12976,#12977,#7321,.T.);
#16593=EDGE_CURVE('',#12977,#12976,#10846,.T.);
#16594=EDGE_CURVE('',#12977,#12978,#7322,.T.);
#16595=EDGE_CURVE('',#12978,#12977,#10847,.T.);
#16596=EDGE_CURVE('',#12978,#12979,#7323,.T.);
#16597=EDGE_CURVE('',#12979,#12978,#10848,.T.);
#16598=EDGE_CURVE('',#12979,#12980,#7324,.T.);
#16599=EDGE_CURVE('',#12980,#12979,#10849,.T.);
#16600=EDGE_CURVE('',#12980,#12981,#7325,.T.);
#16601=EDGE_CURVE('',#12981,#12980,#10850,.T.);
#16602=EDGE_CURVE('',#12981,#12976,#7326,.T.);
#16603=EDGE_CURVE('',#12976,#12981,#10851,.T.);
#16604=EDGE_CURVE('',#12982,#12980,#7327,.T.);
#16605=EDGE_CURVE('',#12970,#12976,#7328,.T.);
#16606=EDGE_CURVE('',#12971,#12977,#7329,.T.);
#16607=EDGE_CURVE('',#12975,#12981,#7330,.T.);
#16608=EDGE_CURVE('',#12974,#12980,#7331,.T.);
#16609=EDGE_CURVE('',#12973,#12979,#7332,.T.);
#16610=EDGE_CURVE('',#12972,#12978,#7333,.T.);
#22658=ORIENTED_EDGE('',*,*,#16190,.F.);
#22659=ORIENTED_EDGE('',*,*,#16191,.F.);
#22660=ORIENTED_EDGE('',*,*,#16192,.F.);
#22661=ORIENTED_EDGE('',*,*,#16193,.T.);
#22662=ORIENTED_EDGE('',*,*,#16194,.F.);
#22663=ORIENTED_EDGE('',*,*,#16195,.F.);
#22664=ORIENTED_EDGE('',*,*,#16190,.T.);
#22665=ORIENTED_EDGE('',*,*,#16196,.T.);
#22666=ORIENTED_EDGE('',*,*,#16197,.F.);
#22667=ORIENTED_EDGE('',*,*,#16198,.F.);
#22668=ORIENTED_EDGE('',*,*,#16199,.F.);
#22669=ORIENTED_EDGE('',*,*,#16194,.T.);
#22670=ORIENTED_EDGE('',*,*,#16200,.T.);
#22671=ORIENTED_EDGE('',*,*,#16201,.T.);
#22672=ORIENTED_EDGE('',*,*,#16202,.F.);
#22673=ORIENTED_EDGE('',*,*,#16203,.F.);
#22674=ORIENTED_EDGE('',*,*,#16197,.T.);
#22675=ORIENTED_EDGE('',*,*,#16204,.T.);
#22676=ORIENTED_EDGE('',*,*,#16205,.F.);
#22677=ORIENTED_EDGE('',*,*,#16206,.F.);
#22678=ORIENTED_EDGE('',*,*,#16207,.F.);
#22679=ORIENTED_EDGE('',*,*,#16202,.T.);
#22680=ORIENTED_EDGE('',*,*,#16208,.T.);
#22681=ORIENTED_EDGE('',*,*,#16209,.T.);
#22682=ORIENTED_EDGE('',*,*,#16210,.F.);
#22683=ORIENTED_EDGE('',*,*,#16211,.F.);
#22684=ORIENTED_EDGE('',*,*,#16205,.T.);
#22685=ORIENTED_EDGE('',*,*,#16212,.T.);
#22686=ORIENTED_EDGE('',*,*,#16213,.F.);
#22687=ORIENTED_EDGE('',*,*,#16214,.F.);
#22688=ORIENTED_EDGE('',*,*,#16215,.F.);
#22689=ORIENTED_EDGE('',*,*,#16210,.T.);
#22690=ORIENTED_EDGE('',*,*,#16216,.T.);
#22691=ORIENTED_EDGE('',*,*,#16217,.T.);
#22692=ORIENTED_EDGE('',*,*,#16218,.T.);
#22693=ORIENTED_EDGE('',*,*,#16219,.F.);
#22694=ORIENTED_EDGE('',*,*,#16220,.T.);
#22695=ORIENTED_EDGE('',*,*,#16221,.T.);
#22696=ORIENTED_EDGE('',*,*,#16222,.T.);
#22697=ORIENTED_EDGE('',*,*,#16223,.T.);
#22698=ORIENTED_EDGE('',*,*,#16224,.T.);
#22699=ORIENTED_EDGE('',*,*,#16225,.T.);
#22700=ORIENTED_EDGE('',*,*,#16226,.T.);
#22701=ORIENTED_EDGE('',*,*,#16227,.T.);
#22702=ORIENTED_EDGE('',*,*,#16228,.T.);
#22703=ORIENTED_EDGE('',*,*,#16229,.F.);
#22704=ORIENTED_EDGE('',*,*,#16230,.T.);
#22705=ORIENTED_EDGE('',*,*,#16231,.T.);
#22706=ORIENTED_EDGE('',*,*,#16232,.T.);
#22707=ORIENTED_EDGE('',*,*,#16233,.T.);
#22708=ORIENTED_EDGE('',*,*,#16234,.T.);
#22709=ORIENTED_EDGE('',*,*,#16235,.T.);
#22710=ORIENTED_EDGE('',*,*,#16236,.T.);
#22711=ORIENTED_EDGE('',*,*,#16237,.T.);
#22712=ORIENTED_EDGE('',*,*,#16213,.T.);
#22713=ORIENTED_EDGE('',*,*,#16238,.T.);
#22714=ORIENTED_EDGE('',*,*,#16239,.F.);
#22715=ORIENTED_EDGE('',*,*,#16240,.F.);
#22716=ORIENTED_EDGE('',*,*,#16241,.F.);
#22717=ORIENTED_EDGE('',*,*,#16242,.T.);
#22718=ORIENTED_EDGE('',*,*,#16239,.T.);
#22719=ORIENTED_EDGE('',*,*,#16243,.T.);
#22720=ORIENTED_EDGE('',*,*,#16244,.T.);
#22721=ORIENTED_EDGE('',*,*,#16245,.F.);
#22722=ORIENTED_EDGE('',*,*,#16242,.F.);
#22723=ORIENTED_EDGE('',*,*,#16246,.F.);
#22724=ORIENTED_EDGE('',*,*,#16228,.F.);
#22725=ORIENTED_EDGE('',*,*,#16227,.F.);
#22726=ORIENTED_EDGE('',*,*,#16226,.F.);
#22727=ORIENTED_EDGE('',*,*,#16225,.F.);
#22728=ORIENTED_EDGE('',*,*,#16224,.F.);
#22729=ORIENTED_EDGE('',*,*,#16223,.F.);
#22730=ORIENTED_EDGE('',*,*,#16222,.F.);
#22731=ORIENTED_EDGE('',*,*,#16221,.F.);
#22732=ORIENTED_EDGE('',*,*,#16220,.F.);
#22733=ORIENTED_EDGE('',*,*,#16247,.F.);
#22734=ORIENTED_EDGE('',*,*,#16248,.T.);
#22735=ORIENTED_EDGE('',*,*,#16191,.T.);
#22736=ORIENTED_EDGE('',*,*,#16195,.T.);
#22737=ORIENTED_EDGE('',*,*,#16199,.T.);
#22738=ORIENTED_EDGE('',*,*,#16198,.T.);
#22739=ORIENTED_EDGE('',*,*,#16203,.T.);
#22740=ORIENTED_EDGE('',*,*,#16207,.T.);
#22741=ORIENTED_EDGE('',*,*,#16206,.T.);
#22742=ORIENTED_EDGE('',*,*,#16211,.T.);
#22743=ORIENTED_EDGE('',*,*,#16215,.T.);
#22744=ORIENTED_EDGE('',*,*,#16214,.T.);
#22745=ORIENTED_EDGE('',*,*,#16240,.T.);
#22746=ORIENTED_EDGE('',*,*,#16249,.F.);
#22747=ORIENTED_EDGE('',*,*,#16250,.T.);
#22748=ORIENTED_EDGE('',*,*,#16192,.T.);
#22749=ORIENTED_EDGE('',*,*,#16248,.F.);
#22750=ORIENTED_EDGE('',*,*,#16247,.T.);
#22751=ORIENTED_EDGE('',*,*,#16251,.F.);
#22752=ORIENTED_EDGE('',*,*,#16244,.F.);
#22753=ORIENTED_EDGE('',*,*,#16243,.F.);
#22754=ORIENTED_EDGE('',*,*,#16238,.F.);
#22755=ORIENTED_EDGE('',*,*,#16217,.F.);
#22756=ORIENTED_EDGE('',*,*,#16216,.F.);
#22757=ORIENTED_EDGE('',*,*,#16212,.F.);
#22758=ORIENTED_EDGE('',*,*,#16209,.F.);
#22759=ORIENTED_EDGE('',*,*,#16208,.F.);
#22760=ORIENTED_EDGE('',*,*,#16204,.F.);
#22761=ORIENTED_EDGE('',*,*,#16201,.F.);
#22762=ORIENTED_EDGE('',*,*,#16200,.F.);
#22763=ORIENTED_EDGE('',*,*,#16196,.F.);
#22764=ORIENTED_EDGE('',*,*,#16193,.F.);
#22765=ORIENTED_EDGE('',*,*,#16250,.F.);
#22766=ORIENTED_EDGE('',*,*,#16252,.F.);
#22767=ORIENTED_EDGE('',*,*,#16218,.F.);
#22768=ORIENTED_EDGE('',*,*,#16237,.F.);
#22769=ORIENTED_EDGE('',*,*,#16236,.F.);
#22770=ORIENTED_EDGE('',*,*,#16235,.F.);
#22771=ORIENTED_EDGE('',*,*,#16234,.F.);
#22772=ORIENTED_EDGE('',*,*,#16233,.F.);
#22773=ORIENTED_EDGE('',*,*,#16232,.F.);
#22774=ORIENTED_EDGE('',*,*,#16231,.F.);
#22775=ORIENTED_EDGE('',*,*,#16230,.F.);
#22776=ORIENTED_EDGE('',*,*,#16253,.T.);
#22777=ORIENTED_EDGE('',*,*,#16254,.T.);
#22778=ORIENTED_EDGE('',*,*,#16251,.T.);
#22779=ORIENTED_EDGE('',*,*,#16219,.T.);
#22780=ORIENTED_EDGE('',*,*,#16252,.T.);
#22781=ORIENTED_EDGE('',*,*,#16249,.T.);
#22782=ORIENTED_EDGE('',*,*,#16254,.F.);
#22783=ORIENTED_EDGE('',*,*,#16255,.F.);
#22784=ORIENTED_EDGE('',*,*,#16253,.F.);
#22785=ORIENTED_EDGE('',*,*,#16241,.T.);
#22786=ORIENTED_EDGE('',*,*,#16256,.T.);
#22787=ORIENTED_EDGE('',*,*,#16257,.T.);
#22788=ORIENTED_EDGE('',*,*,#16256,.F.);
#22789=ORIENTED_EDGE('',*,*,#16245,.T.);
#22790=ORIENTED_EDGE('',*,*,#16229,.T.);
#22791=ORIENTED_EDGE('',*,*,#16246,.T.);
#22792=ORIENTED_EDGE('',*,*,#16257,.F.);
#22793=ORIENTED_EDGE('',*,*,#16258,.F.);
#22794=ORIENTED_EDGE('',*,*,#16259,.T.);
#22795=ORIENTED_EDGE('',*,*,#16260,.F.);
#22796=ORIENTED_EDGE('',*,*,#16261,.F.);
#22797=ORIENTED_EDGE('',*,*,#16262,.F.);
#22798=ORIENTED_EDGE('',*,*,#16263,.F.);
#22799=ORIENTED_EDGE('',*,*,#16260,.T.);
#22800=ORIENTED_EDGE('',*,*,#16264,.T.);
#22801=ORIENTED_EDGE('',*,*,#16265,.F.);
#22802=ORIENTED_EDGE('',*,*,#16264,.F.);
#22803=ORIENTED_EDGE('',*,*,#16259,.F.);
#22804=ORIENTED_EDGE('',*,*,#16266,.T.);
#22805=ORIENTED_EDGE('',*,*,#16267,.T.);
#22806=ORIENTED_EDGE('',*,*,#16268,.T.);
#22807=ORIENTED_EDGE('',*,*,#16269,.T.);
#22808=ORIENTED_EDGE('',*,*,#16270,.T.);
#22809=ORIENTED_EDGE('',*,*,#16271,.T.);
#22810=ORIENTED_EDGE('',*,*,#16272,.T.);
#22811=ORIENTED_EDGE('',*,*,#16273,.T.);
#22812=ORIENTED_EDGE('',*,*,#16274,.T.);
#22813=ORIENTED_EDGE('',*,*,#16275,.T.);
#22814=ORIENTED_EDGE('',*,*,#16276,.T.);
#22815=ORIENTED_EDGE('',*,*,#16277,.T.);
#22816=ORIENTED_EDGE('',*,*,#16278,.T.);
#22817=ORIENTED_EDGE('',*,*,#16279,.T.);
#22818=ORIENTED_EDGE('',*,*,#16280,.T.);
#22819=ORIENTED_EDGE('',*,*,#16281,.T.);
#22820=ORIENTED_EDGE('',*,*,#16282,.T.);
#22821=ORIENTED_EDGE('',*,*,#16283,.T.);
#22822=ORIENTED_EDGE('',*,*,#16284,.T.);
#22823=ORIENTED_EDGE('',*,*,#16285,.T.);
#22824=ORIENTED_EDGE('',*,*,#16286,.T.);
#22825=ORIENTED_EDGE('',*,*,#16287,.T.);
#22826=ORIENTED_EDGE('',*,*,#16288,.T.);
#22827=ORIENTED_EDGE('',*,*,#16289,.T.);
#22828=ORIENTED_EDGE('',*,*,#16290,.T.);
#22829=ORIENTED_EDGE('',*,*,#16291,.T.);
#22830=ORIENTED_EDGE('',*,*,#16292,.T.);
#22831=ORIENTED_EDGE('',*,*,#16293,.T.);
#22832=ORIENTED_EDGE('',*,*,#16294,.T.);
#22833=ORIENTED_EDGE('',*,*,#16295,.T.);
#22834=ORIENTED_EDGE('',*,*,#16296,.T.);
#22835=ORIENTED_EDGE('',*,*,#16297,.T.);
#22836=ORIENTED_EDGE('',*,*,#16298,.T.);
#22837=ORIENTED_EDGE('',*,*,#16299,.T.);
#22838=ORIENTED_EDGE('',*,*,#16300,.T.);
#22839=ORIENTED_EDGE('',*,*,#16301,.T.);
#22840=ORIENTED_EDGE('',*,*,#16302,.T.);
#22841=ORIENTED_EDGE('',*,*,#16303,.T.);
#22842=ORIENTED_EDGE('',*,*,#16304,.T.);
#22843=ORIENTED_EDGE('',*,*,#16305,.T.);
#22844=ORIENTED_EDGE('',*,*,#16306,.T.);
#22845=ORIENTED_EDGE('',*,*,#16307,.T.);
#22846=ORIENTED_EDGE('',*,*,#16308,.T.);
#22847=ORIENTED_EDGE('',*,*,#16309,.T.);
#22848=ORIENTED_EDGE('',*,*,#16310,.T.);
#22849=ORIENTED_EDGE('',*,*,#16311,.T.);
#22850=ORIENTED_EDGE('',*,*,#16312,.T.);
#22851=ORIENTED_EDGE('',*,*,#16313,.T.);
#22852=ORIENTED_EDGE('',*,*,#16314,.T.);
#22853=ORIENTED_EDGE('',*,*,#16315,.T.);
#22854=ORIENTED_EDGE('',*,*,#16316,.T.);
#22855=ORIENTED_EDGE('',*,*,#16317,.T.);
#22856=ORIENTED_EDGE('',*,*,#16318,.T.);
#22857=ORIENTED_EDGE('',*,*,#16319,.T.);
#22858=ORIENTED_EDGE('',*,*,#16320,.T.);
#22859=ORIENTED_EDGE('',*,*,#16321,.T.);
#22860=ORIENTED_EDGE('',*,*,#16322,.T.);
#22861=ORIENTED_EDGE('',*,*,#16323,.T.);
#22862=ORIENTED_EDGE('',*,*,#16324,.T.);
#22863=ORIENTED_EDGE('',*,*,#16325,.T.);
#22864=ORIENTED_EDGE('',*,*,#16326,.T.);
#22865=ORIENTED_EDGE('',*,*,#16327,.T.);
#22866=ORIENTED_EDGE('',*,*,#16328,.T.);
#22867=ORIENTED_EDGE('',*,*,#16329,.T.);
#22868=ORIENTED_EDGE('',*,*,#16330,.T.);
#22869=ORIENTED_EDGE('',*,*,#16331,.T.);
#22870=ORIENTED_EDGE('',*,*,#16332,.T.);
#22871=ORIENTED_EDGE('',*,*,#16333,.T.);
#22872=ORIENTED_EDGE('',*,*,#16334,.T.);
#22873=ORIENTED_EDGE('',*,*,#16335,.T.);
#22874=ORIENTED_EDGE('',*,*,#16336,.T.);
#22875=ORIENTED_EDGE('',*,*,#16337,.T.);
#22876=ORIENTED_EDGE('',*,*,#16338,.T.);
#22877=ORIENTED_EDGE('',*,*,#16339,.T.);
#22878=ORIENTED_EDGE('',*,*,#16340,.T.);
#22879=ORIENTED_EDGE('',*,*,#16341,.T.);
#22880=ORIENTED_EDGE('',*,*,#16342,.T.);
#22881=ORIENTED_EDGE('',*,*,#16343,.T.);
#22882=ORIENTED_EDGE('',*,*,#16344,.T.);
#22883=ORIENTED_EDGE('',*,*,#16345,.T.);
#22884=ORIENTED_EDGE('',*,*,#16346,.T.);
#22885=ORIENTED_EDGE('',*,*,#16347,.T.);
#22886=ORIENTED_EDGE('',*,*,#16348,.T.);
#22887=ORIENTED_EDGE('',*,*,#16261,.T.);
#22888=ORIENTED_EDGE('',*,*,#16263,.T.);
#22889=ORIENTED_EDGE('',*,*,#16349,.T.);
#22890=ORIENTED_EDGE('',*,*,#16350,.T.);
#22891=ORIENTED_EDGE('',*,*,#16351,.T.);
#22892=ORIENTED_EDGE('',*,*,#16352,.T.);
#22893=ORIENTED_EDGE('',*,*,#16353,.T.);
#22894=ORIENTED_EDGE('',*,*,#16354,.T.);
#22895=ORIENTED_EDGE('',*,*,#16355,.T.);
#22896=ORIENTED_EDGE('',*,*,#16356,.T.);
#22897=ORIENTED_EDGE('',*,*,#16357,.T.);
#22898=ORIENTED_EDGE('',*,*,#16358,.T.);
#22899=ORIENTED_EDGE('',*,*,#16359,.T.);
#22900=ORIENTED_EDGE('',*,*,#16360,.T.);
#22901=ORIENTED_EDGE('',*,*,#16361,.T.);
#22902=ORIENTED_EDGE('',*,*,#16362,.T.);
#22903=ORIENTED_EDGE('',*,*,#16363,.T.);
#22904=ORIENTED_EDGE('',*,*,#16364,.T.);
#22905=ORIENTED_EDGE('',*,*,#16365,.T.);
#22906=ORIENTED_EDGE('',*,*,#16366,.T.);
#22907=ORIENTED_EDGE('',*,*,#16367,.T.);
#22908=ORIENTED_EDGE('',*,*,#16368,.T.);
#22909=ORIENTED_EDGE('',*,*,#16369,.T.);
#22910=ORIENTED_EDGE('',*,*,#16370,.T.);
#22911=ORIENTED_EDGE('',*,*,#16371,.T.);
#22912=ORIENTED_EDGE('',*,*,#16372,.T.);
#22913=ORIENTED_EDGE('',*,*,#16373,.T.);
#22914=ORIENTED_EDGE('',*,*,#16372,.F.);
#22915=ORIENTED_EDGE('',*,*,#16374,.F.);
#22916=ORIENTED_EDGE('',*,*,#16375,.T.);
#22917=ORIENTED_EDGE('',*,*,#16376,.F.);
#22918=ORIENTED_EDGE('',*,*,#16350,.F.);
#22919=ORIENTED_EDGE('',*,*,#16377,.F.);
#22920=ORIENTED_EDGE('',*,*,#16351,.F.);
#22921=ORIENTED_EDGE('',*,*,#16376,.T.);
#22922=ORIENTED_EDGE('',*,*,#16378,.T.);
#22923=ORIENTED_EDGE('',*,*,#16379,.F.);
#22924=ORIENTED_EDGE('',*,*,#16378,.F.);
#22925=ORIENTED_EDGE('',*,*,#16375,.F.);
#22926=ORIENTED_EDGE('',*,*,#16380,.F.);
#22927=ORIENTED_EDGE('',*,*,#16381,.T.);
#22928=ORIENTED_EDGE('',*,*,#16382,.F.);
#22929=ORIENTED_EDGE('',*,*,#16353,.F.);
#22930=ORIENTED_EDGE('',*,*,#16383,.F.);
#22931=ORIENTED_EDGE('',*,*,#16354,.F.);
#22932=ORIENTED_EDGE('',*,*,#16382,.T.);
#22933=ORIENTED_EDGE('',*,*,#16384,.T.);
#22934=ORIENTED_EDGE('',*,*,#16385,.F.);
#22935=ORIENTED_EDGE('',*,*,#16384,.F.);
#22936=ORIENTED_EDGE('',*,*,#16381,.F.);
#22937=ORIENTED_EDGE('',*,*,#16386,.F.);
#22938=ORIENTED_EDGE('',*,*,#16387,.T.);
#22939=ORIENTED_EDGE('',*,*,#16388,.F.);
#22940=ORIENTED_EDGE('',*,*,#16356,.F.);
#22941=ORIENTED_EDGE('',*,*,#16389,.F.);
#22942=ORIENTED_EDGE('',*,*,#16357,.F.);
#22943=ORIENTED_EDGE('',*,*,#16388,.T.);
#22944=ORIENTED_EDGE('',*,*,#16390,.T.);
#22945=ORIENTED_EDGE('',*,*,#16391,.F.);
#22946=ORIENTED_EDGE('',*,*,#16390,.F.);
#22947=ORIENTED_EDGE('',*,*,#16387,.F.);
#22948=ORIENTED_EDGE('',*,*,#16392,.F.);
#22949=ORIENTED_EDGE('',*,*,#16393,.T.);
#22950=ORIENTED_EDGE('',*,*,#16394,.F.);
#22951=ORIENTED_EDGE('',*,*,#16359,.F.);
#22952=ORIENTED_EDGE('',*,*,#16395,.F.);
#22953=ORIENTED_EDGE('',*,*,#16360,.F.);
#22954=ORIENTED_EDGE('',*,*,#16394,.T.);
#22955=ORIENTED_EDGE('',*,*,#16396,.T.);
#22956=ORIENTED_EDGE('',*,*,#16397,.F.);
#22957=ORIENTED_EDGE('',*,*,#16396,.F.);
#22958=ORIENTED_EDGE('',*,*,#16393,.F.);
#22959=ORIENTED_EDGE('',*,*,#16398,.F.);
#22960=ORIENTED_EDGE('',*,*,#16399,.T.);
#22961=ORIENTED_EDGE('',*,*,#16400,.F.);
#22962=ORIENTED_EDGE('',*,*,#16362,.F.);
#22963=ORIENTED_EDGE('',*,*,#16401,.F.);
#22964=ORIENTED_EDGE('',*,*,#16363,.F.);
#22965=ORIENTED_EDGE('',*,*,#16400,.T.);
#22966=ORIENTED_EDGE('',*,*,#16402,.T.);
#22967=ORIENTED_EDGE('',*,*,#16403,.F.);
#22968=ORIENTED_EDGE('',*,*,#16402,.F.);
#22969=ORIENTED_EDGE('',*,*,#16399,.F.);
#22970=ORIENTED_EDGE('',*,*,#16404,.F.);
#22971=ORIENTED_EDGE('',*,*,#16405,.T.);
#22972=ORIENTED_EDGE('',*,*,#16406,.F.);
#22973=ORIENTED_EDGE('',*,*,#16365,.F.);
#22974=ORIENTED_EDGE('',*,*,#16407,.F.);
#22975=ORIENTED_EDGE('',*,*,#16366,.F.);
#22976=ORIENTED_EDGE('',*,*,#16406,.T.);
#22977=ORIENTED_EDGE('',*,*,#16408,.T.);
#22978=ORIENTED_EDGE('',*,*,#16409,.F.);
#22979=ORIENTED_EDGE('',*,*,#16408,.F.);
#22980=ORIENTED_EDGE('',*,*,#16405,.F.);
#22981=ORIENTED_EDGE('',*,*,#16410,.F.);
#22982=ORIENTED_EDGE('',*,*,#16411,.T.);
#22983=ORIENTED_EDGE('',*,*,#16412,.F.);
#22984=ORIENTED_EDGE('',*,*,#16368,.F.);
#22985=ORIENTED_EDGE('',*,*,#16413,.F.);
#22986=ORIENTED_EDGE('',*,*,#16369,.F.);
#22987=ORIENTED_EDGE('',*,*,#16412,.T.);
#22988=ORIENTED_EDGE('',*,*,#16414,.T.);
#22989=ORIENTED_EDGE('',*,*,#16415,.F.);
#22990=ORIENTED_EDGE('',*,*,#16414,.F.);
#22991=ORIENTED_EDGE('',*,*,#16411,.F.);
#22992=ORIENTED_EDGE('',*,*,#16416,.F.);
#22993=ORIENTED_EDGE('',*,*,#16417,.T.);
#22994=ORIENTED_EDGE('',*,*,#16418,.F.);
#22995=ORIENTED_EDGE('',*,*,#16371,.F.);
#22996=ORIENTED_EDGE('',*,*,#16419,.F.);
#22997=ORIENTED_EDGE('',*,*,#16266,.F.);
#22998=ORIENTED_EDGE('',*,*,#16418,.T.);
#22999=ORIENTED_EDGE('',*,*,#16420,.T.);
#23000=ORIENTED_EDGE('',*,*,#16421,.F.);
#23001=ORIENTED_EDGE('',*,*,#16420,.F.);
#23002=ORIENTED_EDGE('',*,*,#16417,.F.);
#23003=ORIENTED_EDGE('',*,*,#16422,.F.);
#23004=ORIENTED_EDGE('',*,*,#16423,.F.);
#23005=ORIENTED_EDGE('',*,*,#16424,.T.);
#23006=ORIENTED_EDGE('',*,*,#16425,.F.);
#23007=ORIENTED_EDGE('',*,*,#16268,.F.);
#23008=ORIENTED_EDGE('',*,*,#16426,.F.);
#23009=ORIENTED_EDGE('',*,*,#16269,.F.);
#23010=ORIENTED_EDGE('',*,*,#16425,.T.);
#23011=ORIENTED_EDGE('',*,*,#16427,.T.);
#23012=ORIENTED_EDGE('',*,*,#16428,.F.);
#23013=ORIENTED_EDGE('',*,*,#16427,.F.);
#23014=ORIENTED_EDGE('',*,*,#16424,.F.);
#23015=ORIENTED_EDGE('',*,*,#16429,.F.);
#23016=ORIENTED_EDGE('',*,*,#16430,.T.);
#23017=ORIENTED_EDGE('',*,*,#16431,.F.);
#23018=ORIENTED_EDGE('',*,*,#16271,.F.);
#23019=ORIENTED_EDGE('',*,*,#16432,.F.);
#23020=ORIENTED_EDGE('',*,*,#16272,.F.);
#23021=ORIENTED_EDGE('',*,*,#16431,.T.);
#23022=ORIENTED_EDGE('',*,*,#16433,.T.);
#23023=ORIENTED_EDGE('',*,*,#16434,.F.);
#23024=ORIENTED_EDGE('',*,*,#16433,.F.);
#23025=ORIENTED_EDGE('',*,*,#16430,.F.);
#23026=ORIENTED_EDGE('',*,*,#16435,.F.);
#23027=ORIENTED_EDGE('',*,*,#16436,.T.);
#23028=ORIENTED_EDGE('',*,*,#16437,.F.);
#23029=ORIENTED_EDGE('',*,*,#16274,.F.);
#23030=ORIENTED_EDGE('',*,*,#16438,.F.);
#23031=ORIENTED_EDGE('',*,*,#16275,.F.);
#23032=ORIENTED_EDGE('',*,*,#16437,.T.);
#23033=ORIENTED_EDGE('',*,*,#16439,.T.);
#23034=ORIENTED_EDGE('',*,*,#16440,.F.);
#23035=ORIENTED_EDGE('',*,*,#16439,.F.);
#23036=ORIENTED_EDGE('',*,*,#16436,.F.);
#23037=ORIENTED_EDGE('',*,*,#16441,.F.);
#23038=ORIENTED_EDGE('',*,*,#16442,.T.);
#23039=ORIENTED_EDGE('',*,*,#16443,.F.);
#23040=ORIENTED_EDGE('',*,*,#16277,.F.);
#23041=ORIENTED_EDGE('',*,*,#16444,.F.);
#23042=ORIENTED_EDGE('',*,*,#16278,.F.);
#23043=ORIENTED_EDGE('',*,*,#16443,.T.);
#23044=ORIENTED_EDGE('',*,*,#16445,.T.);
#23045=ORIENTED_EDGE('',*,*,#16446,.F.);
#23046=ORIENTED_EDGE('',*,*,#16445,.F.);
#23047=ORIENTED_EDGE('',*,*,#16442,.F.);
#23048=ORIENTED_EDGE('',*,*,#16447,.F.);
#23049=ORIENTED_EDGE('',*,*,#16448,.T.);
#23050=ORIENTED_EDGE('',*,*,#16449,.F.);
#23051=ORIENTED_EDGE('',*,*,#16280,.F.);
#23052=ORIENTED_EDGE('',*,*,#16450,.F.);
#23053=ORIENTED_EDGE('',*,*,#16281,.F.);
#23054=ORIENTED_EDGE('',*,*,#16449,.T.);
#23055=ORIENTED_EDGE('',*,*,#16451,.T.);
#23056=ORIENTED_EDGE('',*,*,#16452,.F.);
#23057=ORIENTED_EDGE('',*,*,#16451,.F.);
#23058=ORIENTED_EDGE('',*,*,#16448,.F.);
#23059=ORIENTED_EDGE('',*,*,#16453,.F.);
#23060=ORIENTED_EDGE('',*,*,#16454,.T.);
#23061=ORIENTED_EDGE('',*,*,#16455,.F.);
#23062=ORIENTED_EDGE('',*,*,#16283,.F.);
#23063=ORIENTED_EDGE('',*,*,#16456,.F.);
#23064=ORIENTED_EDGE('',*,*,#16284,.F.);
#23065=ORIENTED_EDGE('',*,*,#16455,.T.);
#23066=ORIENTED_EDGE('',*,*,#16457,.T.);
#23067=ORIENTED_EDGE('',*,*,#16458,.F.);
#23068=ORIENTED_EDGE('',*,*,#16457,.F.);
#23069=ORIENTED_EDGE('',*,*,#16454,.F.);
#23070=ORIENTED_EDGE('',*,*,#16459,.F.);
#23071=ORIENTED_EDGE('',*,*,#16460,.T.);
#23072=ORIENTED_EDGE('',*,*,#16461,.F.);
#23073=ORIENTED_EDGE('',*,*,#16286,.F.);
#23074=ORIENTED_EDGE('',*,*,#16462,.F.);
#23075=ORIENTED_EDGE('',*,*,#16287,.F.);
#23076=ORIENTED_EDGE('',*,*,#16461,.T.);
#23077=ORIENTED_EDGE('',*,*,#16463,.T.);
#23078=ORIENTED_EDGE('',*,*,#16464,.F.);
#23079=ORIENTED_EDGE('',*,*,#16463,.F.);
#23080=ORIENTED_EDGE('',*,*,#16460,.F.);
#23081=ORIENTED_EDGE('',*,*,#16465,.F.);
#23082=ORIENTED_EDGE('',*,*,#16466,.T.);
#23083=ORIENTED_EDGE('',*,*,#16467,.F.);
#23084=ORIENTED_EDGE('',*,*,#16289,.F.);
#23085=ORIENTED_EDGE('',*,*,#16468,.F.);
#23086=ORIENTED_EDGE('',*,*,#16290,.F.);
#23087=ORIENTED_EDGE('',*,*,#16467,.T.);
#23088=ORIENTED_EDGE('',*,*,#16469,.T.);
#23089=ORIENTED_EDGE('',*,*,#16470,.F.);
#23090=ORIENTED_EDGE('',*,*,#16469,.F.);
#23091=ORIENTED_EDGE('',*,*,#16466,.F.);
#23092=ORIENTED_EDGE('',*,*,#16471,.F.);
#23093=ORIENTED_EDGE('',*,*,#16472,.T.);
#23094=ORIENTED_EDGE('',*,*,#16473,.F.);
#23095=ORIENTED_EDGE('',*,*,#16292,.F.);
#23096=ORIENTED_EDGE('',*,*,#16474,.F.);
#23097=ORIENTED_EDGE('',*,*,#16293,.F.);
#23098=ORIENTED_EDGE('',*,*,#16473,.T.);
#23099=ORIENTED_EDGE('',*,*,#16475,.T.);
#23100=ORIENTED_EDGE('',*,*,#16476,.F.);
#23101=ORIENTED_EDGE('',*,*,#16475,.F.);
#23102=ORIENTED_EDGE('',*,*,#16472,.F.);
#23103=ORIENTED_EDGE('',*,*,#16477,.F.);
#23104=ORIENTED_EDGE('',*,*,#16478,.T.);
#23105=ORIENTED_EDGE('',*,*,#16479,.F.);
#23106=ORIENTED_EDGE('',*,*,#16295,.F.);
#23107=ORIENTED_EDGE('',*,*,#16480,.F.);
#23108=ORIENTED_EDGE('',*,*,#16296,.F.);
#23109=ORIENTED_EDGE('',*,*,#16479,.T.);
#23110=ORIENTED_EDGE('',*,*,#16481,.T.);
#23111=ORIENTED_EDGE('',*,*,#16482,.F.);
#23112=ORIENTED_EDGE('',*,*,#16481,.F.);
#23113=ORIENTED_EDGE('',*,*,#16478,.F.);
#23114=ORIENTED_EDGE('',*,*,#16483,.F.);
#23115=ORIENTED_EDGE('',*,*,#16484,.T.);
#23116=ORIENTED_EDGE('',*,*,#16485,.F.);
#23117=ORIENTED_EDGE('',*,*,#16298,.F.);
#23118=ORIENTED_EDGE('',*,*,#16486,.F.);
#23119=ORIENTED_EDGE('',*,*,#16299,.F.);
#23120=ORIENTED_EDGE('',*,*,#16485,.T.);
#23121=ORIENTED_EDGE('',*,*,#16487,.T.);
#23122=ORIENTED_EDGE('',*,*,#16488,.F.);
#23123=ORIENTED_EDGE('',*,*,#16487,.F.);
#23124=ORIENTED_EDGE('',*,*,#16484,.F.);
#23125=ORIENTED_EDGE('',*,*,#16489,.F.);
#23126=ORIENTED_EDGE('',*,*,#16490,.T.);
#23127=ORIENTED_EDGE('',*,*,#16491,.F.);
#23128=ORIENTED_EDGE('',*,*,#16301,.F.);
#23129=ORIENTED_EDGE('',*,*,#16492,.F.);
#23130=ORIENTED_EDGE('',*,*,#16302,.F.);
#23131=ORIENTED_EDGE('',*,*,#16491,.T.);
#23132=ORIENTED_EDGE('',*,*,#16493,.T.);
#23133=ORIENTED_EDGE('',*,*,#16494,.F.);
#23134=ORIENTED_EDGE('',*,*,#16493,.F.);
#23135=ORIENTED_EDGE('',*,*,#16490,.F.);
#23136=ORIENTED_EDGE('',*,*,#16495,.F.);
#23137=ORIENTED_EDGE('',*,*,#16496,.T.);
#23138=ORIENTED_EDGE('',*,*,#16497,.F.);
#23139=ORIENTED_EDGE('',*,*,#16304,.F.);
#23140=ORIENTED_EDGE('',*,*,#16498,.F.);
#23141=ORIENTED_EDGE('',*,*,#16305,.F.);
#23142=ORIENTED_EDGE('',*,*,#16497,.T.);
#23143=ORIENTED_EDGE('',*,*,#16499,.T.);
#23144=ORIENTED_EDGE('',*,*,#16500,.F.);
#23145=ORIENTED_EDGE('',*,*,#16499,.F.);
#23146=ORIENTED_EDGE('',*,*,#16496,.F.);
#23147=ORIENTED_EDGE('',*,*,#16501,.F.);
#23148=ORIENTED_EDGE('',*,*,#16502,.T.);
#23149=ORIENTED_EDGE('',*,*,#16503,.F.);
#23150=ORIENTED_EDGE('',*,*,#16307,.F.);
#23151=ORIENTED_EDGE('',*,*,#16504,.F.);
#23152=ORIENTED_EDGE('',*,*,#16308,.F.);
#23153=ORIENTED_EDGE('',*,*,#16503,.T.);
#23154=ORIENTED_EDGE('',*,*,#16505,.T.);
#23155=ORIENTED_EDGE('',*,*,#16506,.F.);
#23156=ORIENTED_EDGE('',*,*,#16505,.F.);
#23157=ORIENTED_EDGE('',*,*,#16502,.F.);
#23158=ORIENTED_EDGE('',*,*,#16507,.F.);
#23159=ORIENTED_EDGE('',*,*,#16508,.T.);
#23160=ORIENTED_EDGE('',*,*,#16509,.F.);
#23161=ORIENTED_EDGE('',*,*,#16310,.F.);
#23162=ORIENTED_EDGE('',*,*,#16510,.F.);
#23163=ORIENTED_EDGE('',*,*,#16311,.F.);
#23164=ORIENTED_EDGE('',*,*,#16509,.T.);
#23165=ORIENTED_EDGE('',*,*,#16511,.T.);
#23166=ORIENTED_EDGE('',*,*,#16512,.F.);
#23167=ORIENTED_EDGE('',*,*,#16511,.F.);
#23168=ORIENTED_EDGE('',*,*,#16508,.F.);
#23169=ORIENTED_EDGE('',*,*,#16513,.F.);
#23170=ORIENTED_EDGE('',*,*,#16514,.T.);
#23171=ORIENTED_EDGE('',*,*,#16515,.F.);
#23172=ORIENTED_EDGE('',*,*,#16313,.F.);
#23173=ORIENTED_EDGE('',*,*,#16516,.F.);
#23174=ORIENTED_EDGE('',*,*,#16314,.F.);
#23175=ORIENTED_EDGE('',*,*,#16515,.T.);
#23176=ORIENTED_EDGE('',*,*,#16517,.T.);
#23177=ORIENTED_EDGE('',*,*,#16518,.F.);
#23178=ORIENTED_EDGE('',*,*,#16517,.F.);
#23179=ORIENTED_EDGE('',*,*,#16514,.F.);
#23180=ORIENTED_EDGE('',*,*,#16519,.F.);
#23181=ORIENTED_EDGE('',*,*,#16520,.T.);
#23182=ORIENTED_EDGE('',*,*,#16521,.F.);
#23183=ORIENTED_EDGE('',*,*,#16316,.F.);
#23184=ORIENTED_EDGE('',*,*,#16522,.F.);
#23185=ORIENTED_EDGE('',*,*,#16317,.F.);
#23186=ORIENTED_EDGE('',*,*,#16521,.T.);
#23187=ORIENTED_EDGE('',*,*,#16523,.T.);
#23188=ORIENTED_EDGE('',*,*,#16524,.F.);
#23189=ORIENTED_EDGE('',*,*,#16523,.F.);
#23190=ORIENTED_EDGE('',*,*,#16520,.F.);
#23191=ORIENTED_EDGE('',*,*,#16525,.F.);
#23192=ORIENTED_EDGE('',*,*,#16526,.T.);
#23193=ORIENTED_EDGE('',*,*,#16527,.F.);
#23194=ORIENTED_EDGE('',*,*,#16319,.F.);
#23195=ORIENTED_EDGE('',*,*,#16528,.F.);
#23196=ORIENTED_EDGE('',*,*,#16320,.F.);
#23197=ORIENTED_EDGE('',*,*,#16527,.T.);
#23198=ORIENTED_EDGE('',*,*,#16529,.T.);
#23199=ORIENTED_EDGE('',*,*,#16530,.F.);
#23200=ORIENTED_EDGE('',*,*,#16529,.F.);
#23201=ORIENTED_EDGE('',*,*,#16526,.F.);
#23202=ORIENTED_EDGE('',*,*,#16531,.F.);
#23203=ORIENTED_EDGE('',*,*,#16532,.T.);
#23204=ORIENTED_EDGE('',*,*,#16533,.F.);
#23205=ORIENTED_EDGE('',*,*,#16322,.F.);
#23206=ORIENTED_EDGE('',*,*,#16534,.F.);
#23207=ORIENTED_EDGE('',*,*,#16323,.F.);
#23208=ORIENTED_EDGE('',*,*,#16533,.T.);
#23209=ORIENTED_EDGE('',*,*,#16535,.T.);
#23210=ORIENTED_EDGE('',*,*,#16536,.F.);
#23211=ORIENTED_EDGE('',*,*,#16535,.F.);
#23212=ORIENTED_EDGE('',*,*,#16532,.F.);
#23213=ORIENTED_EDGE('',*,*,#16537,.F.);
#23214=ORIENTED_EDGE('',*,*,#16538,.T.);
#23215=ORIENTED_EDGE('',*,*,#16539,.F.);
#23216=ORIENTED_EDGE('',*,*,#16325,.F.);
#23217=ORIENTED_EDGE('',*,*,#16540,.F.);
#23218=ORIENTED_EDGE('',*,*,#16326,.F.);
#23219=ORIENTED_EDGE('',*,*,#16539,.T.);
#23220=ORIENTED_EDGE('',*,*,#16541,.T.);
#23221=ORIENTED_EDGE('',*,*,#16542,.F.);
#23222=ORIENTED_EDGE('',*,*,#16541,.F.);
#23223=ORIENTED_EDGE('',*,*,#16538,.F.);
#23224=ORIENTED_EDGE('',*,*,#16543,.F.);
#23225=ORIENTED_EDGE('',*,*,#16544,.T.);
#23226=ORIENTED_EDGE('',*,*,#16545,.F.);
#23227=ORIENTED_EDGE('',*,*,#16328,.F.);
#23228=ORIENTED_EDGE('',*,*,#16546,.F.);
#23229=ORIENTED_EDGE('',*,*,#16329,.F.);
#23230=ORIENTED_EDGE('',*,*,#16545,.T.);
#23231=ORIENTED_EDGE('',*,*,#16547,.T.);
#23232=ORIENTED_EDGE('',*,*,#16548,.F.);
#23233=ORIENTED_EDGE('',*,*,#16547,.F.);
#23234=ORIENTED_EDGE('',*,*,#16544,.F.);
#23235=ORIENTED_EDGE('',*,*,#16549,.F.);
#23236=ORIENTED_EDGE('',*,*,#16550,.T.);
#23237=ORIENTED_EDGE('',*,*,#16551,.F.);
#23238=ORIENTED_EDGE('',*,*,#16331,.F.);
#23239=ORIENTED_EDGE('',*,*,#16552,.F.);
#23240=ORIENTED_EDGE('',*,*,#16332,.F.);
#23241=ORIENTED_EDGE('',*,*,#16551,.T.);
#23242=ORIENTED_EDGE('',*,*,#16553,.T.);
#23243=ORIENTED_EDGE('',*,*,#16554,.F.);
#23244=ORIENTED_EDGE('',*,*,#16553,.F.);
#23245=ORIENTED_EDGE('',*,*,#16550,.F.);
#23246=ORIENTED_EDGE('',*,*,#16555,.F.);
#23247=ORIENTED_EDGE('',*,*,#16556,.T.);
#23248=ORIENTED_EDGE('',*,*,#16557,.F.);
#23249=ORIENTED_EDGE('',*,*,#16334,.F.);
#23250=ORIENTED_EDGE('',*,*,#16558,.F.);
#23251=ORIENTED_EDGE('',*,*,#16335,.F.);
#23252=ORIENTED_EDGE('',*,*,#16557,.T.);
#23253=ORIENTED_EDGE('',*,*,#16559,.T.);
#23254=ORIENTED_EDGE('',*,*,#16560,.F.);
#23255=ORIENTED_EDGE('',*,*,#16559,.F.);
#23256=ORIENTED_EDGE('',*,*,#16556,.F.);
#23257=ORIENTED_EDGE('',*,*,#16561,.F.);
#23258=ORIENTED_EDGE('',*,*,#16562,.T.);
#23259=ORIENTED_EDGE('',*,*,#16563,.F.);
#23260=ORIENTED_EDGE('',*,*,#16337,.F.);
#23261=ORIENTED_EDGE('',*,*,#16564,.F.);
#23262=ORIENTED_EDGE('',*,*,#16338,.F.);
#23263=ORIENTED_EDGE('',*,*,#16563,.T.);
#23264=ORIENTED_EDGE('',*,*,#16565,.T.);
#23265=ORIENTED_EDGE('',*,*,#16566,.F.);
#23266=ORIENTED_EDGE('',*,*,#16565,.F.);
#23267=ORIENTED_EDGE('',*,*,#16562,.F.);
#23268=ORIENTED_EDGE('',*,*,#16567,.F.);
#23269=ORIENTED_EDGE('',*,*,#16568,.T.);
#23270=ORIENTED_EDGE('',*,*,#16569,.F.);
#23271=ORIENTED_EDGE('',*,*,#16340,.F.);
#23272=ORIENTED_EDGE('',*,*,#16570,.F.);
#23273=ORIENTED_EDGE('',*,*,#16341,.F.);
#23274=ORIENTED_EDGE('',*,*,#16569,.T.);
#23275=ORIENTED_EDGE('',*,*,#16571,.T.);
#23276=ORIENTED_EDGE('',*,*,#16572,.F.);
#23277=ORIENTED_EDGE('',*,*,#16571,.F.);
#23278=ORIENTED_EDGE('',*,*,#16568,.F.);
#23279=ORIENTED_EDGE('',*,*,#16573,.F.);
#23280=ORIENTED_EDGE('',*,*,#16574,.T.);
#23281=ORIENTED_EDGE('',*,*,#16575,.F.);
#23282=ORIENTED_EDGE('',*,*,#16343,.F.);
#23283=ORIENTED_EDGE('',*,*,#16576,.F.);
#23284=ORIENTED_EDGE('',*,*,#16344,.F.);
#23285=ORIENTED_EDGE('',*,*,#16575,.T.);
#23286=ORIENTED_EDGE('',*,*,#16577,.T.);
#23287=ORIENTED_EDGE('',*,*,#16578,.F.);
#23288=ORIENTED_EDGE('',*,*,#16577,.F.);
#23289=ORIENTED_EDGE('',*,*,#16574,.F.);
#23290=ORIENTED_EDGE('',*,*,#16579,.F.);
#23291=ORIENTED_EDGE('',*,*,#16580,.T.);
#23292=ORIENTED_EDGE('',*,*,#16581,.F.);
#23293=ORIENTED_EDGE('',*,*,#16346,.F.);
#23294=ORIENTED_EDGE('',*,*,#16582,.F.);
#23295=ORIENTED_EDGE('',*,*,#16347,.F.);
#23296=ORIENTED_EDGE('',*,*,#16581,.T.);
#23297=ORIENTED_EDGE('',*,*,#16583,.T.);
#23298=ORIENTED_EDGE('',*,*,#16584,.F.);
#23299=ORIENTED_EDGE('',*,*,#16583,.F.);
#23300=ORIENTED_EDGE('',*,*,#16580,.F.);
#23301=ORIENTED_EDGE('',*,*,#16421,.T.);
#23302=ORIENTED_EDGE('',*,*,#16585,.T.);
#23303=ORIENTED_EDGE('',*,*,#16255,.T.);
#23304=ORIENTED_EDGE('',*,*,#16585,.F.);
#23305=ORIENTED_EDGE('',*,*,#16422,.T.);
#23306=ORIENTED_EDGE('',*,*,#16416,.T.);
#23307=ORIENTED_EDGE('',*,*,#16370,.F.);
#23308=ORIENTED_EDGE('',*,*,#16413,.T.);
#23309=ORIENTED_EDGE('',*,*,#16415,.T.);
#23310=ORIENTED_EDGE('',*,*,#16410,.T.);
#23311=ORIENTED_EDGE('',*,*,#16367,.F.);
#23312=ORIENTED_EDGE('',*,*,#16407,.T.);
#23313=ORIENTED_EDGE('',*,*,#16409,.T.);
#23314=ORIENTED_EDGE('',*,*,#16404,.T.);
#23315=ORIENTED_EDGE('',*,*,#16364,.F.);
#23316=ORIENTED_EDGE('',*,*,#16401,.T.);
#23317=ORIENTED_EDGE('',*,*,#16403,.T.);
#23318=ORIENTED_EDGE('',*,*,#16398,.T.);
#23319=ORIENTED_EDGE('',*,*,#16361,.F.);
#23320=ORIENTED_EDGE('',*,*,#16395,.T.);
#23321=ORIENTED_EDGE('',*,*,#16397,.T.);
#23322=ORIENTED_EDGE('',*,*,#16392,.T.);
#23323=ORIENTED_EDGE('',*,*,#16358,.F.);
#23324=ORIENTED_EDGE('',*,*,#16389,.T.);
#23325=ORIENTED_EDGE('',*,*,#16391,.T.);
#23326=ORIENTED_EDGE('',*,*,#16386,.T.);
#23327=ORIENTED_EDGE('',*,*,#16355,.F.);
#23328=ORIENTED_EDGE('',*,*,#16383,.T.);
#23329=ORIENTED_EDGE('',*,*,#16385,.T.);
#23330=ORIENTED_EDGE('',*,*,#16380,.T.);
#23331=ORIENTED_EDGE('',*,*,#16352,.F.);
#23332=ORIENTED_EDGE('',*,*,#16377,.T.);
#23333=ORIENTED_EDGE('',*,*,#16379,.T.);
#23334=ORIENTED_EDGE('',*,*,#16374,.T.);
#23335=ORIENTED_EDGE('',*,*,#16349,.F.);
#23336=ORIENTED_EDGE('',*,*,#16262,.T.);
#23337=ORIENTED_EDGE('',*,*,#16265,.T.);
#23338=ORIENTED_EDGE('',*,*,#16258,.T.);
#23339=ORIENTED_EDGE('',*,*,#16348,.F.);
#23340=ORIENTED_EDGE('',*,*,#16582,.T.);
#23341=ORIENTED_EDGE('',*,*,#16584,.T.);
#23342=ORIENTED_EDGE('',*,*,#16579,.T.);
#23343=ORIENTED_EDGE('',*,*,#16345,.F.);
#23344=ORIENTED_EDGE('',*,*,#16576,.T.);
#23345=ORIENTED_EDGE('',*,*,#16578,.T.);
#23346=ORIENTED_EDGE('',*,*,#16573,.T.);
#23347=ORIENTED_EDGE('',*,*,#16342,.F.);
#23348=ORIENTED_EDGE('',*,*,#16570,.T.);
#23349=ORIENTED_EDGE('',*,*,#16572,.T.);
#23350=ORIENTED_EDGE('',*,*,#16567,.T.);
#23351=ORIENTED_EDGE('',*,*,#16339,.F.);
#23352=ORIENTED_EDGE('',*,*,#16564,.T.);
#23353=ORIENTED_EDGE('',*,*,#16566,.T.);
#23354=ORIENTED_EDGE('',*,*,#16561,.T.);
#23355=ORIENTED_EDGE('',*,*,#16336,.F.);
#23356=ORIENTED_EDGE('',*,*,#16558,.T.);
#23357=ORIENTED_EDGE('',*,*,#16560,.T.);
#23358=ORIENTED_EDGE('',*,*,#16555,.T.);
#23359=ORIENTED_EDGE('',*,*,#16333,.F.);
#23360=ORIENTED_EDGE('',*,*,#16552,.T.);
#23361=ORIENTED_EDGE('',*,*,#16554,.T.);
#23362=ORIENTED_EDGE('',*,*,#16549,.T.);
#23363=ORIENTED_EDGE('',*,*,#16330,.F.);
#23364=ORIENTED_EDGE('',*,*,#16546,.T.);
#23365=ORIENTED_EDGE('',*,*,#16548,.T.);
#23366=ORIENTED_EDGE('',*,*,#16543,.T.);
#23367=ORIENTED_EDGE('',*,*,#16327,.F.);
#23368=ORIENTED_EDGE('',*,*,#16540,.T.);
#23369=ORIENTED_EDGE('',*,*,#16542,.T.);
#23370=ORIENTED_EDGE('',*,*,#16537,.T.);
#23371=ORIENTED_EDGE('',*,*,#16324,.F.);
#23372=ORIENTED_EDGE('',*,*,#16534,.T.);
#23373=ORIENTED_EDGE('',*,*,#16536,.T.);
#23374=ORIENTED_EDGE('',*,*,#16531,.T.);
#23375=ORIENTED_EDGE('',*,*,#16321,.F.);
#23376=ORIENTED_EDGE('',*,*,#16528,.T.);
#23377=ORIENTED_EDGE('',*,*,#16530,.T.);
#23378=ORIENTED_EDGE('',*,*,#16525,.T.);
#23379=ORIENTED_EDGE('',*,*,#16318,.F.);
#23380=ORIENTED_EDGE('',*,*,#16522,.T.);
#23381=ORIENTED_EDGE('',*,*,#16524,.T.);
#23382=ORIENTED_EDGE('',*,*,#16519,.T.);
#23383=ORIENTED_EDGE('',*,*,#16315,.F.);
#23384=ORIENTED_EDGE('',*,*,#16516,.T.);
#23385=ORIENTED_EDGE('',*,*,#16518,.T.);
#23386=ORIENTED_EDGE('',*,*,#16513,.T.);
#23387=ORIENTED_EDGE('',*,*,#16312,.F.);
#23388=ORIENTED_EDGE('',*,*,#16510,.T.);
#23389=ORIENTED_EDGE('',*,*,#16512,.T.);
#23390=ORIENTED_EDGE('',*,*,#16507,.T.);
#23391=ORIENTED_EDGE('',*,*,#16309,.F.);
#23392=ORIENTED_EDGE('',*,*,#16504,.T.);
#23393=ORIENTED_EDGE('',*,*,#16506,.T.);
#23394=ORIENTED_EDGE('',*,*,#16501,.T.);
#23395=ORIENTED_EDGE('',*,*,#16306,.F.);
#23396=ORIENTED_EDGE('',*,*,#16498,.T.);
#23397=ORIENTED_EDGE('',*,*,#16500,.T.);
#23398=ORIENTED_EDGE('',*,*,#16495,.T.);
#23399=ORIENTED_EDGE('',*,*,#16303,.F.);
#23400=ORIENTED_EDGE('',*,*,#16492,.T.);
#23401=ORIENTED_EDGE('',*,*,#16494,.T.);
#23402=ORIENTED_EDGE('',*,*,#16489,.T.);
#23403=ORIENTED_EDGE('',*,*,#16300,.F.);
#23404=ORIENTED_EDGE('',*,*,#16486,.T.);
#23405=ORIENTED_EDGE('',*,*,#16488,.T.);
#23406=ORIENTED_EDGE('',*,*,#16483,.T.);
#23407=ORIENTED_EDGE('',*,*,#16297,.F.);
#23408=ORIENTED_EDGE('',*,*,#16480,.T.);
#23409=ORIENTED_EDGE('',*,*,#16482,.T.);
#23410=ORIENTED_EDGE('',*,*,#16477,.T.);
#23411=ORIENTED_EDGE('',*,*,#16294,.F.);
#23412=ORIENTED_EDGE('',*,*,#16474,.T.);
#23413=ORIENTED_EDGE('',*,*,#16476,.T.);
#23414=ORIENTED_EDGE('',*,*,#16471,.T.);
#23415=ORIENTED_EDGE('',*,*,#16291,.F.);
#23416=ORIENTED_EDGE('',*,*,#16468,.T.);
#23417=ORIENTED_EDGE('',*,*,#16470,.T.);
#23418=ORIENTED_EDGE('',*,*,#16465,.T.);
#23419=ORIENTED_EDGE('',*,*,#16288,.F.);
#23420=ORIENTED_EDGE('',*,*,#16462,.T.);
#23421=ORIENTED_EDGE('',*,*,#16464,.T.);
#23422=ORIENTED_EDGE('',*,*,#16459,.T.);
#23423=ORIENTED_EDGE('',*,*,#16285,.F.);
#23424=ORIENTED_EDGE('',*,*,#16456,.T.);
#23425=ORIENTED_EDGE('',*,*,#16458,.T.);
#23426=ORIENTED_EDGE('',*,*,#16453,.T.);
#23427=ORIENTED_EDGE('',*,*,#16282,.F.);
#23428=ORIENTED_EDGE('',*,*,#16450,.T.);
#23429=ORIENTED_EDGE('',*,*,#16452,.T.);
#23430=ORIENTED_EDGE('',*,*,#16447,.T.);
#23431=ORIENTED_EDGE('',*,*,#16279,.F.);
#23432=ORIENTED_EDGE('',*,*,#16444,.T.);
#23433=ORIENTED_EDGE('',*,*,#16446,.T.);
#23434=ORIENTED_EDGE('',*,*,#16441,.T.);
#23435=ORIENTED_EDGE('',*,*,#16276,.F.);
#23436=ORIENTED_EDGE('',*,*,#16438,.T.);
#23437=ORIENTED_EDGE('',*,*,#16440,.T.);
#23438=ORIENTED_EDGE('',*,*,#16435,.T.);
#23439=ORIENTED_EDGE('',*,*,#16273,.F.);
#23440=ORIENTED_EDGE('',*,*,#16432,.T.);
#23441=ORIENTED_EDGE('',*,*,#16434,.T.);
#23442=ORIENTED_EDGE('',*,*,#16429,.T.);
#23443=ORIENTED_EDGE('',*,*,#16270,.F.);
#23444=ORIENTED_EDGE('',*,*,#16426,.T.);
#23445=ORIENTED_EDGE('',*,*,#16428,.T.);
#23446=ORIENTED_EDGE('',*,*,#16423,.T.);
#23447=ORIENTED_EDGE('',*,*,#16267,.F.);
#23448=ORIENTED_EDGE('',*,*,#16419,.T.);
#23449=ORIENTED_EDGE('',*,*,#16373,.F.);
#23450=ORIENTED_EDGE('',*,*,#16586,.T.);
#23451=ORIENTED_EDGE('',*,*,#16587,.T.);
#23452=ORIENTED_EDGE('',*,*,#16588,.T.);
#23453=ORIENTED_EDGE('',*,*,#16589,.T.);
#23454=ORIENTED_EDGE('',*,*,#16590,.T.);
#23455=ORIENTED_EDGE('',*,*,#16591,.T.);
#23456=ORIENTED_EDGE('',*,*,#16592,.F.);
#23457=ORIENTED_EDGE('',*,*,#16593,.F.);
#23458=ORIENTED_EDGE('',*,*,#16594,.F.);
#23459=ORIENTED_EDGE('',*,*,#16595,.F.);
#23460=ORIENTED_EDGE('',*,*,#16596,.F.);
#23461=ORIENTED_EDGE('',*,*,#16597,.F.);
#23462=ORIENTED_EDGE('',*,*,#16598,.F.);
#23463=ORIENTED_EDGE('',*,*,#16599,.F.);
#23464=ORIENTED_EDGE('',*,*,#16600,.F.);
#23465=ORIENTED_EDGE('',*,*,#16601,.F.);
#23466=ORIENTED_EDGE('',*,*,#16602,.F.);
#23467=ORIENTED_EDGE('',*,*,#16603,.F.);
#23468=ORIENTED_EDGE('',*,*,#16604,.T.);
#23469=ORIENTED_EDGE('',*,*,#16599,.T.);
#23470=ORIENTED_EDGE('',*,*,#16597,.T.);
#23471=ORIENTED_EDGE('',*,*,#16595,.T.);
#23472=ORIENTED_EDGE('',*,*,#16593,.T.);
#23473=ORIENTED_EDGE('',*,*,#16603,.T.);
#23474=ORIENTED_EDGE('',*,*,#16601,.T.);
#23475=ORIENTED_EDGE('',*,*,#16604,.F.);
#23476=ORIENTED_EDGE('',*,*,#16586,.F.);
#23477=ORIENTED_EDGE('',*,*,#16605,.T.);
#23478=ORIENTED_EDGE('',*,*,#16592,.T.);
#23479=ORIENTED_EDGE('',*,*,#16606,.F.);
#23480=ORIENTED_EDGE('',*,*,#16591,.F.);
#23481=ORIENTED_EDGE('',*,*,#16607,.T.);
#23482=ORIENTED_EDGE('',*,*,#16602,.T.);
#23483=ORIENTED_EDGE('',*,*,#16605,.F.);
#23484=ORIENTED_EDGE('',*,*,#16590,.F.);
#23485=ORIENTED_EDGE('',*,*,#16608,.T.);
#23486=ORIENTED_EDGE('',*,*,#16600,.T.);
#23487=ORIENTED_EDGE('',*,*,#16607,.F.);
#23488=ORIENTED_EDGE('',*,*,#16589,.F.);
#23489=ORIENTED_EDGE('',*,*,#16609,.T.);
#23490=ORIENTED_EDGE('',*,*,#16598,.T.);
#23491=ORIENTED_EDGE('',*,*,#16608,.F.);
#23492=ORIENTED_EDGE('',*,*,#16588,.F.);
#23493=ORIENTED_EDGE('',*,*,#16610,.T.);
#23494=ORIENTED_EDGE('',*,*,#16596,.T.);
#23495=ORIENTED_EDGE('',*,*,#16609,.F.);
#23496=ORIENTED_EDGE('',*,*,#16587,.F.);
#23497=ORIENTED_EDGE('',*,*,#16606,.T.);
#23498=ORIENTED_EDGE('',*,*,#16594,.T.);
#23499=ORIENTED_EDGE('',*,*,#16610,.F.);
#25536=CONICAL_SURFACE('',#28486,1.52934,0.785398163397448);
#25537=CONICAL_SURFACE('',#28493,2.7202,0.785398163397452);
#25538=CONICAL_SURFACE('',#28686,0.801975608296219,1.02974425867665);
#26470=ADVANCED_FACE('',(#3277),#2308,.T.);
#26471=ADVANCED_FACE('',(#3278),#2309,.T.);
#26472=ADVANCED_FACE('',(#3279),#2310,.T.);
#26473=ADVANCED_FACE('',(#3280),#2311,.T.);
#26474=ADVANCED_FACE('',(#3281),#2312,.T.);
#26475=ADVANCED_FACE('',(#3282),#2313,.T.);
#26476=ADVANCED_FACE('',(#3283),#2314,.T.);
#26477=ADVANCED_FACE('',(#3284),#2315,.T.);
#26478=ADVANCED_FACE('',(#3285),#2316,.T.);
#26479=ADVANCED_FACE('',(#3286),#1755,.T.);
#26480=ADVANCED_FACE('',(#3287),#899,.F.);
#26481=ADVANCED_FACE('',(#3288),#1756,.F.);
#26482=ADVANCED_FACE('',(#3289),#900,.F.);
#26483=ADVANCED_FACE('',(#3290),#505,.F.);
#26484=ADVANCED_FACE('',(#3291,#1111),#1757,.F.);
#26485=ADVANCED_FACE('',(#3292),#25536,.T.);
#26486=ADVANCED_FACE('',(#3293),#1758,.F.);
#26487=ADVANCED_FACE('',(#3294),#1759,.F.);
#26488=ADVANCED_FACE('',(#3295),#1760,.F.);
#26489=ADVANCED_FACE('',(#3296),#1761,.F.);
#26490=ADVANCED_FACE('',(#3297),#25537,.T.);
#26491=ADVANCED_FACE('',(#3298),#1762,.F.);
#26492=ADVANCED_FACE('',(#3299),#1763,.F.);
#26493=ADVANCED_FACE('',(#3300),#1764,.F.);
#26494=ADVANCED_FACE('',(#3301),#1765,.F.);
#26495=ADVANCED_FACE('',(#3302),#1766,.F.);
#26496=ADVANCED_FACE('',(#3303),#1767,.F.);
#26497=ADVANCED_FACE('',(#3304),#1768,.F.);
#26498=ADVANCED_FACE('',(#3305),#1769,.F.);
#26499=ADVANCED_FACE('',(#3306),#1770,.F.);
#26500=ADVANCED_FACE('',(#3307),#1771,.F.);
#26501=ADVANCED_FACE('',(#3308),#1772,.F.);
#26502=ADVANCED_FACE('',(#3309),#1773,.F.);
#26503=ADVANCED_FACE('',(#3310),#1774,.F.);
#26504=ADVANCED_FACE('',(#3311),#1775,.F.);
#26505=ADVANCED_FACE('',(#3312),#1776,.F.);
#26506=ADVANCED_FACE('',(#3313),#1777,.F.);
#26507=ADVANCED_FACE('',(#3314),#1778,.F.);
#26508=ADVANCED_FACE('',(#3315),#1779,.F.);
#26509=ADVANCED_FACE('',(#3316),#1780,.F.);
#26510=ADVANCED_FACE('',(#3317),#1781,.F.);
#26511=ADVANCED_FACE('',(#3318),#1782,.F.);
#26512=ADVANCED_FACE('',(#3319),#1783,.F.);
#26513=ADVANCED_FACE('',(#3320),#1784,.F.);
#26514=ADVANCED_FACE('',(#3321),#1785,.F.);
#26515=ADVANCED_FACE('',(#3322),#1786,.F.);
#26516=ADVANCED_FACE('',(#3323),#1787,.F.);
#26517=ADVANCED_FACE('',(#3324),#1788,.F.);
#26518=ADVANCED_FACE('',(#3325),#1789,.F.);
#26519=ADVANCED_FACE('',(#3326),#1790,.F.);
#26520=ADVANCED_FACE('',(#3327),#1791,.F.);
#26521=ADVANCED_FACE('',(#3328),#1792,.F.);
#26522=ADVANCED_FACE('',(#3329),#1793,.F.);
#26523=ADVANCED_FACE('',(#3330),#1794,.F.);
#26524=ADVANCED_FACE('',(#3331),#1795,.F.);
#26525=ADVANCED_FACE('',(#3332),#1796,.F.);
#26526=ADVANCED_FACE('',(#3333),#1797,.F.);
#26527=ADVANCED_FACE('',(#3334),#1798,.F.);
#26528=ADVANCED_FACE('',(#3335),#1799,.F.);
#26529=ADVANCED_FACE('',(#3336),#1800,.F.);
#26530=ADVANCED_FACE('',(#3337),#1801,.F.);
#26531=ADVANCED_FACE('',(#3338),#1802,.F.);
#26532=ADVANCED_FACE('',(#3339),#1803,.F.);
#26533=ADVANCED_FACE('',(#3340),#1804,.F.);
#26534=ADVANCED_FACE('',(#3341),#1805,.F.);
#26535=ADVANCED_FACE('',(#3342),#1806,.F.);
#26536=ADVANCED_FACE('',(#3343),#1807,.F.);
#26537=ADVANCED_FACE('',(#3344),#1808,.F.);
#26538=ADVANCED_FACE('',(#3345),#1809,.F.);
#26539=ADVANCED_FACE('',(#3346),#1810,.F.);
#26540=ADVANCED_FACE('',(#3347),#1811,.F.);
#26541=ADVANCED_FACE('',(#3348),#1812,.F.);
#26542=ADVANCED_FACE('',(#3349),#1813,.F.);
#26543=ADVANCED_FACE('',(#3350),#1814,.F.);
#26544=ADVANCED_FACE('',(#3351),#1815,.F.);
#26545=ADVANCED_FACE('',(#3352),#1816,.F.);
#26546=ADVANCED_FACE('',(#3353),#1817,.F.);
#26547=ADVANCED_FACE('',(#3354),#1818,.F.);
#26548=ADVANCED_FACE('',(#3355),#1819,.F.);
#26549=ADVANCED_FACE('',(#3356),#1820,.F.);
#26550=ADVANCED_FACE('',(#3357),#1821,.F.);
#26551=ADVANCED_FACE('',(#3358),#1822,.F.);
#26552=ADVANCED_FACE('',(#3359),#1823,.F.);
#26553=ADVANCED_FACE('',(#3360),#1824,.F.);
#26554=ADVANCED_FACE('',(#3361),#1825,.F.);
#26555=ADVANCED_FACE('',(#3362),#1826,.F.);
#26556=ADVANCED_FACE('',(#3363),#1827,.F.);
#26557=ADVANCED_FACE('',(#3364),#1828,.F.);
#26558=ADVANCED_FACE('',(#3365),#1829,.F.);
#26559=ADVANCED_FACE('',(#3366),#1830,.F.);
#26560=ADVANCED_FACE('',(#3367),#1831,.F.);
#26561=ADVANCED_FACE('',(#3368),#1832,.F.);
#26562=ADVANCED_FACE('',(#3369),#1833,.F.);
#26563=ADVANCED_FACE('',(#3370),#1834,.F.);
#26564=ADVANCED_FACE('',(#3371),#1835,.F.);
#26565=ADVANCED_FACE('',(#3372),#1836,.F.);
#26566=ADVANCED_FACE('',(#3373),#1837,.F.);
#26567=ADVANCED_FACE('',(#3374),#1838,.F.);
#26568=ADVANCED_FACE('',(#3375),#1839,.F.);
#26569=ADVANCED_FACE('',(#3376),#1840,.F.);
#26570=ADVANCED_FACE('',(#3377),#1841,.F.);
#26571=ADVANCED_FACE('',(#3378),#1842,.F.);
#26572=ADVANCED_FACE('',(#3379),#1843,.F.);
#26573=ADVANCED_FACE('',(#3380),#1844,.F.);
#26574=ADVANCED_FACE('',(#3381),#1845,.F.);
#26575=ADVANCED_FACE('',(#3382),#1846,.F.);
#26576=ADVANCED_FACE('',(#3383),#1847,.F.);
#26577=ADVANCED_FACE('',(#3384),#1848,.F.);
#26578=ADVANCED_FACE('',(#3385),#1849,.F.);
#26579=ADVANCED_FACE('',(#3386),#1850,.F.);
#26580=ADVANCED_FACE('',(#3387),#1851,.F.);
#26581=ADVANCED_FACE('',(#3388),#1852,.F.);
#26582=ADVANCED_FACE('',(#3389),#1853,.F.);
#26583=ADVANCED_FACE('',(#3390),#1854,.F.);
#26584=ADVANCED_FACE('',(#3391),#1855,.F.);
#26585=ADVANCED_FACE('',(#3392),#1856,.F.);
#26586=ADVANCED_FACE('',(#3393),#1857,.F.);
#26587=ADVANCED_FACE('',(#3394),#1858,.F.);
#26588=ADVANCED_FACE('',(#3395),#1859,.F.);
#26589=ADVANCED_FACE('',(#3396),#1860,.F.);
#26590=ADVANCED_FACE('',(#3397),#1861,.F.);
#26591=ADVANCED_FACE('',(#3398),#1862,.F.);
#26592=ADVANCED_FACE('',(#3399),#1863,.F.);
#26593=ADVANCED_FACE('',(#3400),#1864,.F.);
#26594=ADVANCED_FACE('',(#3401),#1865,.F.);
#26595=ADVANCED_FACE('',(#3402),#1866,.F.);
#26596=ADVANCED_FACE('',(#3403),#2317,.T.);
#26597=ADVANCED_FACE('',(#3404,#1112),#1867,.T.);
#26598=ADVANCED_FACE('',(#3405),#1868,.F.);
#26599=ADVANCED_FACE('',(#3406),#1869,.F.);
#26600=ADVANCED_FACE('',(#3407),#1870,.F.);
#26601=ADVANCED_FACE('',(#3408),#1871,.F.);
#26602=ADVANCED_FACE('',(#3409),#1872,.F.);
#26603=ADVANCED_FACE('',(#3410),#1873,.F.);
#26604=ADVANCED_FACE('',(#3411),#25538,.F.);
#26605=ADVANCED_FACE('',(#3412),#1874,.F.);
#26606=ADVANCED_FACE('',(#3413),#1875,.F.);
#26607=ADVANCED_FACE('',(#3414),#1876,.F.);
#26608=ADVANCED_FACE('',(#3415),#1877,.F.);
#26609=ADVANCED_FACE('',(#3416),#1878,.F.);
#26610=ADVANCED_FACE('',(#3417),#1879,.F.);
#26938=CLOSED_SHELL('',(#26470,#26471,#26472,#26473,#26474,#26475,#26476,
#26477,#26478,#26479,#26480,#26481,#26482,#26483,#26484,#26485,#26486,#26487,
#26488,#26489,#26490,#26491,#26492,#26493,#26494,#26495,#26496,#26497,#26498,
#26499,#26500,#26501,#26502,#26503,#26504,#26505,#26506,#26507,#26508,#26509,
#26510,#26511,#26512,#26513,#26514,#26515,#26516,#26517,#26518,#26519,#26520,
#26521,#26522,#26523,#26524,#26525,#26526,#26527,#26528,#26529,#26530,#26531,
#26532,#26533,#26534,#26535,#26536,#26537,#26538,#26539,#26540,#26541,#26542,
#26543,#26544,#26545,#26546,#26547,#26548,#26549,#26550,#26551,#26552,#26553,
#26554,#26555,#26556,#26557,#26558,#26559,#26560,#26561,#26562,#26563,#26564,
#26565,#26566,#26567,#26568,#26569,#26570,#26571,#26572,#26573,#26574,#26575,
#26576,#26577,#26578,#26579,#26580,#26581,#26582,#26583,#26584,#26585,#26586,
#26587,#26588,#26589,#26590,#26591,#26592,#26593,#26594,#26595,#26596,#26597,
#26598,#26599,#26600,#26601,#26602,#26603,#26604,#26605,#26606,#26607,#26608,
#26609,#26610));
#28461=AXIS2_PLACEMENT_3D('',#53157,#33829,#33830);
#28462=AXIS2_PLACEMENT_3D('',#53158,#33831,#33832);
#28463=AXIS2_PLACEMENT_3D('',#53270,#33834,#33835);
#28464=AXIS2_PLACEMENT_3D('',#53345,#33836,#33837);
#28465=AXIS2_PLACEMENT_3D('',#53643,#33839,#33840);
#28466=AXIS2_PLACEMENT_3D('',#53943,#33842,#33843);
#28467=AXIS2_PLACEMENT_3D('',#54233,#33845,#33846);
#28468=AXIS2_PLACEMENT_3D('',#54531,#33848,#33849);
#28469=AXIS2_PLACEMENT_3D('',#54823,#33851,#33852);
#28470=AXIS2_PLACEMENT_3D('',#55113,#33854,#33855);
#28471=AXIS2_PLACEMENT_3D('',#55175,#33856,#33857);
#28472=AXIS2_PLACEMENT_3D('',#56447,#33858,#33859);
#28473=AXIS2_PLACEMENT_3D('',#57519,#33860,#33861);
#28474=AXIS2_PLACEMENT_3D('',#57650,#33862,#33863);
#28475=AXIS2_PLACEMENT_3D('',#57747,#33864,#33865);
#28476=AXIS2_PLACEMENT_3D('',#57750,#33866,#33867);
#28477=AXIS2_PLACEMENT_3D('',#57920,#33868,#33869);
#28478=AXIS2_PLACEMENT_3D('',#58223,#33870,#33871);
#28479=AXIS2_PLACEMENT_3D('',#58226,#33872,#33873);
#28480=AXIS2_PLACEMENT_3D('',#58306,#33874,#33875);
#28481=AXIS2_PLACEMENT_3D('',#58519,#33876,#33877);
#28482=AXIS2_PLACEMENT_3D('',#58521,#33878,#33879);
#28483=AXIS2_PLACEMENT_3D('',#58522,#33880,#33881);
#28484=AXIS2_PLACEMENT_3D('',#58523,#33882,#33883);
#28485=AXIS2_PLACEMENT_3D('',#58525,#33884,#33885);
#28486=AXIS2_PLACEMENT_3D('',#58526,#33886,#33887);
#28487=AXIS2_PLACEMENT_3D('',#58529,#33889,#33890);
#28488=AXIS2_PLACEMENT_3D('',#58530,#33891,#33892);
#28489=AXIS2_PLACEMENT_3D('',#58531,#33893,#33894);
#28490=AXIS2_PLACEMENT_3D('',#58542,#33898,#33899);
#28491=AXIS2_PLACEMENT_3D('',#58550,#33902,#33903);
#28492=AXIS2_PLACEMENT_3D('',#58551,#33904,#33905);
#28493=AXIS2_PLACEMENT_3D('',#58552,#33906,#33907);
#28494=AXIS2_PLACEMENT_3D('',#58559,#33908,#33909);
#28495=AXIS2_PLACEMENT_3D('',#58569,#33910,#33911);
#28496=AXIS2_PLACEMENT_3D('',#58579,#33912,#33913);
#28497=AXIS2_PLACEMENT_3D('',#58589,#33914,#33915);
#28498=AXIS2_PLACEMENT_3D('',#58599,#33916,#33917);
#28499=AXIS2_PLACEMENT_3D('',#58609,#33918,#33919);
#28500=AXIS2_PLACEMENT_3D('',#58619,#33920,#33921);
#28501=AXIS2_PLACEMENT_3D('',#58629,#33922,#33923);
#28502=AXIS2_PLACEMENT_3D('',#58639,#33924,#33925);
#28503=AXIS2_PLACEMENT_3D('',#58649,#33926,#33927);
#28504=AXIS2_PLACEMENT_3D('',#58659,#33928,#33929);
#28505=AXIS2_PLACEMENT_3D('',#58669,#33930,#33931);
#28506=AXIS2_PLACEMENT_3D('',#58679,#33932,#33933);
#28507=AXIS2_PLACEMENT_3D('',#58689,#33934,#33935);
#28508=AXIS2_PLACEMENT_3D('',#58699,#33936,#33937);
#28509=AXIS2_PLACEMENT_3D('',#58709,#33938,#33939);
#28510=AXIS2_PLACEMENT_3D('',#58719,#33940,#33941);
#28511=AXIS2_PLACEMENT_3D('',#58729,#33942,#33943);
#28512=AXIS2_PLACEMENT_3D('',#58739,#33944,#33945);
#28513=AXIS2_PLACEMENT_3D('',#58749,#33946,#33947);
#28514=AXIS2_PLACEMENT_3D('',#58759,#33948,#33949);
#28515=AXIS2_PLACEMENT_3D('',#58769,#33950,#33951);
#28516=AXIS2_PLACEMENT_3D('',#58779,#33952,#33953);
#28517=AXIS2_PLACEMENT_3D('',#58789,#33954,#33955);
#28518=AXIS2_PLACEMENT_3D('',#58799,#33956,#33957);
#28519=AXIS2_PLACEMENT_3D('',#58809,#33958,#33959);
#28520=AXIS2_PLACEMENT_3D('',#58819,#33960,#33961);
#28521=AXIS2_PLACEMENT_3D('',#58828,#33962,#33963);
#28522=AXIS2_PLACEMENT_3D('',#58830,#33964,#33965);
#28523=AXIS2_PLACEMENT_3D('',#58840,#33966,#33967);
#28524=AXIS2_PLACEMENT_3D('',#58850,#33968,#33969);
#28525=AXIS2_PLACEMENT_3D('',#58860,#33970,#33971);
#28526=AXIS2_PLACEMENT_3D('',#58870,#33972,#33973);
#28527=AXIS2_PLACEMENT_3D('',#58880,#33974,#33975);
#28528=AXIS2_PLACEMENT_3D('',#58890,#33976,#33977);
#28529=AXIS2_PLACEMENT_3D('',#58900,#33978,#33979);
#28530=AXIS2_PLACEMENT_3D('',#58906,#33981,#33982);
#28531=AXIS2_PLACEMENT_3D('',#58907,#33983,#33984);
#28532=AXIS2_PLACEMENT_3D('',#58913,#33988,#33989);
#28533=AXIS2_PLACEMENT_3D('',#58917,#33992,#33993);
#28534=AXIS2_PLACEMENT_3D('',#58918,#33994,#33995);
#28535=AXIS2_PLACEMENT_3D('',#58919,#33996,#33997);
#28536=AXIS2_PLACEMENT_3D('',#58925,#34001,#34002);
#28537=AXIS2_PLACEMENT_3D('',#58929,#34005,#34006);
#28538=AXIS2_PLACEMENT_3D('',#58930,#34007,#34008);
#28539=AXIS2_PLACEMENT_3D('',#58931,#34009,#34010);
#28540=AXIS2_PLACEMENT_3D('',#58937,#34014,#34015);
#28541=AXIS2_PLACEMENT_3D('',#58941,#34018,#34019);
#28542=AXIS2_PLACEMENT_3D('',#58942,#34020,#34021);
#28543=AXIS2_PLACEMENT_3D('',#58943,#34022,#34023);
#28544=AXIS2_PLACEMENT_3D('',#58949,#34027,#34028);
#28545=AXIS2_PLACEMENT_3D('',#58953,#34031,#34032);
#28546=AXIS2_PLACEMENT_3D('',#58954,#34033,#34034);
#28547=AXIS2_PLACEMENT_3D('',#58955,#34035,#34036);
#28548=AXIS2_PLACEMENT_3D('',#58961,#34040,#34041);
#28549=AXIS2_PLACEMENT_3D('',#58965,#34044,#34045);
#28550=AXIS2_PLACEMENT_3D('',#58966,#34046,#34047);
#28551=AXIS2_PLACEMENT_3D('',#58967,#34048,#34049);
#28552=AXIS2_PLACEMENT_3D('',#58973,#34053,#34054);
#28553=AXIS2_PLACEMENT_3D('',#58977,#34057,#34058);
#28554=AXIS2_PLACEMENT_3D('',#58978,#34059,#34060);
#28555=AXIS2_PLACEMENT_3D('',#58979,#34061,#34062);
#28556=AXIS2_PLACEMENT_3D('',#58985,#34066,#34067);
#28557=AXIS2_PLACEMENT_3D('',#58989,#34070,#34071);
#28558=AXIS2_PLACEMENT_3D('',#58990,#34072,#34073);
#28559=AXIS2_PLACEMENT_3D('',#58991,#34074,#34075);
#28560=AXIS2_PLACEMENT_3D('',#58997,#34079,#34080);
#28561=AXIS2_PLACEMENT_3D('',#59001,#34083,#34084);
#28562=AXIS2_PLACEMENT_3D('',#59003,#34085,#34086);
#28563=AXIS2_PLACEMENT_3D('',#59004,#34087,#34088);
#28564=AXIS2_PLACEMENT_3D('',#59005,#34089,#34090);
#28565=AXIS2_PLACEMENT_3D('',#59011,#34094,#34095);
#28566=AXIS2_PLACEMENT_3D('',#59015,#34098,#34099);
#28567=AXIS2_PLACEMENT_3D('',#59016,#34100,#34101);
#28568=AXIS2_PLACEMENT_3D('',#59017,#34102,#34103);
#28569=AXIS2_PLACEMENT_3D('',#59023,#34107,#34108);
#28570=AXIS2_PLACEMENT_3D('',#59027,#34111,#34112);
#28571=AXIS2_PLACEMENT_3D('',#59028,#34113,#34114);
#28572=AXIS2_PLACEMENT_3D('',#59029,#34115,#34116);
#28573=AXIS2_PLACEMENT_3D('',#59035,#34120,#34121);
#28574=AXIS2_PLACEMENT_3D('',#59039,#34124,#34125);
#28575=AXIS2_PLACEMENT_3D('',#59040,#34126,#34127);
#28576=AXIS2_PLACEMENT_3D('',#59041,#34128,#34129);
#28577=AXIS2_PLACEMENT_3D('',#59047,#34133,#34134);
#28578=AXIS2_PLACEMENT_3D('',#59051,#34137,#34138);
#28579=AXIS2_PLACEMENT_3D('',#59052,#34139,#34140);
#28580=AXIS2_PLACEMENT_3D('',#59053,#34141,#34142);
#28581=AXIS2_PLACEMENT_3D('',#59059,#34146,#34147);
#28582=AXIS2_PLACEMENT_3D('',#59063,#34150,#34151);
#28583=AXIS2_PLACEMENT_3D('',#59064,#34152,#34153);
#28584=AXIS2_PLACEMENT_3D('',#59065,#34154,#34155);
#28585=AXIS2_PLACEMENT_3D('',#59071,#34159,#34160);
#28586=AXIS2_PLACEMENT_3D('',#59075,#34163,#34164);
#28587=AXIS2_PLACEMENT_3D('',#59076,#34165,#34166);
#28588=AXIS2_PLACEMENT_3D('',#59077,#34167,#34168);
#28589=AXIS2_PLACEMENT_3D('',#59083,#34172,#34173);
#28590=AXIS2_PLACEMENT_3D('',#59087,#34176,#34177);
#28591=AXIS2_PLACEMENT_3D('',#59088,#34178,#34179);
#28592=AXIS2_PLACEMENT_3D('',#59089,#34180,#34181);
#28593=AXIS2_PLACEMENT_3D('',#59095,#34185,#34186);
#28594=AXIS2_PLACEMENT_3D('',#59099,#34189,#34190);
#28595=AXIS2_PLACEMENT_3D('',#59100,#34191,#34192);
#28596=AXIS2_PLACEMENT_3D('',#59101,#34193,#34194);
#28597=AXIS2_PLACEMENT_3D('',#59107,#34198,#34199);
#28598=AXIS2_PLACEMENT_3D('',#59111,#34202,#34203);
#28599=AXIS2_PLACEMENT_3D('',#59112,#34204,#34205);
#28600=AXIS2_PLACEMENT_3D('',#59113,#34206,#34207);
#28601=AXIS2_PLACEMENT_3D('',#59119,#34211,#34212);
#28602=AXIS2_PLACEMENT_3D('',#59123,#34215,#34216);
#28603=AXIS2_PLACEMENT_3D('',#59124,#34217,#34218);
#28604=AXIS2_PLACEMENT_3D('',#59125,#34219,#34220);
#28605=AXIS2_PLACEMENT_3D('',#59131,#34224,#34225);
#28606=AXIS2_PLACEMENT_3D('',#59135,#34228,#34229);
#28607=AXIS2_PLACEMENT_3D('',#59136,#34230,#34231);
#28608=AXIS2_PLACEMENT_3D('',#59137,#34232,#34233);
#28609=AXIS2_PLACEMENT_3D('',#59143,#34237,#34238);
#28610=AXIS2_PLACEMENT_3D('',#59147,#34241,#34242);
#28611=AXIS2_PLACEMENT_3D('',#59148,#34243,#34244);
#28612=AXIS2_PLACEMENT_3D('',#59149,#34245,#34246);
#28613=AXIS2_PLACEMENT_3D('',#59155,#34250,#34251);
#28614=AXIS2_PLACEMENT_3D('',#59159,#34254,#34255);
#28615=AXIS2_PLACEMENT_3D('',#59160,#34256,#34257);
#28616=AXIS2_PLACEMENT_3D('',#59161,#34258,#34259);
#28617=AXIS2_PLACEMENT_3D('',#59167,#34263,#34264);
#28618=AXIS2_PLACEMENT_3D('',#59171,#34267,#34268);
#28619=AXIS2_PLACEMENT_3D('',#59172,#34269,#34270);
#28620=AXIS2_PLACEMENT_3D('',#59173,#34271,#34272);
#28621=AXIS2_PLACEMENT_3D('',#59179,#34276,#34277);
#28622=AXIS2_PLACEMENT_3D('',#59183,#34280,#34281);
#28623=AXIS2_PLACEMENT_3D('',#59184,#34282,#34283);
#28624=AXIS2_PLACEMENT_3D('',#59185,#34284,#34285);
#28625=AXIS2_PLACEMENT_3D('',#59191,#34289,#34290);
#28626=AXIS2_PLACEMENT_3D('',#59195,#34293,#34294);
#28627=AXIS2_PLACEMENT_3D('',#59196,#34295,#34296);
#28628=AXIS2_PLACEMENT_3D('',#59197,#34297,#34298);
#28629=AXIS2_PLACEMENT_3D('',#59203,#34302,#34303);
#28630=AXIS2_PLACEMENT_3D('',#59207,#34306,#34307);
#28631=AXIS2_PLACEMENT_3D('',#59208,#34308,#34309);
#28632=AXIS2_PLACEMENT_3D('',#59209,#34310,#34311);
#28633=AXIS2_PLACEMENT_3D('',#59215,#34315,#34316);
#28634=AXIS2_PLACEMENT_3D('',#59219,#34319,#34320);
#28635=AXIS2_PLACEMENT_3D('',#59220,#34321,#34322);
#28636=AXIS2_PLACEMENT_3D('',#59221,#34323,#34324);
#28637=AXIS2_PLACEMENT_3D('',#59227,#34328,#34329);
#28638=AXIS2_PLACEMENT_3D('',#59231,#34332,#34333);
#28639=AXIS2_PLACEMENT_3D('',#59232,#34334,#34335);
#28640=AXIS2_PLACEMENT_3D('',#59233,#34336,#34337);
#28641=AXIS2_PLACEMENT_3D('',#59239,#34341,#34342);
#28642=AXIS2_PLACEMENT_3D('',#59243,#34345,#34346);
#28643=AXIS2_PLACEMENT_3D('',#59244,#34347,#34348);
#28644=AXIS2_PLACEMENT_3D('',#59245,#34349,#34350);
#28645=AXIS2_PLACEMENT_3D('',#59251,#34354,#34355);
#28646=AXIS2_PLACEMENT_3D('',#59255,#34358,#34359);
#28647=AXIS2_PLACEMENT_3D('',#59256,#34360,#34361);
#28648=AXIS2_PLACEMENT_3D('',#59257,#34362,#34363);
#28649=AXIS2_PLACEMENT_3D('',#59263,#34367,#34368);
#28650=AXIS2_PLACEMENT_3D('',#59267,#34371,#34372);
#28651=AXIS2_PLACEMENT_3D('',#59268,#34373,#34374);
#28652=AXIS2_PLACEMENT_3D('',#59269,#34375,#34376);
#28653=AXIS2_PLACEMENT_3D('',#59275,#34380,#34381);
#28654=AXIS2_PLACEMENT_3D('',#59279,#34384,#34385);
#28655=AXIS2_PLACEMENT_3D('',#59280,#34386,#34387);
#28656=AXIS2_PLACEMENT_3D('',#59281,#34388,#34389);
#28657=AXIS2_PLACEMENT_3D('',#59287,#34393,#34394);
#28658=AXIS2_PLACEMENT_3D('',#59291,#34397,#34398);
#28659=AXIS2_PLACEMENT_3D('',#59292,#34399,#34400);
#28660=AXIS2_PLACEMENT_3D('',#59293,#34401,#34402);
#28661=AXIS2_PLACEMENT_3D('',#59299,#34406,#34407);
#28662=AXIS2_PLACEMENT_3D('',#59303,#34410,#34411);
#28663=AXIS2_PLACEMENT_3D('',#59304,#34412,#34413);
#28664=AXIS2_PLACEMENT_3D('',#59305,#34414,#34415);
#28665=AXIS2_PLACEMENT_3D('',#59311,#34419,#34420);
#28666=AXIS2_PLACEMENT_3D('',#59315,#34423,#34424);
#28667=AXIS2_PLACEMENT_3D('',#59316,#34425,#34426);
#28668=AXIS2_PLACEMENT_3D('',#59317,#34427,#34428);
#28669=AXIS2_PLACEMENT_3D('',#59323,#34432,#34433);
#28670=AXIS2_PLACEMENT_3D('',#59327,#34436,#34437);
#28671=AXIS2_PLACEMENT_3D('',#59328,#34438,#34439);
#28672=AXIS2_PLACEMENT_3D('',#59329,#34440,#34441);
#28673=AXIS2_PLACEMENT_3D('',#59331,#34443,#34444);
#28674=AXIS2_PLACEMENT_3D('',#59344,#34451,#34452);
#28675=AXIS2_PLACEMENT_3D('',#59348,#34454,#34455);
#28676=AXIS2_PLACEMENT_3D('',#59349,#34456,#34457);
#28677=AXIS2_PLACEMENT_3D('',#59352,#34459,#34460);
#28678=AXIS2_PLACEMENT_3D('',#59353,#34461,#34462);
#28679=AXIS2_PLACEMENT_3D('',#59356,#34464,#34465);
#28680=AXIS2_PLACEMENT_3D('',#59357,#34466,#34467);
#28681=AXIS2_PLACEMENT_3D('',#59360,#34469,#34470);
#28682=AXIS2_PLACEMENT_3D('',#59361,#34471,#34472);
#28683=AXIS2_PLACEMENT_3D('',#59364,#34474,#34475);
#28684=AXIS2_PLACEMENT_3D('',#59365,#34476,#34477);
#28685=AXIS2_PLACEMENT_3D('',#59367,#34479,#34480);
#28686=AXIS2_PLACEMENT_3D('',#59368,#34481,#34482);
#28687=AXIS2_PLACEMENT_3D('',#59371,#34484,#34485);
#28688=AXIS2_PLACEMENT_3D('',#59374,#34488,#34489);
#28689=AXIS2_PLACEMENT_3D('',#59376,#34491,#34492);
#28690=AXIS2_PLACEMENT_3D('',#59378,#34494,#34495);
#28691=AXIS2_PLACEMENT_3D('',#59380,#34497,#34498);
#28692=AXIS2_PLACEMENT_3D('',#59382,#34500,#34501);
#33829=DIRECTION('axis',(0.,0.,1.));
#33830=DIRECTION('refdir',(1.,0.,0.));
#33831=DIRECTION('center_axis',(-1.,0.,0.));
#33832=DIRECTION('ref_axis',(0.,0.756725241443425,-0.653733056348224));
#33833=DIRECTION('',(1.,0.,0.));
#33834=DIRECTION('center_axis',(1.,0.,0.));
#33835=DIRECTION('ref_axis',(0.,-2.79741234551221E-14,-1.));
#33836=DIRECTION('center_axis',(-1.,0.,0.));
#33837=DIRECTION('ref_axis',(0.,0.756725241443425,-0.653733056348224));
#33838=DIRECTION('',(1.,0.,0.));
#33839=DIRECTION('center_axis',(-1.,0.,0.));
#33840=DIRECTION('ref_axis',(0.,0.756725241443425,-0.653733056348224));
#33841=DIRECTION('',(1.,0.,0.));
#33842=DIRECTION('center_axis',(-1.,0.,0.));
#33843=DIRECTION('ref_axis',(0.,0.756725241443425,-0.653733056348224));
#33844=DIRECTION('',(1.,0.,0.));
#33845=DIRECTION('center_axis',(-1.,0.,0.));
#33846=DIRECTION('ref_axis',(0.,0.756725241443425,-0.653733056348224));
#33847=DIRECTION('',(1.,0.,0.));
#33848=DIRECTION('center_axis',(-1.,0.,0.));
#33849=DIRECTION('ref_axis',(0.,0.756725241443425,-0.653733056348224));
#33850=DIRECTION('',(1.,0.,0.));
#33851=DIRECTION('center_axis',(-1.,0.,0.));
#33852=DIRECTION('ref_axis',(0.,0.756725241443425,-0.653733056348224));
#33853=DIRECTION('',(1.,0.,0.));
#33854=DIRECTION('center_axis',(-1.,0.,0.));
#33855=DIRECTION('ref_axis',(0.,0.,-1.));
#33856=DIRECTION('center_axis',(1.,0.,0.));
#33857=DIRECTION('ref_axis',(0.,0.,-1.));
#33858=DIRECTION('center_axis',(-1.,0.,0.));
#33859=DIRECTION('ref_axis',(0.,0.,-1.));
#33860=DIRECTION('center_axis',(-1.,0.,0.));
#33861=DIRECTION('ref_axis',(0.,0.961400218503714,-0.275153811278367));
#33862=DIRECTION('center_axis',(-1.,0.,0.));
#33863=DIRECTION('ref_axis',(0.,-2.79741234551221E-14,-1.));
#33864=DIRECTION('center_axis',(1.,0.,0.));
#33865=DIRECTION('ref_axis',(0.,0.,-1.));
#33866=DIRECTION('center_axis',(-1.,0.,0.));
#33867=DIRECTION('ref_axis',(0.,0.,-1.));
#33868=DIRECTION('center_axis',(-1.,0.,0.));
#33869=DIRECTION('ref_axis',(0.,0.,-1.));
#33870=DIRECTION('center_axis',(1.,0.,0.));
#33871=DIRECTION('ref_axis',(0.,0.,-1.));
#33872=DIRECTION('center_axis',(1.,0.,0.));
#33873=DIRECTION('ref_axis',(0.,0.,-1.));
#33874=DIRECTION('center_axis',(1.,0.,0.));
#33875=DIRECTION('ref_axis',(0.,0.,-1.));
#33876=DIRECTION('center_axis',(1.,0.,0.));
#33877=DIRECTION('ref_axis',(0.,0.,-1.));
#33878=DIRECTION('center_axis',(-1.,0.,0.));
#33879=DIRECTION('ref_axis',(0.,0.,-1.));
#33880=DIRECTION('center_axis',(0.,1.,0.));
#33881=DIRECTION('ref_axis',(0.,0.,1.));
#33882=DIRECTION('center_axis',(1.,0.,0.));
#33883=DIRECTION('ref_axis',(0.,0.,-1.));
#33884=DIRECTION('center_axis',(1.,0.,0.));
#33885=DIRECTION('ref_axis',(0.,0.,-1.));
#33886=DIRECTION('center_axis',(1.,0.,0.));
#33887=DIRECTION('ref_axis',(0.,0.,-1.));
#33888=DIRECTION('',(-0.707106781186548,8.65956056235493E-17,-0.707106781186547));
#33889=DIRECTION('center_axis',(1.,0.,0.));
#33890=DIRECTION('ref_axis',(0.,0.,-1.));
#33891=DIRECTION('center_axis',(1.,0.,0.));
#33892=DIRECTION('ref_axis',(0.,0.,-1.));
#33893=DIRECTION('center_axis',(0.,-0.188314866426192,-0.982108706347157));
#33894=DIRECTION('ref_axis',(0.,-0.982108706347157,0.188314866426192));
#33895=DIRECTION('',(1.,0.,0.));
#33896=DIRECTION('',(0.,-0.982108706347157,0.188314866426192));
#33897=DIRECTION('',(-1.,0.,0.));
#33898=DIRECTION('center_axis',(0.,-0.512859050871219,0.858472826558577));
#33899=DIRECTION('ref_axis',(0.,0.858472826558577,0.512859050871219));
#33900=DIRECTION('',(-1.,0.,0.));
#33901=DIRECTION('',(0.,0.858472826558577,0.512859050871219));
#33902=DIRECTION('center_axis',(-1.,0.,0.));
#33903=DIRECTION('ref_axis',(0.,-0.17364817766693,0.984807753012208));
#33904=DIRECTION('center_axis',(-1.,0.,0.));
#33905=DIRECTION('ref_axis',(0.,0.,-1.));
#33906=DIRECTION('center_axis',(-1.,0.,0.));
#33907=DIRECTION('ref_axis',(0.,0.,-1.));
#33908=DIRECTION('center_axis',(1.,0.,0.));
#33909=DIRECTION('ref_axis',(0.,0.,-1.));
#33910=DIRECTION('center_axis',(1.,0.,0.));
#33911=DIRECTION('ref_axis',(0.,0.,-1.));
#33912=DIRECTION('center_axis',(1.,0.,0.));
#33913=DIRECTION('ref_axis',(0.,0.,-1.));
#33914=DIRECTION('center_axis',(1.,0.,0.));
#33915=DIRECTION('ref_axis',(0.,0.,-1.));
#33916=DIRECTION('center_axis',(1.,0.,0.));
#33917=DIRECTION('ref_axis',(0.,0.,-1.));
#33918=DIRECTION('center_axis',(1.,0.,0.));
#33919=DIRECTION('ref_axis',(0.,0.,-1.));
#33920=DIRECTION('center_axis',(1.,0.,0.));
#33921=DIRECTION('ref_axis',(0.,0.,-1.));
#33922=DIRECTION('center_axis',(1.,0.,0.));
#33923=DIRECTION('ref_axis',(0.,0.,-1.));
#33924=DIRECTION('center_axis',(1.,0.,0.));
#33925=DIRECTION('ref_axis',(0.,0.,-1.));
#33926=DIRECTION('center_axis',(1.,0.,0.));
#33927=DIRECTION('ref_axis',(0.,0.,-1.));
#33928=DIRECTION('center_axis',(1.,0.,0.));
#33929=DIRECTION('ref_axis',(0.,0.,-1.));
#33930=DIRECTION('center_axis',(1.,0.,0.));
#33931=DIRECTION('ref_axis',(0.,0.,-1.));
#33932=DIRECTION('center_axis',(1.,0.,0.));
#33933=DIRECTION('ref_axis',(0.,0.,-1.));
#33934=DIRECTION('center_axis',(1.,0.,0.));
#33935=DIRECTION('ref_axis',(0.,0.,-1.));
#33936=DIRECTION('center_axis',(1.,0.,0.));
#33937=DIRECTION('ref_axis',(0.,0.,-1.));
#33938=DIRECTION('center_axis',(1.,0.,0.));
#33939=DIRECTION('ref_axis',(0.,0.,-1.));
#33940=DIRECTION('center_axis',(1.,0.,0.));
#33941=DIRECTION('ref_axis',(0.,0.,-1.));
#33942=DIRECTION('center_axis',(1.,0.,0.));
#33943=DIRECTION('ref_axis',(0.,0.,-1.));
#33944=DIRECTION('center_axis',(1.,0.,0.));
#33945=DIRECTION('ref_axis',(0.,0.,-1.));
#33946=DIRECTION('center_axis',(1.,0.,0.));
#33947=DIRECTION('ref_axis',(0.,0.,-1.));
#33948=DIRECTION('center_axis',(1.,0.,0.));
#33949=DIRECTION('ref_axis',(0.,0.,-1.));
#33950=DIRECTION('center_axis',(1.,0.,0.));
#33951=DIRECTION('ref_axis',(0.,0.,-1.));
#33952=DIRECTION('center_axis',(1.,0.,0.));
#33953=DIRECTION('ref_axis',(0.,0.,-1.));
#33954=DIRECTION('center_axis',(1.,0.,0.));
#33955=DIRECTION('ref_axis',(0.,0.,-1.));
#33956=DIRECTION('center_axis',(1.,0.,0.));
#33957=DIRECTION('ref_axis',(0.,0.,-1.));
#33958=DIRECTION('center_axis',(1.,0.,0.));
#33959=DIRECTION('ref_axis',(0.,0.,-1.));
#33960=DIRECTION('center_axis',(1.,0.,0.));
#33961=DIRECTION('ref_axis',(0.,0.,-1.));
#33962=DIRECTION('center_axis',(1.,0.,0.));
#33963=DIRECTION('ref_axis',(0.,0.,-1.));
#33964=DIRECTION('center_axis',(1.,0.,0.));
#33965=DIRECTION('ref_axis',(0.,0.,-1.));
#33966=DIRECTION('center_axis',(1.,0.,0.));
#33967=DIRECTION('ref_axis',(0.,0.,-1.));
#33968=DIRECTION('center_axis',(1.,0.,0.));
#33969=DIRECTION('ref_axis',(0.,0.,-1.));
#33970=DIRECTION('center_axis',(1.,0.,0.));
#33971=DIRECTION('ref_axis',(0.,0.,-1.));
#33972=DIRECTION('center_axis',(1.,0.,0.));
#33973=DIRECTION('ref_axis',(0.,0.,-1.));
#33974=DIRECTION('center_axis',(1.,0.,0.));
#33975=DIRECTION('ref_axis',(0.,0.,-1.));
#33976=DIRECTION('center_axis',(1.,0.,0.));
#33977=DIRECTION('ref_axis',(0.,0.,-1.));
#33978=DIRECTION('center_axis',(1.,0.,0.));
#33979=DIRECTION('ref_axis',(0.,0.,-1.));
#33980=DIRECTION('',(0.707106781186545,-8.65956056235496E-17,-0.70710678118655));
#33981=DIRECTION('center_axis',(-1.,0.,0.));
#33982=DIRECTION('ref_axis',(0.,0.,-1.));
#33983=DIRECTION('center_axis',(0.,-0.0149125533359619,-0.999888801693969));
#33984=DIRECTION('ref_axis',(0.,-0.999888801693969,0.0149125533359619));
#33985=DIRECTION('',(1.,0.,0.));
#33986=DIRECTION('',(0.,-0.999888801693969,0.0149125533359619));
#33987=DIRECTION('',(-1.,0.,0.));
#33988=DIRECTION('center_axis',(0.,-0.654139811408935,0.756373655761412));
#33989=DIRECTION('ref_axis',(0.,0.756373655761412,0.654139811408935));
#33990=DIRECTION('',(-1.,0.,0.));
#33991=DIRECTION('',(0.,0.756373655761412,0.654139811408935));
#33992=DIRECTION('center_axis',(-1.,0.,0.));
#33993=DIRECTION('ref_axis',(0.,-0.342020143325669,0.939692620785908));
#33994=DIRECTION('center_axis',(-1.,0.,0.));
#33995=DIRECTION('ref_axis',(0.,0.,-1.));
#33996=DIRECTION('center_axis',(0.,0.158942870141265,-0.987287781769458));
#33997=DIRECTION('ref_axis',(0.,-0.987287781769458,-0.158942870141265));
#33998=DIRECTION('',(1.,0.,0.));
#33999=DIRECTION('',(0.,-0.987287781769458,-0.158942870141265));
#34000=DIRECTION('',(-1.,0.,0.));
#34001=DIRECTION('center_axis',(0.,-0.775544864787706,0.631292454177475));
#34002=DIRECTION('ref_axis',(0.,0.631292454177475,0.775544864787706));
#34003=DIRECTION('',(-1.,0.,0.));
#34004=DIRECTION('',(0.,0.631292454177475,0.775544864787706));
#34005=DIRECTION('center_axis',(-1.,0.,0.));
#34006=DIRECTION('ref_axis',(0.,-0.5,0.866025403784438));
#34007=DIRECTION('center_axis',(-1.,0.,0.));
#34008=DIRECTION('ref_axis',(0.,0.,-1.));
#34009=DIRECTION('center_axis',(0.,0.327968894938223,-0.944688522187605));
#34010=DIRECTION('ref_axis',(0.,-0.944688522187605,-0.327968894938223));
#34011=DIRECTION('',(1.,0.,0.));
#34012=DIRECTION('',(0.,-0.944688522187605,-0.327968894938223));
#34013=DIRECTION('',(-1.,0.,0.));
#34014=DIRECTION('center_axis',(0.,-0.87338537989454,0.48702975082275));
#34015=DIRECTION('ref_axis',(0.,0.48702975082275,0.87338537989454));
#34016=DIRECTION('',(-1.,0.,0.));
#34017=DIRECTION('',(0.,0.48702975082275,0.87338537989454));
#34018=DIRECTION('center_axis',(-1.,0.,0.));
#34019=DIRECTION('ref_axis',(0.,-0.64278760968654,0.766044443118978));
#34020=DIRECTION('center_axis',(-1.,0.,0.));
#34021=DIRECTION('ref_axis',(0.,0.,-1.));
#34022=DIRECTION('center_axis',(0.,0.487029750822751,-0.87338537989454));
#34023=DIRECTION('ref_axis',(0.,-0.87338537989454,-0.487029750822751));
#34024=DIRECTION('',(1.,0.,0.));
#34025=DIRECTION('',(0.,-0.87338537989454,-0.487029750822751));
#34026=DIRECTION('',(-1.,0.,0.));
#34027=DIRECTION('center_axis',(0.,-0.944688522187605,0.327968894938222));
#34028=DIRECTION('ref_axis',(0.,0.327968894938222,0.944688522187605));
#34029=DIRECTION('',(-1.,0.,0.));
#34030=DIRECTION('',(0.,0.327968894938222,0.944688522187605));
#34031=DIRECTION('center_axis',(-1.,0.,0.));
#34032=DIRECTION('ref_axis',(0.,-0.766044443118978,0.642787609686539));
#34033=DIRECTION('center_axis',(-1.,0.,0.));
#34034=DIRECTION('ref_axis',(0.,0.,-1.));
#34035=DIRECTION('center_axis',(0.,0.631292454177475,-0.775544864787706));
#34036=DIRECTION('ref_axis',(0.,-0.775544864787706,-0.631292454177475));
#34037=DIRECTION('',(1.,0.,0.));
#34038=DIRECTION('',(0.,-0.775544864787705,-0.631292454177475));
#34039=DIRECTION('',(-1.,0.,0.));
#34040=DIRECTION('center_axis',(0.,-0.987287781769458,0.158942870141265));
#34041=DIRECTION('ref_axis',(0.,0.158942870141265,0.987287781769458));
#34042=DIRECTION('',(-1.,0.,0.));
#34043=DIRECTION('',(0.,0.158942870141265,0.987287781769458));
#34044=DIRECTION('center_axis',(-1.,0.,0.));
#34045=DIRECTION('ref_axis',(0.,-0.866025403784439,0.5));
#34046=DIRECTION('center_axis',(-1.,0.,0.));
#34047=DIRECTION('ref_axis',(0.,0.,-1.));
#34048=DIRECTION('center_axis',(0.,0.756373655761413,-0.654139811408934));
#34049=DIRECTION('ref_axis',(0.,-0.654139811408934,-0.756373655761413));
#34050=DIRECTION('',(1.,0.,0.));
#34051=DIRECTION('',(0.,-0.654139811408934,-0.756373655761413));
#34052=DIRECTION('',(-1.,0.,0.));
#34053=DIRECTION('center_axis',(0.,-0.999888801693969,-0.0149125533359631));
#34054=DIRECTION('ref_axis',(0.,-0.0149125533359631,0.999888801693969));
#34055=DIRECTION('',(-1.,0.,0.));
#34056=DIRECTION('',(0.,-0.0149125533359631,0.999888801693969));
#34057=DIRECTION('center_axis',(-1.,0.,0.));
#34058=DIRECTION('ref_axis',(0.,-0.939692620785909,0.342020143325668));
#34059=DIRECTION('center_axis',(-1.,0.,0.));
#34060=DIRECTION('ref_axis',(0.,0.,-1.));
#34061=DIRECTION('center_axis',(0.,0.858472826558577,-0.512859050871218));
#34062=DIRECTION('ref_axis',(0.,-0.512859050871218,-0.858472826558577));
#34063=DIRECTION('',(1.,0.,0.));
#34064=DIRECTION('',(0.,-0.512859050871218,-0.858472826558577));
#34065=DIRECTION('',(-1.,0.,0.));
#34066=DIRECTION('center_axis',(0.,-0.982108706347157,-0.188314866426193));
#34067=DIRECTION('ref_axis',(0.,-0.188314866426193,0.982108706347157));
#34068=DIRECTION('',(-1.,0.,0.));
#34069=DIRECTION('',(0.,-0.188314866426193,0.982108706347156));
#34070=DIRECTION('center_axis',(-1.,0.,0.));
#34071=DIRECTION('ref_axis',(0.,-0.984807753012208,0.17364817766693));
#34072=DIRECTION('center_axis',(-1.,0.,0.));
#34073=DIRECTION('ref_axis',(0.,0.,-1.));
#34074=DIRECTION('center_axis',(0.,0.93448773492897,-0.355995327591983));
#34075=DIRECTION('ref_axis',(0.,-0.355995327591983,-0.93448773492897));
#34076=DIRECTION('',(1.,0.,0.));
#34077=DIRECTION('',(0.,-0.355995327591983,-0.93448773492897));
#34078=DIRECTION('',(-1.,0.,0.));
#34079=DIRECTION('center_axis',(0.,-0.93448773492897,-0.355995327591983));
#34080=DIRECTION('ref_axis',(0.,-0.355995327591983,0.93448773492897));
#34081=DIRECTION('',(-1.,0.,0.));
#34082=DIRECTION('',(0.,-0.355995327591983,0.93448773492897));
#34083=DIRECTION('center_axis',(-1.,0.,0.));
#34084=DIRECTION('ref_axis',(0.,-1.,-1.83697019872103E-16));
#34085=DIRECTION('center_axis',(-1.,0.,0.));
#34086=DIRECTION('ref_axis',(0.,0.,-1.));
#34087=DIRECTION('center_axis',(-1.,0.,0.));
#34088=DIRECTION('ref_axis',(0.,0.,-1.));
#34089=DIRECTION('center_axis',(0.,0.982108706347157,-0.188314866426193));
#34090=DIRECTION('ref_axis',(0.,-0.188314866426193,-0.982108706347156));
#34091=DIRECTION('',(1.,0.,0.));
#34092=DIRECTION('',(0.,-0.188314866426193,-0.982108706347156));
#34093=DIRECTION('',(-1.,0.,0.));
#34094=DIRECTION('center_axis',(0.,-0.858472826558577,-0.512859050871219));
#34095=DIRECTION('ref_axis',(0.,-0.512859050871219,0.858472826558577));
#34096=DIRECTION('',(-1.,0.,0.));
#34097=DIRECTION('',(0.,-0.512859050871219,0.858472826558577));
#34098=DIRECTION('center_axis',(-1.,0.,0.));
#34099=DIRECTION('ref_axis',(0.,-0.984807753012208,-0.17364817766693));
#34100=DIRECTION('center_axis',(-1.,0.,0.));
#34101=DIRECTION('ref_axis',(0.,0.,-1.));
#34102=DIRECTION('center_axis',(0.,0.99988880169397,-0.014912553335962));
#34103=DIRECTION('ref_axis',(0.,-0.014912553335962,-0.99988880169397));
#34104=DIRECTION('',(1.,0.,0.));
#34105=DIRECTION('',(0.,-0.014912553335962,-0.999888801693969));
#34106=DIRECTION('',(-1.,0.,0.));
#34107=DIRECTION('center_axis',(0.,-0.756373655761412,-0.654139811408935));
#34108=DIRECTION('ref_axis',(0.,-0.654139811408935,0.756373655761412));
#34109=DIRECTION('',(-1.,0.,0.));
#34110=DIRECTION('',(0.,-0.654139811408935,0.756373655761412));
#34111=DIRECTION('center_axis',(-1.,0.,0.));
#34112=DIRECTION('ref_axis',(0.,-0.939692620785908,-0.342020143325669));
#34113=DIRECTION('center_axis',(-1.,0.,0.));
#34114=DIRECTION('ref_axis',(0.,0.,-1.));
#34115=DIRECTION('center_axis',(0.,0.987287781769458,0.158942870141265));
#34116=DIRECTION('ref_axis',(0.,0.158942870141265,-0.987287781769458));
#34117=DIRECTION('',(1.,0.,0.));
#34118=DIRECTION('',(0.,0.158942870141265,-0.987287781769458));
#34119=DIRECTION('',(-1.,0.,0.));
#34120=DIRECTION('center_axis',(0.,-0.631292454177475,-0.775544864787706));
#34121=DIRECTION('ref_axis',(0.,-0.775544864787706,0.631292454177475));
#34122=DIRECTION('',(-1.,0.,0.));
#34123=DIRECTION('',(0.,-0.775544864787706,0.631292454177475));
#34124=DIRECTION('center_axis',(-1.,0.,0.));
#34125=DIRECTION('ref_axis',(0.,-0.866025403784438,-0.5));
#34126=DIRECTION('center_axis',(-1.,0.,0.));
#34127=DIRECTION('ref_axis',(0.,0.,-1.));
#34128=DIRECTION('center_axis',(0.,0.944688522187605,0.327968894938222));
#34129=DIRECTION('ref_axis',(0.,0.327968894938222,-0.944688522187605));
#34130=DIRECTION('',(1.,0.,0.));
#34131=DIRECTION('',(0.,0.327968894938222,-0.944688522187605));
#34132=DIRECTION('',(-1.,0.,0.));
#34133=DIRECTION('center_axis',(0.,-0.487029750822751,-0.87338537989454));
#34134=DIRECTION('ref_axis',(0.,-0.87338537989454,0.487029750822751));
#34135=DIRECTION('',(-1.,0.,0.));
#34136=DIRECTION('',(0.,-0.87338537989454,0.487029750822751));
#34137=DIRECTION('center_axis',(-1.,0.,0.));
#34138=DIRECTION('ref_axis',(0.,-0.766044443118978,-0.642787609686539));
#34139=DIRECTION('center_axis',(-1.,0.,0.));
#34140=DIRECTION('ref_axis',(0.,0.,-1.));
#34141=DIRECTION('center_axis',(0.,0.87338537989454,0.487029750822751));
#34142=DIRECTION('ref_axis',(0.,0.487029750822751,-0.87338537989454));
#34143=DIRECTION('',(1.,0.,0.));
#34144=DIRECTION('',(0.,0.487029750822751,-0.87338537989454));
#34145=DIRECTION('',(-1.,0.,0.));
#34146=DIRECTION('center_axis',(0.,-0.327968894938222,-0.944688522187605));
#34147=DIRECTION('ref_axis',(0.,-0.944688522187605,0.327968894938222));
#34148=DIRECTION('',(-1.,0.,0.));
#34149=DIRECTION('',(0.,-0.944688522187605,0.327968894938222));
#34150=DIRECTION('center_axis',(-1.,0.,0.));
#34151=DIRECTION('ref_axis',(0.,-0.642787609686539,-0.766044443118978));
#34152=DIRECTION('center_axis',(-1.,0.,0.));
#34153=DIRECTION('ref_axis',(0.,0.,-1.));
#34154=DIRECTION('center_axis',(0.,0.775544864787705,0.631292454177475));
#34155=DIRECTION('ref_axis',(0.,0.631292454177475,-0.775544864787705));
#34156=DIRECTION('',(1.,0.,0.));
#34157=DIRECTION('',(0.,0.631292454177475,-0.775544864787705));
#34158=DIRECTION('',(-1.,0.,0.));
#34159=DIRECTION('center_axis',(0.,-0.158942870141264,-0.987287781769458));
#34160=DIRECTION('ref_axis',(0.,-0.987287781769458,0.158942870141264));
#34161=DIRECTION('',(-1.,0.,0.));
#34162=DIRECTION('',(0.,-0.987287781769458,0.158942870141264));
#34163=DIRECTION('center_axis',(-1.,0.,0.));
#34164=DIRECTION('ref_axis',(0.,-0.5,-0.866025403784439));
#34165=DIRECTION('center_axis',(-1.,0.,0.));
#34166=DIRECTION('ref_axis',(0.,0.,-1.));
#34167=DIRECTION('center_axis',(0.,0.654139811408934,0.756373655761413));
#34168=DIRECTION('ref_axis',(0.,0.756373655761413,-0.654139811408934));
#34169=DIRECTION('',(1.,0.,0.));
#34170=DIRECTION('',(0.,0.756373655761413,-0.654139811408934));
#34171=DIRECTION('',(-1.,0.,0.));
#34172=DIRECTION('center_axis',(0.,0.0149125533359627,-0.99988880169397));
#34173=DIRECTION('ref_axis',(0.,-0.99988880169397,-0.0149125533359627));
#34174=DIRECTION('',(-1.,0.,0.));
#34175=DIRECTION('',(0.,-0.999888801693969,-0.0149125533359627));
#34176=DIRECTION('center_axis',(-1.,0.,0.));
#34177=DIRECTION('ref_axis',(0.,-0.342020143325669,-0.939692620785908));
#34178=DIRECTION('center_axis',(-1.,0.,0.));
#34179=DIRECTION('ref_axis',(0.,0.,-1.));
#34180=DIRECTION('center_axis',(0.,0.512859050871218,0.858472826558577));
#34181=DIRECTION('ref_axis',(0.,0.858472826558577,-0.512859050871218));
#34182=DIRECTION('',(1.,0.,0.));
#34183=DIRECTION('',(0.,0.858472826558577,-0.512859050871218));
#34184=DIRECTION('',(-1.,0.,0.));
#34185=DIRECTION('center_axis',(0.,0.188314866426193,-0.982108706347157));
#34186=DIRECTION('ref_axis',(0.,-0.982108706347157,-0.188314866426193));
#34187=DIRECTION('',(-1.,0.,0.));
#34188=DIRECTION('',(0.,-0.982108706347156,-0.188314866426193));
#34189=DIRECTION('center_axis',(-1.,0.,0.));
#34190=DIRECTION('ref_axis',(0.,-0.17364817766693,-0.984807753012208));
#34191=DIRECTION('center_axis',(-1.,0.,0.));
#34192=DIRECTION('ref_axis',(0.,0.,-1.));
#34193=DIRECTION('center_axis',(0.,0.355995327591983,0.93448773492897));
#34194=DIRECTION('ref_axis',(0.,0.93448773492897,-0.355995327591983));
#34195=DIRECTION('',(1.,0.,0.));
#34196=DIRECTION('',(0.,0.93448773492897,-0.355995327591983));
#34197=DIRECTION('',(-1.,0.,0.));
#34198=DIRECTION('center_axis',(0.,0.355995327591983,-0.93448773492897));
#34199=DIRECTION('ref_axis',(0.,-0.93448773492897,-0.355995327591983));
#34200=DIRECTION('',(-1.,0.,0.));
#34201=DIRECTION('',(0.,-0.93448773492897,-0.355995327591983));
#34202=DIRECTION('center_axis',(-1.,0.,0.));
#34203=DIRECTION('ref_axis',(0.,1.22464679914735E-16,-1.));
#34204=DIRECTION('center_axis',(-1.,0.,0.));
#34205=DIRECTION('ref_axis',(0.,0.,-1.));
#34206=DIRECTION('center_axis',(0.,0.188314866426192,0.982108706347157));
#34207=DIRECTION('ref_axis',(0.,0.982108706347157,-0.188314866426192));
#34208=DIRECTION('',(1.,0.,0.));
#34209=DIRECTION('',(0.,0.982108706347157,-0.188314866426192));
#34210=DIRECTION('',(-1.,0.,0.));
#34211=DIRECTION('center_axis',(0.,0.512859050871219,-0.858472826558577));
#34212=DIRECTION('ref_axis',(0.,-0.858472826558577,-0.512859050871219));
#34213=DIRECTION('',(-1.,0.,0.));
#34214=DIRECTION('',(0.,-0.858472826558577,-0.512859050871219));
#34215=DIRECTION('center_axis',(-1.,0.,0.));
#34216=DIRECTION('ref_axis',(0.,0.173648177666931,-0.984807753012208));
#34217=DIRECTION('center_axis',(-1.,0.,0.));
#34218=DIRECTION('ref_axis',(0.,0.,-1.));
#34219=DIRECTION('center_axis',(0.,0.0149125533359624,0.99988880169397));
#34220=DIRECTION('ref_axis',(0.,0.99988880169397,-0.0149125533359624));
#34221=DIRECTION('',(1.,0.,0.));
#34222=DIRECTION('',(0.,0.999888801693969,-0.0149125533359624));
#34223=DIRECTION('',(-1.,0.,0.));
#34224=DIRECTION('center_axis',(0.,0.654139811408934,-0.756373655761413));
#34225=DIRECTION('ref_axis',(0.,-0.756373655761413,-0.654139811408935));
#34226=DIRECTION('',(-1.,0.,0.));
#34227=DIRECTION('',(0.,-0.756373655761413,-0.654139811408934));
#34228=DIRECTION('center_axis',(-1.,0.,0.));
#34229=DIRECTION('ref_axis',(0.,0.342020143325669,-0.939692620785908));
#34230=DIRECTION('center_axis',(-1.,0.,0.));
#34231=DIRECTION('ref_axis',(0.,0.,-1.));
#34232=DIRECTION('center_axis',(0.,-0.158942870141264,0.987287781769458));
#34233=DIRECTION('ref_axis',(0.,0.987287781769458,0.158942870141264));
#34234=DIRECTION('',(1.,0.,0.));
#34235=DIRECTION('',(0.,0.987287781769458,0.158942870141264));
#34236=DIRECTION('',(-1.,0.,0.));
#34237=DIRECTION('center_axis',(0.,0.775544864787705,-0.631292454177475));
#34238=DIRECTION('ref_axis',(0.,-0.631292454177475,-0.775544864787705));
#34239=DIRECTION('',(-1.,0.,0.));
#34240=DIRECTION('',(0.,-0.631292454177475,-0.775544864787705));
#34241=DIRECTION('center_axis',(-1.,0.,0.));
#34242=DIRECTION('ref_axis',(0.,0.5,-0.866025403784439));
#34243=DIRECTION('center_axis',(-1.,0.,0.));
#34244=DIRECTION('ref_axis',(0.,0.,-1.));
#34245=DIRECTION('center_axis',(0.,-0.327968894938222,0.944688522187605));
#34246=DIRECTION('ref_axis',(0.,0.944688522187605,0.327968894938222));
#34247=DIRECTION('',(1.,0.,0.));
#34248=DIRECTION('',(0.,0.944688522187605,0.327968894938222));
#34249=DIRECTION('',(-1.,0.,0.));
#34250=DIRECTION('center_axis',(0.,0.87338537989454,-0.487029750822751));
#34251=DIRECTION('ref_axis',(0.,-0.487029750822751,-0.87338537989454));
#34252=DIRECTION('',(-1.,0.,0.));
#34253=DIRECTION('',(0.,-0.487029750822751,-0.87338537989454));
#34254=DIRECTION('center_axis',(-1.,0.,0.));
#34255=DIRECTION('ref_axis',(0.,0.642787609686539,-0.766044443118978));
#34256=DIRECTION('center_axis',(-1.,0.,0.));
#34257=DIRECTION('ref_axis',(0.,0.,-1.));
#34258=DIRECTION('center_axis',(0.,-0.487029750822751,0.87338537989454));
#34259=DIRECTION('ref_axis',(0.,0.87338537989454,0.487029750822751));
#34260=DIRECTION('',(1.,0.,0.));
#34261=DIRECTION('',(0.,0.87338537989454,0.487029750822751));
#34262=DIRECTION('',(-1.,0.,0.));
#34263=DIRECTION('center_axis',(0.,0.944688522187605,-0.327968894938222));
#34264=DIRECTION('ref_axis',(0.,-0.327968894938222,-0.944688522187605));
#34265=DIRECTION('',(-1.,0.,0.));
#34266=DIRECTION('',(0.,-0.327968894938222,-0.944688522187605));
#34267=DIRECTION('center_axis',(-1.,0.,0.));
#34268=DIRECTION('ref_axis',(0.,0.766044443118978,-0.642787609686539));
#34269=DIRECTION('center_axis',(-1.,0.,0.));
#34270=DIRECTION('ref_axis',(0.,0.,-1.));
#34271=DIRECTION('center_axis',(0.,-0.631292454177475,0.775544864787705));
#34272=DIRECTION('ref_axis',(0.,0.775544864787705,0.631292454177475));
#34273=DIRECTION('',(1.,0.,0.));
#34274=DIRECTION('',(0.,0.775544864787705,0.631292454177475));
#34275=DIRECTION('',(-1.,0.,0.));
#34276=DIRECTION('center_axis',(0.,0.987287781769458,-0.158942870141264));
#34277=DIRECTION('ref_axis',(0.,-0.158942870141264,-0.987287781769458));
#34278=DIRECTION('',(-1.,0.,0.));
#34279=DIRECTION('',(0.,-0.158942870141264,-0.987287781769458));
#34280=DIRECTION('center_axis',(-1.,0.,0.));
#34281=DIRECTION('ref_axis',(0.,0.866025403784439,-0.5));
#34282=DIRECTION('center_axis',(-1.,0.,0.));
#34283=DIRECTION('ref_axis',(0.,0.,-1.));
#34284=DIRECTION('center_axis',(0.,-0.756373655761413,0.654139811408934));
#34285=DIRECTION('ref_axis',(0.,0.654139811408934,0.756373655761413));
#34286=DIRECTION('',(1.,0.,0.));
#34287=DIRECTION('',(0.,0.654139811408934,0.756373655761413));
#34288=DIRECTION('',(-1.,0.,0.));
#34289=DIRECTION('center_axis',(0.,0.99988880169397,0.0149125533359626));
#34290=DIRECTION('ref_axis',(0.,0.0149125533359626,-0.99988880169397));
#34291=DIRECTION('',(-1.,0.,0.));
#34292=DIRECTION('',(0.,0.0149125533359626,-0.999888801693969));
#34293=DIRECTION('center_axis',(-1.,0.,0.));
#34294=DIRECTION('ref_axis',(0.,0.939692620785908,-0.342020143325669));
#34295=DIRECTION('center_axis',(-1.,0.,0.));
#34296=DIRECTION('ref_axis',(0.,0.,-1.));
#34297=DIRECTION('center_axis',(0.,-0.858472826558577,0.512859050871219));
#34298=DIRECTION('ref_axis',(0.,0.512859050871219,0.858472826558577));
#34299=DIRECTION('',(1.,0.,0.));
#34300=DIRECTION('',(0.,0.512859050871219,0.858472826558577));
#34301=DIRECTION('',(-1.,0.,0.));
#34302=DIRECTION('center_axis',(0.,0.982108706347157,0.188314866426193));
#34303=DIRECTION('ref_axis',(0.,0.188314866426193,-0.982108706347156));
#34304=DIRECTION('',(-1.,0.,0.));
#34305=DIRECTION('',(0.,0.188314866426193,-0.982108706347156));
#34306=DIRECTION('center_axis',(-1.,0.,0.));
#34307=DIRECTION('ref_axis',(0.,0.984807753012208,-0.17364817766693));
#34308=DIRECTION('center_axis',(-1.,0.,0.));
#34309=DIRECTION('ref_axis',(0.,0.,-1.));
#34310=DIRECTION('center_axis',(0.,-0.93448773492897,0.355995327591983));
#34311=DIRECTION('ref_axis',(0.,0.355995327591983,0.93448773492897));
#34312=DIRECTION('',(1.,0.,0.));
#34313=DIRECTION('',(0.,0.355995327591983,0.93448773492897));
#34314=DIRECTION('',(-1.,0.,0.));
#34315=DIRECTION('center_axis',(0.,0.93448773492897,0.355995327591983));
#34316=DIRECTION('ref_axis',(0.,0.355995327591983,-0.93448773492897));
#34317=DIRECTION('',(-1.,0.,0.));
#34318=DIRECTION('',(0.,0.355995327591983,-0.93448773492897));
#34319=DIRECTION('center_axis',(-1.,0.,0.));
#34320=DIRECTION('ref_axis',(0.,1.,6.12323399573677E-17));
#34321=DIRECTION('center_axis',(-1.,0.,0.));
#34322=DIRECTION('ref_axis',(0.,0.,-1.));
#34323=DIRECTION('center_axis',(0.,-0.982108706347157,0.188314866426192));
#34324=DIRECTION('ref_axis',(0.,0.188314866426192,0.982108706347157));
#34325=DIRECTION('',(1.,0.,0.));
#34326=DIRECTION('',(0.,0.188314866426192,0.982108706347157));
#34327=DIRECTION('',(-1.,0.,0.));
#34328=DIRECTION('center_axis',(0.,0.858472826558577,0.512859050871219));
#34329=DIRECTION('ref_axis',(0.,0.512859050871219,-0.858472826558577));
#34330=DIRECTION('',(-1.,0.,0.));
#34331=DIRECTION('',(0.,0.512859050871219,-0.858472826558577));
#34332=DIRECTION('center_axis',(-1.,0.,0.));
#34333=DIRECTION('ref_axis',(0.,0.984807753012208,0.17364817766693));
#34334=DIRECTION('center_axis',(-1.,0.,0.));
#34335=DIRECTION('ref_axis',(0.,0.,-1.));
#34336=DIRECTION('center_axis',(0.,-0.99988880169397,0.0149125533359625));
#34337=DIRECTION('ref_axis',(0.,0.0149125533359625,0.99988880169397));
#34338=DIRECTION('',(1.,0.,0.));
#34339=DIRECTION('',(0.,0.0149125533359625,0.99988880169397));
#34340=DIRECTION('',(-1.,0.,0.));
#34341=DIRECTION('center_axis',(0.,0.756373655761413,0.654139811408934));
#34342=DIRECTION('ref_axis',(0.,0.654139811408935,-0.756373655761413));
#34343=DIRECTION('',(-1.,0.,0.));
#34344=DIRECTION('',(0.,0.654139811408934,-0.756373655761413));
#34345=DIRECTION('center_axis',(-1.,0.,0.));
#34346=DIRECTION('ref_axis',(0.,0.939692620785908,0.342020143325669));
#34347=DIRECTION('center_axis',(-1.,0.,0.));
#34348=DIRECTION('ref_axis',(0.,0.,-1.));
#34349=DIRECTION('center_axis',(0.,-0.987287781769458,-0.158942870141265));
#34350=DIRECTION('ref_axis',(0.,-0.158942870141265,0.987287781769458));
#34351=DIRECTION('',(1.,0.,0.));
#34352=DIRECTION('',(0.,-0.158942870141265,0.987287781769458));
#34353=DIRECTION('',(-1.,0.,0.));
#34354=DIRECTION('center_axis',(0.,0.631292454177475,0.775544864787706));
#34355=DIRECTION('ref_axis',(0.,0.775544864787706,-0.631292454177475));
#34356=DIRECTION('',(-1.,0.,0.));
#34357=DIRECTION('',(0.,0.775544864787705,-0.631292454177475));
#34358=DIRECTION('center_axis',(-1.,0.,0.));
#34359=DIRECTION('ref_axis',(0.,0.866025403784439,0.5));
#34360=DIRECTION('center_axis',(-1.,0.,0.));
#34361=DIRECTION('ref_axis',(0.,0.,-1.));
#34362=DIRECTION('center_axis',(0.,-0.944688522187605,-0.327968894938222));
#34363=DIRECTION('ref_axis',(0.,-0.327968894938222,0.944688522187605));
#34364=DIRECTION('',(1.,0.,0.));
#34365=DIRECTION('',(0.,-0.327968894938222,0.944688522187605));
#34366=DIRECTION('',(-1.,0.,0.));
#34367=DIRECTION('center_axis',(0.,0.487029750822751,0.87338537989454));
#34368=DIRECTION('ref_axis',(0.,0.87338537989454,-0.487029750822751));
#34369=DIRECTION('',(-1.,0.,0.));
#34370=DIRECTION('',(0.,0.87338537989454,-0.487029750822751));
#34371=DIRECTION('center_axis',(-1.,0.,0.));
#34372=DIRECTION('ref_axis',(0.,0.766044443118978,0.642787609686539));
#34373=DIRECTION('center_axis',(-1.,0.,0.));
#34374=DIRECTION('ref_axis',(0.,0.,-1.));
#34375=DIRECTION('center_axis',(0.,-0.87338537989454,-0.487029750822751));
#34376=DIRECTION('ref_axis',(0.,-0.487029750822751,0.87338537989454));
#34377=DIRECTION('',(1.,0.,0.));
#34378=DIRECTION('',(0.,-0.487029750822751,0.87338537989454));
#34379=DIRECTION('',(-1.,0.,0.));
#34380=DIRECTION('center_axis',(0.,0.327968894938222,0.944688522187605));
#34381=DIRECTION('ref_axis',(0.,0.944688522187605,-0.327968894938222));
#34382=DIRECTION('',(-1.,0.,0.));
#34383=DIRECTION('',(0.,0.944688522187605,-0.327968894938222));
#34384=DIRECTION('center_axis',(-1.,0.,0.));
#34385=DIRECTION('ref_axis',(0.,0.642787609686539,0.766044443118978));
#34386=DIRECTION('center_axis',(-1.,0.,0.));
#34387=DIRECTION('ref_axis',(0.,0.,-1.));
#34388=DIRECTION('center_axis',(0.,-0.775544864787705,-0.631292454177475));
#34389=DIRECTION('ref_axis',(0.,-0.631292454177475,0.775544864787705));
#34390=DIRECTION('',(1.,0.,0.));
#34391=DIRECTION('',(0.,-0.631292454177475,0.775544864787705));
#34392=DIRECTION('',(-1.,0.,0.));
#34393=DIRECTION('center_axis',(0.,0.158942870141264,0.987287781769458));
#34394=DIRECTION('ref_axis',(0.,0.987287781769458,-0.158942870141264));
#34395=DIRECTION('',(-1.,0.,0.));
#34396=DIRECTION('',(0.,0.987287781769458,-0.158942870141264));
#34397=DIRECTION('center_axis',(-1.,0.,0.));
#34398=DIRECTION('ref_axis',(0.,0.5,0.866025403784439));
#34399=DIRECTION('center_axis',(-1.,0.,0.));
#34400=DIRECTION('ref_axis',(0.,0.,-1.));
#34401=DIRECTION('center_axis',(0.,-0.654139811408934,-0.756373655761413));
#34402=DIRECTION('ref_axis',(0.,-0.756373655761413,0.654139811408934));
#34403=DIRECTION('',(1.,0.,0.));
#34404=DIRECTION('',(0.,-0.756373655761413,0.654139811408934));
#34405=DIRECTION('',(-1.,0.,0.));
#34406=DIRECTION('center_axis',(0.,-0.0149125533359626,0.99988880169397));
#34407=DIRECTION('ref_axis',(0.,0.99988880169397,0.0149125533359626));
#34408=DIRECTION('',(-1.,0.,0.));
#34409=DIRECTION('',(0.,0.999888801693969,0.0149125533359626));
#34410=DIRECTION('center_axis',(-1.,0.,0.));
#34411=DIRECTION('ref_axis',(0.,0.342020143325669,0.939692620785908));
#34412=DIRECTION('center_axis',(-1.,0.,0.));
#34413=DIRECTION('ref_axis',(0.,0.,-1.));
#34414=DIRECTION('center_axis',(0.,-0.512859050871219,-0.858472826558577));
#34415=DIRECTION('ref_axis',(0.,-0.858472826558577,0.512859050871219));
#34416=DIRECTION('',(1.,0.,0.));
#34417=DIRECTION('',(0.,-0.858472826558577,0.512859050871219));
#34418=DIRECTION('',(-1.,0.,0.));
#34419=DIRECTION('center_axis',(0.,-0.188314866426193,0.982108706347157));
#34420=DIRECTION('ref_axis',(0.,0.982108706347156,0.188314866426193));
#34421=DIRECTION('',(-1.,0.,0.));
#34422=DIRECTION('',(0.,0.982108706347156,0.188314866426193));
#34423=DIRECTION('center_axis',(-1.,0.,0.));
#34424=DIRECTION('ref_axis',(0.,0.17364817766693,0.984807753012208));
#34425=DIRECTION('center_axis',(-1.,0.,0.));
#34426=DIRECTION('ref_axis',(0.,0.,-1.));
#34427=DIRECTION('center_axis',(0.,-0.355995327591983,-0.93448773492897));
#34428=DIRECTION('ref_axis',(0.,-0.93448773492897,0.355995327591983));
#34429=DIRECTION('',(1.,0.,0.));
#34430=DIRECTION('',(0.,-0.93448773492897,0.355995327591983));
#34431=DIRECTION('',(-1.,0.,0.));
#34432=DIRECTION('center_axis',(0.,-0.355995327591983,0.93448773492897));
#34433=DIRECTION('ref_axis',(0.,0.93448773492897,0.355995327591983));
#34434=DIRECTION('',(-1.,0.,0.));
#34435=DIRECTION('',(0.,0.93448773492897,0.355995327591983));
#34436=DIRECTION('center_axis',(-1.,0.,0.));
#34437=DIRECTION('ref_axis',(0.,0.,1.));
#34438=DIRECTION('center_axis',(-1.,0.,0.));
#34439=DIRECTION('ref_axis',(0.,0.,-1.));
#34440=DIRECTION('center_axis',(1.,0.,0.));
#34441=DIRECTION('ref_axis',(0.,0.,-1.));
#34442=DIRECTION('',(-1.,0.,0.));
#34443=DIRECTION('center_axis',(1.,0.,0.));
#34444=DIRECTION('ref_axis',(0.,0.,-1.));
#34445=DIRECTION('',(0.,0.499999999999998,-0.86602540378444));
#34446=DIRECTION('',(0.,-0.499999999999999,-0.866025403784439));
#34447=DIRECTION('',(0.,-1.,0.));
#34448=DIRECTION('',(0.,-0.500000000000003,0.866025403784437));
#34449=DIRECTION('',(0.,0.500000000000002,0.866025403784437));
#34450=DIRECTION('',(0.,1.,0.));
#34451=DIRECTION('center_axis',(1.,0.,0.));
#34452=DIRECTION('ref_axis',(0.,0.,-1.));
#34453=DIRECTION('',(0.,0.499999999999998,-0.86602540378444));
#34454=DIRECTION('center_axis',(1.,0.,0.));
#34455=DIRECTION('ref_axis',(0.,0.,-1.));
#34456=DIRECTION('center_axis',(1.,0.,0.));
#34457=DIRECTION('ref_axis',(0.,0.,-1.));
#34458=DIRECTION('',(0.,-0.499999999999999,-0.866025403784439));
#34459=DIRECTION('center_axis',(1.,0.,0.));
#34460=DIRECTION('ref_axis',(0.,0.,-1.));
#34461=DIRECTION('center_axis',(1.,0.,0.));
#34462=DIRECTION('ref_axis',(0.,0.,-1.));
#34463=DIRECTION('',(0.,-1.,0.));
#34464=DIRECTION('center_axis',(1.,0.,0.));
#34465=DIRECTION('ref_axis',(0.,0.,-1.));
#34466=DIRECTION('center_axis',(1.,0.,0.));
#34467=DIRECTION('ref_axis',(0.,0.,-1.));
#34468=DIRECTION('',(0.,-0.500000000000003,0.866025403784437));
#34469=DIRECTION('center_axis',(1.,0.,0.));
#34470=DIRECTION('ref_axis',(0.,0.,-1.));
#34471=DIRECTION('center_axis',(1.,0.,0.));
#34472=DIRECTION('ref_axis',(0.,0.,-1.));
#34473=DIRECTION('',(0.,0.500000000000002,0.866025403784437));
#34474=DIRECTION('center_axis',(1.,0.,0.));
#34475=DIRECTION('ref_axis',(0.,0.,-1.));
#34476=DIRECTION('center_axis',(1.,0.,0.));
#34477=DIRECTION('ref_axis',(0.,0.,-1.));
#34478=DIRECTION('',(0.,1.,0.));
#34479=DIRECTION('center_axis',(1.,0.,0.));
#34480=DIRECTION('ref_axis',(0.,0.,-1.));
#34481=DIRECTION('center_axis',(1.,0.,0.));
#34482=DIRECTION('ref_axis',(0.,1.,0.));
#34483=DIRECTION('',(0.515038074910058,-0.85716730070211,-1.04972719113862E-16));
#34484=DIRECTION('center_axis',(0.,0.86602540378444,0.499999999999998));
#34485=DIRECTION('ref_axis',(0.,0.499999999999998,-0.86602540378444));
#34486=DIRECTION('',(-1.,0.,0.));
#34487=DIRECTION('',(-1.,0.,0.));
#34488=DIRECTION('center_axis',(0.,0.,1.));
#34489=DIRECTION('ref_axis',(0.,1.,0.));
#34490=DIRECTION('',(-1.,0.,0.));
#34491=DIRECTION('center_axis',(0.,-0.866025403784437,0.500000000000002));
#34492=DIRECTION('ref_axis',(0.,0.500000000000002,0.866025403784437));
#34493=DIRECTION('',(-1.,0.,0.));
#34494=DIRECTION('center_axis',(0.,-0.866025403784437,-0.500000000000003));
#34495=DIRECTION('ref_axis',(0.,-0.500000000000003,0.866025403784437));
#34496=DIRECTION('',(-1.,0.,0.));
#34497=DIRECTION('center_axis',(0.,0.,-1.));
#34498=DIRECTION('ref_axis',(0.,-1.,0.));
#34499=DIRECTION('',(-1.,0.,0.));
#34500=DIRECTION('center_axis',(0.,0.866025403784439,-0.499999999999999));
#34501=DIRECTION('ref_axis',(0.,-0.499999999999999,-0.866025403784439));
#53157=CARTESIAN_POINT('',(0.,0.,0.));
#53158=CARTESIAN_POINT('Origin',(21.26284859951,71.6454,13.47));
#53159=CARTESIAN_POINT('',(19.2164763792089,70.6843589395965,14.3002409771978));
#53160=CARTESIAN_POINT('',(19.3867992156006,70.6843590974191,14.3002411598846));
#53161=CARTESIAN_POINT('',(21.26284859951,70.6843589433668,14.3002409815622));
#53162=CARTESIAN_POINT('',(19.789,72.647668068024,14.249973537897));
#53163=CARTESIAN_POINT('Ctrl Pts',(19.2164763792089,70.6843589395965,14.3002409771978));
#53164=CARTESIAN_POINT('Ctrl Pts',(19.2168429075804,70.681863837098,14.2973527844721));
#53165=CARTESIAN_POINT('Ctrl Pts',(19.2172098790625,70.679381571615,14.2944531325613));
#53166=CARTESIAN_POINT('Ctrl Pts',(19.2203735586003,70.6581199751139,14.2693885665096));
#53167=CARTESIAN_POINT('Ctrl Pts',(19.2231939759151,70.6400952029175,14.2465989227062));
#53168=CARTESIAN_POINT('Ctrl Pts',(19.2283298761436,70.6090614176701,14.2044687577327));
#53169=CARTESIAN_POINT('Ctrl Pts',(19.2306334126591,70.5957730093062,14.1853495767784));
#53170=CARTESIAN_POINT('Ctrl Pts',(19.2358933228042,70.566899472208,14.1412689611443));
#53171=CARTESIAN_POINT('Ctrl Pts',(19.2388601162184,70.5516421023775,14.1161104475929));
#53172=CARTESIAN_POINT('Ctrl Pts',(19.245306516531,70.5207313108932,14.0609034025463));
#53173=CARTESIAN_POINT('Ctrl Pts',(19.248793395299,70.5053792974457,14.0307127787972));
#53174=CARTESIAN_POINT('Ctrl Pts',(19.260638083729,70.4577964388134,13.9270844769763));
#53175=CARTESIAN_POINT('Ctrl Pts',(19.2691208238696,70.4313164707027,13.851218962717));
#53176=CARTESIAN_POINT('Ctrl Pts',(19.2811264822653,70.403892231256,13.7397374214405));
#53177=CARTESIAN_POINT('Ctrl Pts',(19.2847231573083,70.3969964706005,13.7057732353553));
#53178=CARTESIAN_POINT('Ctrl Pts',(19.2899042395514,70.3889490281663,13.6557116143545));
#53179=CARTESIAN_POINT('Ctrl Pts',(19.2915324535741,70.3867011485181,13.6398091350018));
#53180=CARTESIAN_POINT('Ctrl Pts',(19.2945437089717,70.3830668610433,13.6100331070147));
#53181=CARTESIAN_POINT('Ctrl Pts',(19.295929794351,70.3816062560078,13.596173036667));
#53182=CARTESIAN_POINT('Ctrl Pts',(19.2997078124637,70.3782205834204,13.558030982768));
#53183=CARTESIAN_POINT('Ctrl Pts',(19.3020765616023,70.3767652524541,13.5337124428857));
#53184=CARTESIAN_POINT('Ctrl Pts',(19.3112196809774,70.3738224559109,13.4388155969604));
#53185=CARTESIAN_POINT('Ctrl Pts',(19.3178124549841,70.3775195642012,13.3681986156259));
#53186=CARTESIAN_POINT('Ctrl Pts',(19.3303011348092,70.3954907639043,13.2365338949063));
#53187=CARTESIAN_POINT('Ctrl Pts',(19.336170246313,70.4084416179811,13.1755310944575));
#53188=CARTESIAN_POINT('Ctrl Pts',(19.3449414390738,70.4338472116275,13.0880715213876));
#53189=CARTESIAN_POINT('Ctrl Pts',(19.3477390753848,70.4428192040899,13.0606973585204));
#53190=CARTESIAN_POINT('Ctrl Pts',(19.3528559857273,70.4607239213449,13.0117574570982));
#53191=CARTESIAN_POINT('Ctrl Pts',(19.3551639014561,70.4693356376713,12.9900874270695));
#53192=CARTESIAN_POINT('Ctrl Pts',(19.3604659406686,70.4902952193295,12.9413034783983));
#53193=CARTESIAN_POINT('Ctrl Pts',(19.3634711651694,70.5030099694296,12.9143636854465));
#53194=CARTESIAN_POINT('Ctrl Pts',(19.3700228310512,70.5324665265379,12.8572450724786));
#53195=CARTESIAN_POINT('Ctrl Pts',(19.3735771176978,70.5495150216147,12.8272518836919));
#53196=CARTESIAN_POINT('Ctrl Pts',(19.3859489294713,70.6124930226616,12.7262596317474));
#53197=CARTESIAN_POINT('Ctrl Pts',(19.3949053466999,70.6642753087591,12.6591736926245));
#53198=CARTESIAN_POINT('Ctrl Pts',(19.4070481448538,70.7442249556762,12.574567306746));
#53199=CARTESIAN_POINT('Ctrl Pts',(19.4103473619394,70.7669863786179,12.5522276023595));
#53200=CARTESIAN_POINT('Ctrl Pts',(19.4151268096689,70.8016787093509,12.5206527915009));
#53201=CARTESIAN_POINT('Ctrl Pts',(19.4166459995177,70.8129697896658,12.5107368649377));
#53202=CARTESIAN_POINT('Ctrl Pts',(19.4195932073838,70.8354252412169,12.4917115085214));
#53203=CARTESIAN_POINT('Ctrl Pts',(19.4210218878832,70.8465736314974,12.4825872339658));
#53204=CARTESIAN_POINT('Ctrl Pts',(19.4251914134929,70.8798241201264,12.45630563044));
#53205=CARTESIAN_POINT('Ctrl Pts',(19.4278994890532,70.902342629105,12.4396850803356));
#53206=CARTESIAN_POINT('Ctrl Pts',(19.4347054728509,70.9608637271432,12.3994094951654));
#53207=CARTESIAN_POINT('Ctrl Pts',(19.4387619929617,70.9975545483525,12.3768161769161));
#53208=CARTESIAN_POINT('Ctrl Pts',(19.4508471703472,71.110373258616,12.315024619423));
#53209=CARTESIAN_POINT('Ctrl Pts',(19.4588265941442,71.1893737152542,12.2816148369606));
#53210=CARTESIAN_POINT('Ctrl Pts',(19.4698025389508,71.2982724301739,12.2480305189914));
#53211=CARTESIAN_POINT('Ctrl Pts',(19.4725621440301,71.3256885414681,12.2405727938614));
#53212=CARTESIAN_POINT('Ctrl Pts',(19.4776248489093,71.3758648007065,12.2287155892559));
#53213=CARTESIAN_POINT('Ctrl Pts',(19.4799170825887,71.3985398628625,12.2240079817857));
#53214=CARTESIAN_POINT('Ctrl Pts',(19.4851976209107,71.4505879456488,12.2146785881989));
#53215=CARTESIAN_POINT('Ctrl Pts',(19.4881972703673,71.4800185947512,12.2104634964333));
#53216=CARTESIAN_POINT('Ctrl Pts',(19.4947439182504,71.5438588165329,12.2035960665193));
#53217=CARTESIAN_POINT('Ctrl Pts',(19.4982989405825,71.5782828528241,12.2013060533782));
#53218=CARTESIAN_POINT('Ctrl Pts',(19.5107312255758,71.6978178066059,12.1982323250094));
#53219=CARTESIAN_POINT('Ctrl Pts',(19.5197495849094,71.7828786800747,12.2045994047425));
#53220=CARTESIAN_POINT('Ctrl Pts',(19.5318875764421,71.8974776408687,12.2248749813478));
#53221=CARTESIAN_POINT('Ctrl Pts',(19.5351259120864,71.9280869601518,12.2314653790781));
#53222=CARTESIAN_POINT('Ctrl Pts',(19.5398337800826,71.9728712918292,12.2428550418573));
#53223=CARTESIAN_POINT('Ctrl Pts',(19.5413409228134,71.9872531055494,12.2467834505386));
#53224=CARTESIAN_POINT('Ctrl Pts',(19.5442942608923,72.015562915247,12.2550546821376));
#53225=CARTESIAN_POINT('Ctrl Pts',(19.5457407640702,72.0294918319582,12.259386005918));
#53226=CARTESIAN_POINT('Ctrl Pts',(19.5499984136167,72.0705925315987,12.2729475282185));
#53227=CARTESIAN_POINT('Ctrl Pts',(19.5527751996227,72.0975318150761,12.2828603534509));
#53228=CARTESIAN_POINT('Ctrl Pts',(19.5598205255003,72.1656581354462,12.3105850170304));
#53229=CARTESIAN_POINT('Ctrl Pts',(19.5640444489924,72.2062799415021,12.3296816135803));
#53230=CARTESIAN_POINT('Ctrl Pts',(19.5759528630704,72.3179256393901,12.3895801636631));
#53231=CARTESIAN_POINT('Ctrl Pts',(19.5836016786601,72.3861247366692,12.4351462409573));
#53232=CARTESIAN_POINT('Ctrl Pts',(19.5942649102365,72.4718197969328,12.5052385828239));
#53233=CARTESIAN_POINT('Ctrl Pts',(19.5970708789752,72.4935448817875,12.5242811033578));
#53234=CARTESIAN_POINT('Ctrl Pts',(19.6022046167316,72.5316602332081,12.5600602738273));
#53235=CARTESIAN_POINT('Ctrl Pts',(19.604521012432,72.5482729755313,12.5765417091077));
#53236=CARTESIAN_POINT('Ctrl Pts',(19.6098466804553,72.585077824801,12.6151307265006));
#53237=CARTESIAN_POINT('Ctrl Pts',(19.612867158386,72.6049614312251,12.637511336186));
#53238=CARTESIAN_POINT('Ctrl Pts',(19.6194588098718,72.6461681550016,12.6873320196457));
#53239=CARTESIAN_POINT('Ctrl Pts',(19.623037963183,72.6671927970557,12.7149867203004));
#53240=CARTESIAN_POINT('Ctrl Pts',(19.6356191537873,72.7364351073826,12.8142616228827));
#53241=CARTESIAN_POINT('Ctrl Pts',(19.6447635263264,72.7784644025375,12.8899017016047));
#53242=CARTESIAN_POINT('Ctrl Pts',(19.6568859224128,72.8243704710686,12.9968876180625));
#53243=CARTESIAN_POINT('Ctrl Pts',(19.6599963790701,72.8352575146703,13.02497615349));
#53244=CARTESIAN_POINT('Ctrl Pts',(19.6645720017463,72.8500065262947,13.0674536794229));
#53245=CARTESIAN_POINT('Ctrl Pts',(19.6660713638686,72.8546305486713,13.0815646861551));
#53246=CARTESIAN_POINT('Ctrl Pts',(19.6690754581906,72.8634810902459,13.1102653333141));
#53247=CARTESIAN_POINT('Ctrl Pts',(19.6705794803392,72.8676955066706,13.1248560476031));
#53248=CARTESIAN_POINT('Ctrl Pts',(19.6752168388686,72.8799792249048,13.170434856023));
#53249=CARTESIAN_POINT('Ctrl Pts',(19.6783069432916,72.8871399328896,13.2016576698065));
#53250=CARTESIAN_POINT('Ctrl Pts',(19.686625634525,72.9033779104689,13.2871882636698));
#53251=CARTESIAN_POINT('Ctrl Pts',(19.6917879714546,72.9101180824344,13.3418687883531));
#53252=CARTESIAN_POINT('Ctrl Pts',(19.7029309147804,72.9169394823104,13.4600500361316));
#53253=CARTESIAN_POINT('Ctrl Pts',(19.7089034057813,72.9158535470839,13.5234594134692));
#53254=CARTESIAN_POINT('Ctrl Pts',(19.7177908111219,72.9073934457991,13.615282351177));
#53255=CARTESIAN_POINT('Ctrl Pts',(19.7205984160596,72.9037628881701,13.6439452880197));
#53256=CARTESIAN_POINT('Ctrl Pts',(19.725726796497,72.8954411422604,13.6954794733644));
#53257=CARTESIAN_POINT('Ctrl Pts',(19.7280361519483,72.8910903866998,13.718393105371));
#53258=CARTESIAN_POINT('Ctrl Pts',(19.7333880858738,72.8796506962368,13.7707338614926));
#53259=CARTESIAN_POINT('Ctrl Pts',(19.73644264786,72.8721359288739,13.8000518319183));
#53260=CARTESIAN_POINT('Ctrl Pts',(19.7474350955257,72.8416656876718,13.9034251323406));
#53261=CARTESIAN_POINT('Ctrl Pts',(19.7555375219246,72.8129916041973,13.9756029856989));
#53262=CARTESIAN_POINT('Ctrl Pts',(19.7703697319023,72.7491901579731,14.1013317241615));
#53263=CARTESIAN_POINT('Ctrl Pts',(19.7770595157045,72.7162445241044,14.1557303774103));
#53264=CARTESIAN_POINT('Ctrl Pts',(19.7849207425938,72.6718520992,14.2179728876546));
#53265=CARTESIAN_POINT('Ctrl Pts',(19.7862437452096,72.6641794033323,14.2283903497352));
#53266=CARTESIAN_POINT('Ctrl Pts',(19.788039790452,72.6534761011556,14.2424668884386));
#53267=CARTESIAN_POINT('Ctrl Pts',(19.7885205481825,72.6505826200053,14.2462283308591));
#53268=CARTESIAN_POINT('Ctrl Pts',(19.789,72.647668068024,14.249973537897));
#53269=CARTESIAN_POINT('',(19.789,72.6399444526778,12.6802017145829));
#53270=CARTESIAN_POINT('Origin',(19.789,71.6454,13.47));
#53271=CARTESIAN_POINT('Ctrl Pts',(19.789,72.6399444526778,12.6802017145829));
#53272=CARTESIAN_POINT('Ctrl Pts',(19.7879988394882,72.6336852930391,12.672319939436));
#53273=CARTESIAN_POINT('Ctrl Pts',(19.7870028556559,72.6273323603128,12.6645124714419));
#53274=CARTESIAN_POINT('Ctrl Pts',(19.7847784439559,72.6128720806095,12.6471668188866));
#53275=CARTESIAN_POINT('Ctrl Pts',(19.7835526048889,72.6047150907637,12.6376711834672));
#53276=CARTESIAN_POINT('Ctrl Pts',(19.7773813155715,72.5627506193215,12.5902565904165));
#53277=CARTESIAN_POINT('Ctrl Pts',(19.7725303707011,72.5268266800043,12.5542659926393));
#53278=CARTESIAN_POINT('Ctrl Pts',(19.7617685551579,72.4422971478315,12.4791768851631));
#53279=CARTESIAN_POINT('Ctrl Pts',(19.7558780378122,72.3927802509567,12.4413126180756));
#53280=CARTESIAN_POINT('Ctrl Pts',(19.7462334159638,72.3087868944108,12.3863620821621));
#53281=CARTESIAN_POINT('Ctrl Pts',(19.7425421902648,72.2759649348693,12.3669403329942));
#53282=CARTESIAN_POINT('Ctrl Pts',(19.736254889877,72.2193745096782,12.3368057594637));
#53283=CARTESIAN_POINT('Ctrl Pts',(19.7336854247468,72.1960588739323,12.3252945758548));
#53284=CARTESIAN_POINT('Ctrl Pts',(19.7281348856773,72.1454268695547,12.3022018303799));
#53285=CARTESIAN_POINT('Ctrl Pts',(19.7251484813524,72.1180255286648,12.2908459830346));
#53286=CARTESIAN_POINT('Ctrl Pts',(19.7140452233699,72.0157999892946,12.2526164872599));
#53287=CARTESIAN_POINT('Ctrl Pts',(19.7057531723403,71.9389123233391,12.2318303828563));
#53288=CARTESIAN_POINT('Ctrl Pts',(19.6913527117728,71.8044342218704,12.2087084287361));
#53289=CARTESIAN_POINT('Ctrl Pts',(19.6853095854195,71.7476766647075,12.2028424775483));
#53290=CARTESIAN_POINT('Ctrl Pts',(19.6768504473155,71.6669693918566,12.1999608821039));
#53291=CARTESIAN_POINT('Ctrl Pts',(19.6743762563562,71.6432020505806,12.1997795629759));
#53292=CARTESIAN_POINT('Ctrl Pts',(19.669947988605,71.6002578236911,12.200657509051));
#53293=CARTESIAN_POINT('Ctrl Pts',(19.6679860457168,71.5810833269988,12.2014844546591));
#53294=CARTESIAN_POINT('Ctrl Pts',(19.6647026309535,71.5486777115068,12.2036188307956));
#53295=CARTESIAN_POINT('Ctrl Pts',(19.6633704522261,71.5354361464308,12.2046998399272));
#53296=CARTESIAN_POINT('Ctrl Pts',(19.6602845196912,71.5045364833099,12.2077112635583));
#53297=CARTESIAN_POINT('Ctrl Pts',(19.6585393557641,71.4868974890424,12.2098045934731));
#53298=CARTESIAN_POINT('Ctrl Pts',(19.6498582440392,71.3986097154966,12.2221656500283));
#53299=CARTESIAN_POINT('Ctrl Pts',(19.6431693056601,71.3288603498329,12.2380088120933));
#53300=CARTESIAN_POINT('Ctrl Pts',(19.6293829670148,71.1888474772813,12.2824984306449));
#53301=CARTESIAN_POINT('Ctrl Pts',(19.6223084569495,71.1190850290944,12.311729570797));
#53302=CARTESIAN_POINT('Ctrl Pts',(19.6124496507591,71.0286864704104,12.3594687047662));
#53303=CARTESIAN_POINT('Ctrl Pts',(19.6098485541804,71.0054387019098,12.3727012160118));
#53304=CARTESIAN_POINT('Ctrl Pts',(19.6050255725437,70.9635718536933,12.3983146807423));
#53305=CARTESIAN_POINT('Ctrl Pts',(19.6028126646699,70.9448283893441,12.410472605138));
#53306=CARTESIAN_POINT('Ctrl Pts',(19.5977221940172,70.9028369999673,12.4393116639029));
#53307=CARTESIAN_POINT('Ctrl Pts',(19.5948337905242,70.8798137824313,12.4562960714327));
#53308=CARTESIAN_POINT('Ctrl Pts',(19.5841226200794,70.797485542498,12.5214351470659));
#53309=CARTESIAN_POINT('Ctrl Pts',(19.5761269612599,70.7419955868275,12.5741261346011));
#53310=CARTESIAN_POINT('Ctrl Pts',(19.5627784869408,70.6585251082356,12.669072493034));
#53311=CARTESIAN_POINT('Ctrl Pts',(19.5574781612633,70.6277176693713,12.7085999416123));
#53312=CARTESIAN_POINT('Ctrl Pts',(19.5499662115609,70.5869744350306,12.7677823866825));
#53313=CARTESIAN_POINT('Ctrl Pts',(19.5477032092482,70.5750879154414,12.7860362186686));
#53314=CARTESIAN_POINT('Ctrl Pts',(19.5436336555357,70.5543660060603,12.819722713213));
#53315=CARTESIAN_POINT('Ctrl Pts',(19.5418202203562,70.5453738894984,12.8350524380318));
#53316=CARTESIAN_POINT('Ctrl Pts',(19.5387084575586,70.5303372145233,12.8619658983364));
#53317=CARTESIAN_POINT('Ctrl Pts',(19.5374020074727,70.5241452364414,12.8734614197647));
#53318=CARTESIAN_POINT('Ctrl Pts',(19.5342433060912,70.5094867933954,12.9017101196916));
#53319=CARTESIAN_POINT('Ctrl Pts',(19.532402211052,70.5012123517248,12.9185591906536));
#53320=CARTESIAN_POINT('Ctrl Pts',(19.5245275905332,70.4671254145594,12.9920437533232));
#53321=CARTESIAN_POINT('Ctrl Pts',(19.5186670208826,70.445118143105,13.0503583479718));
#53322=CARTESIAN_POINT('Ctrl Pts',(19.505389113183,70.4050624171872,13.1858947310944));
#53323=CARTESIAN_POINT('Ctrl Pts',(19.4980018544375,70.389784631206,13.263647936012));
#53324=CARTESIAN_POINT('Ctrl Pts',(19.4875001249208,70.3787966095861,13.3723817903781));
#53325=CARTESIAN_POINT('Ctrl Pts',(19.4845703988531,70.376832553647,13.4025480942954));
#53326=CARTESIAN_POINT('Ctrl Pts',(19.4793007955481,70.3752560384368,13.4562790365754));
#53327=CARTESIAN_POINT('Ctrl Pts',(19.4769748788724,70.3752199411901,13.4798176295983));
#53328=CARTESIAN_POINT('Ctrl Pts',(19.4717346745804,70.3765998513407,13.5323607598734));
#53329=CARTESIAN_POINT('Ctrl Pts',(19.4688113226574,70.3783565953324,13.5613419568591));
#53330=CARTESIAN_POINT('Ctrl Pts',(19.4591533400977,70.3873460382674,13.6558680040669));
#53331=CARTESIAN_POINT('Ctrl Pts',(19.4523070297242,70.3986879227047,13.7209038937591));
#53332=CARTESIAN_POINT('Ctrl Pts',(19.4398511109362,70.4281474718696,13.836061332478));
#53333=CARTESIAN_POINT('Ctrl Pts',(19.4342764055587,70.4444692454006,13.8864975665481));
#53334=CARTESIAN_POINT('Ctrl Pts',(19.4254955442047,70.4754023224365,13.9649649865178));
#53335=CARTESIAN_POINT('Ctrl Pts',(19.4222532025384,70.4879916706145,13.9937282944117));
#53336=CARTESIAN_POINT('Ctrl Pts',(19.4175229582569,70.5081964536159,14.0355934572513));
#53337=CARTESIAN_POINT('Ctrl Pts',(19.4159984281185,70.514999931154,14.0490713494076));
#53338=CARTESIAN_POINT('Ctrl Pts',(19.4129954177348,70.5290043609389,14.0756265349366));
#53339=CARTESIAN_POINT('Ctrl Pts',(19.4115170092043,70.5361986872056,14.0887044839687));
#53340=CARTESIAN_POINT('Ctrl Pts',(19.4071386715044,70.5583618679716,14.1273631674709));
#53341=CARTESIAN_POINT('Ctrl Pts',(19.4042749414895,70.5739985221918,14.1525522286725));
#53342=CARTESIAN_POINT('Ctrl Pts',(19.3964964233314,70.6192749395329,14.2200913337217));
#53343=CARTESIAN_POINT('Ctrl Pts',(19.3916486420623,70.6506210044543,14.2611878234796));
#53344=CARTESIAN_POINT('Ctrl Pts',(19.3867992156006,70.6843590974191,14.3002411598846));
#53345=CARTESIAN_POINT('Origin',(21.26284859951,71.6454,13.47));
#53346=CARTESIAN_POINT('',(18.4247393426037,70.684358943376,14.3002409815728));
#53347=CARTESIAN_POINT('',(18.5941331801233,70.6843589436049,14.3002409818378));
#53348=CARTESIAN_POINT('',(21.26284859951,70.6843589433668,14.3002409815622));
#53349=CARTESIAN_POINT('Ctrl Pts',(18.4247393426037,70.684358943376,14.3002409815728));
#53350=CARTESIAN_POINT('Ctrl Pts',(18.425741837683,70.677743151105,14.2925829062241));
#53351=CARTESIAN_POINT('Ctrl Pts',(18.426738253587,70.6712186152227,14.2848454309185));
#53352=CARTESIAN_POINT('Ctrl Pts',(18.4310008909796,70.6435570992383,14.251234236303));
#53353=CARTESIAN_POINT('Ctrl Pts',(18.4342130005463,70.62335075497,14.2246072170568));
#53354=CARTESIAN_POINT('Ctrl Pts',(18.4451512763027,70.557562841565,14.1304153569593));
#53355=CARTESIAN_POINT('Ctrl Pts',(18.4527090504329,70.5174438461248,14.0592829745899));
#53356=CARTESIAN_POINT('Ctrl Pts',(18.4636331169903,70.4706142053097,13.9536708102035));
#53357=CARTESIAN_POINT('Ctrl Pts',(18.4668715850954,70.4580719728617,13.9220076591756));
#53358=CARTESIAN_POINT('Ctrl Pts',(18.4729847990637,70.4370577292689,13.8620209287228));
#53359=CARTESIAN_POINT('Ctrl Pts',(18.4758486955719,70.428273161499,13.8338315433662));
#53360=CARTESIAN_POINT('Ctrl Pts',(18.4810269221752,70.4143335579837,13.7829170210937));
#53361=CARTESIAN_POINT('Ctrl Pts',(18.483328303393,70.4088065798096,13.7603070505413));
#53362=CARTESIAN_POINT('Ctrl Pts',(18.4885356144993,70.3978094517496,13.709279624219));
#53363=CARTESIAN_POINT('Ctrl Pts',(18.491450989609,70.3926834048692,13.680802528491));
#53364=CARTESIAN_POINT('Ctrl Pts',(18.5024808275012,70.3771409462211,13.5735734785334));
#53365=CARTESIAN_POINT('Ctrl Pts',(18.5107762815057,70.3731487127085,13.4940889856527));
#53366=CARTESIAN_POINT('Ctrl Pts',(18.5239525363185,70.3785970503642,13.3689271249055));
#53367=CARTESIAN_POINT('Ctrl Pts',(18.5287838083082,70.3830755652537,13.3232250803623));
#53368=CARTESIAN_POINT('Ctrl Pts',(18.5365832358525,70.394411456068,13.2491585425132));
#53369=CARTESIAN_POINT('Ctrl Pts',(18.5395816522431,70.3997885703953,13.2206090407001));
#53370=CARTESIAN_POINT('Ctrl Pts',(18.5440235569083,70.4093357795369,13.1780090611116));
#53371=CARTESIAN_POINT('Ctrl Pts',(18.5454989030837,70.4127770063366,13.1638070835307));
#53372=CARTESIAN_POINT('Ctrl Pts',(18.5484508306831,70.4202214396926,13.1352470496773));
#53373=CARTESIAN_POINT('Ctrl Pts',(18.5499267264548,70.4242337721853,13.1208937637423));
#53374=CARTESIAN_POINT('Ctrl Pts',(18.5544368803024,70.4373710838782,13.0768998218101));
#53375=CARTESIAN_POINT('Ctrl Pts',(18.5574299679871,70.447330451625,13.0475174934628));
#53376=CARTESIAN_POINT('Ctrl Pts',(18.5672561716199,70.4838962940663,12.9513764204617));
#53377=CARTESIAN_POINT('Ctrl Pts',(18.5739450902649,70.5150891527752,12.8865102397918));
#53378=CARTESIAN_POINT('Ctrl Pts',(18.584531299636,70.5722362610615,12.7896557921468));
#53379=CARTESIAN_POINT('Ctrl Pts',(18.5883696803837,70.5945332513164,12.755698062384));
#53380=CARTESIAN_POINT('Ctrl Pts',(18.5954163945729,70.6378460445888,12.6961616468645));
#53381=CARTESIAN_POINT('Ctrl Pts',(18.5986057031769,70.6583077968545,12.6702254514615));
#53382=CARTESIAN_POINT('Ctrl Pts',(18.6041314029079,70.6950198077227,12.6272486530822));
#53383=CARTESIAN_POINT('Ctrl Pts',(18.606447414308,70.7107764233039,12.609807618483));
#53384=CARTESIAN_POINT('Ctrl Pts',(18.6114353914224,70.7454265991816,12.5735296411886));
#53385=CARTESIAN_POINT('Ctrl Pts',(18.614111999859,70.7644477113742,12.5548311508484));
#53386=CARTESIAN_POINT('Ctrl Pts',(18.6230514054813,70.8292754194238,12.4949975469171));
#53387=CARTESIAN_POINT('Ctrl Pts',(18.629417008987,70.8774760617912,12.4566001537864));
#53388=CARTESIAN_POINT('Ctrl Pts',(18.642452446823,70.9802527148792,12.3862806296208));
#53389=CARTESIAN_POINT('Ctrl Pts',(18.6491085557561,71.0348184245439,12.3546262370709));
#53390=CARTESIAN_POINT('Ctrl Pts',(18.6582392870559,71.1134623988977,12.3165106668744));
#53391=CARTESIAN_POINT('Ctrl Pts',(18.6607746650606,71.1357213872924,12.3065039086482));
#53392=CARTESIAN_POINT('Ctrl Pts',(18.6652822071527,71.1761733835701,12.2897022520299));
#53393=CARTESIAN_POINT('Ctrl Pts',(18.6672627623462,71.1942601728435,12.2826713192427));
#53394=CARTESIAN_POINT('Ctrl Pts',(18.6705766991242,71.225123269539,12.271481044188));
#53395=CARTESIAN_POINT('Ctrl Pts',(18.6719206729941,71.2378157227746,12.2671054329145));
#53396=CARTESIAN_POINT('Ctrl Pts',(18.6751100446828,71.268354504273,12.2571164384364));
#53397=CARTESIAN_POINT('Ctrl Pts',(18.6769452671747,71.2862597317993,12.2516945187455));
#53398=CARTESIAN_POINT('Ctrl Pts',(18.6852311740424,71.3683470179891,12.2288048565841));
#53399=CARTESIAN_POINT('Ctrl Pts',(18.6914817290103,71.4337293142145,12.2159975481437));
#53400=CARTESIAN_POINT('Ctrl Pts',(18.7028746761604,71.5542198965642,12.202094430482));
#53401=CARTESIAN_POINT('Ctrl Pts',(18.7080048237426,71.6089618895223,12.1993426730394));
#53402=CARTESIAN_POINT('Ctrl Pts',(18.7149849456307,71.6823568457297,12.2004008361423));
#53403=CARTESIAN_POINT('Ctrl Pts',(18.7167661545181,71.7009964481357,12.2010804528747));
#53404=CARTESIAN_POINT('Ctrl Pts',(18.7214712191112,71.7498942503459,12.2039427274346));
#53405=CARTESIAN_POINT('Ctrl Pts',(18.7244104326693,71.7800987532055,12.2067993152529));
#53406=CARTESIAN_POINT('Ctrl Pts',(18.7296657776108,71.8332681954377,12.2137563011357));
#53407=CARTESIAN_POINT('Ctrl Pts',(18.7319672570578,71.8562774919834,12.2174133974531));
#53408=CARTESIAN_POINT('Ctrl Pts',(18.7371035289255,71.9069302170527,12.2268992316055));
#53409=CARTESIAN_POINT('Ctrl Pts',(18.7399463531597,71.9345049480494,12.2330215904059));
#53410=CARTESIAN_POINT('Ctrl Pts',(18.7517212305061,72.0466684808723,12.2618799734655));
#53411=CARTESIAN_POINT('Ctrl Pts',(18.76088556572,72.1289843684963,12.292413420382));
#53412=CARTESIAN_POINT('Ctrl Pts',(18.7745076957934,72.2451074152659,12.3497272481955));
#53413=CARTESIAN_POINT('Ctrl Pts',(18.7789187575112,72.2817864543717,12.3701487751323));
#53414=CARTESIAN_POINT('Ctrl Pts',(18.7861460998922,72.3407787665375,12.4069345453571));
#53415=CARTESIAN_POINT('Ctrl Pts',(18.7889883744013,72.3636900159105,12.4222788567443));
#53416=CARTESIAN_POINT('Ctrl Pts',(18.7932539191645,72.3977732989133,12.4467495813929));
#53417=CARTESIAN_POINT('Ctrl Pts',(18.7947055623812,72.4093182927454,12.4553394999471));
#53418=CARTESIAN_POINT('Ctrl Pts',(18.79765988588,72.4327308716207,12.4733856214846));
#53419=CARTESIAN_POINT('Ctrl Pts',(18.799161083622,72.4445798921469,12.4828618626807));
#53420=CARTESIAN_POINT('Ctrl Pts',(18.8038846964512,72.4816240808016,12.5135923548317));
#53421=CARTESIAN_POINT('Ctrl Pts',(18.8070599379444,72.5061655313132,12.5356180770225));
#53422=CARTESIAN_POINT('Ctrl Pts',(18.8181491769481,72.589626760429,12.6166070242412));
#53423=CARTESIAN_POINT('Ctrl Pts',(18.8258747786941,72.6435749784694,12.6803848022371));
#53424=CARTESIAN_POINT('Ctrl Pts',(18.8369962934314,72.7103646447034,12.7772322428483));
#53425=CARTESIAN_POINT('Ctrl Pts',(18.8402585235291,72.7286867616725,12.8062483155181));
#53426=CARTESIAN_POINT('Ctrl Pts',(18.8464092783241,72.760621014105,12.861672662604));
#53427=CARTESIAN_POINT('Ctrl Pts',(18.8492866633893,72.7745246579151,12.8878855406901));
#53428=CARTESIAN_POINT('Ctrl Pts',(18.8544785763088,72.7976767306835,12.9354907707228));
#53429=CARTESIAN_POINT('Ctrl Pts',(18.8567798516853,72.8072784404918,12.9566968795014));
#53430=CARTESIAN_POINT('Ctrl Pts',(18.8619734812797,72.8274443636432,13.0047039062497));
#53431=CARTESIAN_POINT('Ctrl Pts',(18.8648750106071,72.8376898225921,13.0316234780821));
#53432=CARTESIAN_POINT('Ctrl Pts',(18.874154985656,72.8672079936783,13.1178953273526));
#53433=CARTESIAN_POINT('Ctrl Pts',(18.8806325976069,72.88302443744,13.178322757841));
#53434=CARTESIAN_POINT('Ctrl Pts',(18.8945920094353,72.907162704179,13.3092022408263));
#53435=CARTESIAN_POINT('Ctrl Pts',(18.9020704643738,72.9141583153627,13.3796993284569));
#53436=CARTESIAN_POINT('Ctrl Pts',(18.9119271978859,72.9156252207459,13.4748095522636));
#53437=CARTESIAN_POINT('Ctrl Pts',(18.9144347044341,72.9152984675103,13.4992127829934));
#53438=CARTESIAN_POINT('Ctrl Pts',(18.9183225146682,72.9136811563357,13.5375035484363));
#53439=CARTESIAN_POINT('Ctrl Pts',(18.9197240610293,72.9128649145516,13.5514039632831));
#53440=CARTESIAN_POINT('Ctrl Pts',(18.9227081539455,72.9106201564345,13.5812371619966));
#53441=CARTESIAN_POINT('Ctrl Pts',(18.9242869939796,72.9091190194082,13.5971616420481));
#53442=CARTESIAN_POINT('Ctrl Pts',(18.929530722707,72.9030850235207,13.6503887701341));
#53443=CARTESIAN_POINT('Ctrl Pts',(18.9331337968108,72.897197432332,13.6875217404613));
#53444=CARTESIAN_POINT('Ctrl Pts',(18.9441228428679,72.8740214460814,13.8009005427082));
#53445=CARTESIAN_POINT('Ctrl Pts',(18.9513787991395,72.8513400118167,13.8758514502966));
#53446=CARTESIAN_POINT('Ctrl Pts',(18.9619460712768,72.8092765171444,13.9793304067216));
#53447=CARTESIAN_POINT('Ctrl Pts',(18.9651397873988,72.7954142676102,14.0099007837454));
#53448=CARTESIAN_POINT('Ctrl Pts',(18.9711823650676,72.7672352881783,14.0660209236222));
#53449=CARTESIAN_POINT('Ctrl Pts',(18.9740209227945,72.7532139580133,14.0916938783444));
#53450=CARTESIAN_POINT('Ctrl Pts',(18.9791743639213,72.7264646398409,14.1368890864682));
#53451=CARTESIAN_POINT('Ctrl Pts',(18.9814768837008,72.7140614694285,14.1565888845649));
#53452=CARTESIAN_POINT('Ctrl Pts',(18.9867141739085,72.6848893052458,14.2002158102131));
#53453=CARTESIAN_POINT('Ctrl Pts',(18.9896589474522,72.667822523857,14.2239263740537));
#53454=CARTESIAN_POINT('Ctrl Pts',(18.9998431830052,72.6066430915271,14.3030204892916));
#53455=CARTESIAN_POINT('Ctrl Pts',(19.0072179822778,72.5587329792036,14.355285654541));
#53456=CARTESIAN_POINT('Ctrl Pts',(19.0200248069847,72.4691747571639,14.4379394528602));
#53457=CARTESIAN_POINT('Ctrl Pts',(19.0254134155555,72.4295610924943,14.4703016448822));
#53458=CARTESIAN_POINT('Ctrl Pts',(19.0330524297008,72.3701141356545,14.5131592691046));
#53459=CARTESIAN_POINT('Ctrl Pts',(19.035351029317,72.3517862866908,14.525656387916));
#53460=CARTESIAN_POINT('Ctrl Pts',(19.0394926614683,72.3178742720979,14.5475008370576));
#53461=CARTESIAN_POINT('Ctrl Pts',(19.0413422669862,72.3023988252927,14.5570061498825));
#53462=CARTESIAN_POINT('Ctrl Pts',(19.0445271916547,72.2751189450706,14.5729663671099));
#53463=CARTESIAN_POINT('Ctrl Pts',(19.0458704314388,72.2634077516452,14.5795707397645));
#53464=CARTESIAN_POINT('Ctrl Pts',(19.0491881848486,72.2339835554525,14.595553612684));
#53465=CARTESIAN_POINT('Ctrl Pts',(19.0511494896536,72.2161494795621,14.604701164699));
#53466=CARTESIAN_POINT('Ctrl Pts',(19.0555730049531,72.1750771373837,14.6245545847283));
#53467=CARTESIAN_POINT('Ctrl Pts',(19.0580229246198,72.1517166425684,14.6349883476451));
#53468=CARTESIAN_POINT('Ctrl Pts',(19.0671648340642,72.0627933775437,14.6715243794105));
#53469=CARTESIAN_POINT('Ctrl Pts',(19.0737308568641,71.9954078705765,14.692854692719));
#53470=CARTESIAN_POINT('Ctrl Pts',(19.0853488019237,71.8752269736946,14.7201417605105));
#53471=CARTESIAN_POINT('Ctrl Pts',(19.0903495753432,71.8231882922918,14.7285964163104));
#53472=CARTESIAN_POINT('Ctrl Pts',(19.0979928876443,71.7445804236849,14.7363950571698));
#53473=CARTESIAN_POINT('Ctrl Pts',(19.1005616591792,71.7183083081137,14.7381787483975));
#53474=CARTESIAN_POINT('Ctrl Pts',(19.1054780163233,71.6684508723498,14.7400094711514));
#53475=CARTESIAN_POINT('Ctrl Pts',(19.1078195703161,71.644882395617,14.7402184640046));
#53476=CARTESIAN_POINT('Ctrl Pts',(19.1135665775289,71.5875599318104,14.7391315632282));
#53477=CARTESIAN_POINT('Ctrl Pts',(19.1169914913882,71.5538394041259,14.737145029325));
#53478=CARTESIAN_POINT('Ctrl Pts',(19.1227208930491,71.4982410112389,14.7316390191867));
#53479=CARTESIAN_POINT('Ctrl Pts',(19.1250029603896,71.4763023249277,14.7288862670089));
#53480=CARTESIAN_POINT('Ctrl Pts',(19.1351975063417,71.3792071612724,14.7141195697546));
#53481=CARTESIAN_POINT('Ctrl Pts',(19.1432393733349,71.3051513326321,14.6959368624199));
#53482=CARTESIAN_POINT('Ctrl Pts',(19.1552241639399,71.1969783564105,14.6588156635142));
#53483=CARTESIAN_POINT('Ctrl Pts',(19.1592094370848,71.1613551992887,14.6447620975226));
#53484=CARTESIAN_POINT('Ctrl Pts',(19.1648498746406,71.1110730828369,14.622248841776));
#53485=CARTESIAN_POINT('Ctrl Pts',(19.1665577966296,71.0958652805527,14.6150739468854));
#53486=CARTESIAN_POINT('Ctrl Pts',(19.1696202560236,71.0685826219487,14.6015334010914));
#53487=CARTESIAN_POINT('Ctrl Pts',(19.1709796977349,71.056461313854,14.5952721391617));
#53488=CARTESIAN_POINT('Ctrl Pts',(19.1745285607266,71.0248314318002,14.5782825235474));
#53489=CARTESIAN_POINT('Ctrl Pts',(19.1766996991741,71.0054996511563,14.5672343682509));
#53490=CARTESIAN_POINT('Ctrl Pts',(19.1803606290721,70.9731002478418,14.5475701849106));
#53491=CARTESIAN_POINT('Ctrl Pts',(19.1818604638763,70.9598843983955,14.539211332752));
#53492=CARTESIAN_POINT('Ctrl Pts',(19.1885942748069,70.9009588723045,14.5003998358305));
#53493=CARTESIAN_POINT('Ctrl Pts',(19.1937372306643,70.8570966217514,14.4672437627804));
#53494=CARTESIAN_POINT('Ctrl Pts',(19.2047114100082,70.7686518367894,14.3908938985588));
#53495=CARTESIAN_POINT('Ctrl Pts',(19.2105330337721,70.7248176249402,14.3470737148405));
#53496=CARTESIAN_POINT('Ctrl Pts',(19.2164763792089,70.6843589395965,14.3002409771978));
#53497=CARTESIAN_POINT('Ctrl Pts',(19.3867992156006,70.6843590974191,14.3002411598846));
#53498=CARTESIAN_POINT('Ctrl Pts',(19.3835334172154,70.7070796831207,14.3265412438178));
#53499=CARTESIAN_POINT('Ctrl Pts',(19.3802671931033,70.7308851081539,14.3519147508244));
#53500=CARTESIAN_POINT('Ctrl Pts',(19.3723650013119,70.7905264941611,14.4104628088744));
#53501=CARTESIAN_POINT('Ctrl Pts',(19.3677158978359,70.827268187921,14.4425935784481));
#53502=CARTESIAN_POINT('Ctrl Pts',(19.3605099636473,70.8858973050198,14.4881877372903));
#53503=CARTESIAN_POINT('Ctrl Pts',(19.3580149054582,70.9064977957848,14.5032346906094));
#53504=CARTESIAN_POINT('Ctrl Pts',(19.3531450225679,70.947173496373,14.5311062455875));
#53505=CARTESIAN_POINT('Ctrl Pts',(19.3507742593599,70.9671841027914,14.5440063877134));
#53506=CARTESIAN_POINT('Ctrl Pts',(19.3446757316856,71.0191051148364,14.5754483869345));
#53507=CARTESIAN_POINT('Ctrl Pts',(19.3409214743082,71.0514802001727,14.593174079633));
#53508=CARTESIAN_POINT('Ctrl Pts',(19.3280588222347,71.1636000090351,14.6483573920042));
#53509=CARTESIAN_POINT('Ctrl Pts',(19.318762402838,71.2464457944114,14.6789204257536));
#53510=CARTESIAN_POINT('Ctrl Pts',(19.3063063127941,71.3614685626476,14.7082335091833));
#53511=CARTESIAN_POINT('Ctrl Pts',(19.3031033733097,71.3914336600095,14.7147251387834));
#53512=CARTESIAN_POINT('Ctrl Pts',(19.2975911306912,71.4439042367553,14.7241182488114));
#53513=CARTESIAN_POINT('Ctrl Pts',(19.2952677222421,71.4663072489211,14.7275130730426));
#53514=CARTESIAN_POINT('Ctrl Pts',(19.2915852361487,71.5023810329232,14.7319956835361));
#53515=CARTESIAN_POINT('Ctrl Pts',(19.2902086670708,71.5159983745807,14.7334646177926));
#53516=CARTESIAN_POINT('Ctrl Pts',(19.2871920134304,71.5461564877241,14.7362250368024));
#53517=CARTESIAN_POINT('Ctrl Pts',(19.2855571924625,71.5627037056621,14.7374133278357));
#53518=CARTESIAN_POINT('Ctrl Pts',(19.2798939294452,71.6205847241462,14.7404312921623));
#53519=CARTESIAN_POINT('Ctrl Pts',(19.2759410503684,71.6619852170594,14.7405657764868));
#53520=CARTESIAN_POINT('Ctrl Pts',(19.2649967634848,71.7774643625782,14.7352933445566));
#53521=CARTESIAN_POINT('Ctrl Pts',(19.2580987963386,71.8511656874217,14.7254159256175));
#53522=CARTESIAN_POINT('Ctrl Pts',(19.2490087100834,71.9448882572721,14.7043757712989));
#53523=CARTESIAN_POINT('Ctrl Pts',(19.2469338402253,71.9660649296679,14.6990446188099));
#53524=CARTESIAN_POINT('Ctrl Pts',(19.2416456260955,72.0193236852016,14.6841667848063));
#53525=CARTESIAN_POINT('Ctrl Pts',(19.238416575831,72.0511827708328,14.6738936030261));
#53526=CARTESIAN_POINT('Ctrl Pts',(19.2328575530865,72.104602285102,14.6543068169986));
#53527=CARTESIAN_POINT('Ctrl Pts',(19.2305491570999,72.126378954612,14.6456310826091));
#53528=CARTESIAN_POINT('Ctrl Pts',(19.2256146017602,72.1719849569639,14.6259826805042));
#53529=CARTESIAN_POINT('Ctrl Pts',(19.2229844897638,72.1957389324514,14.6148643921935));
#53530=CARTESIAN_POINT('Ctrl Pts',(19.2146917655003,72.2688048503666,14.5778658517363));
#53531=CARTESIAN_POINT('Ctrl Pts',(19.2089482398177,72.3167629617254,14.5494767475252));
#53532=CARTESIAN_POINT('Ctrl Pts',(19.1959625531235,72.4193547329688,14.4792610613385));
#53533=CARTESIAN_POINT('Ctrl Pts',(19.1887013054433,72.4727722286487,14.4359547019324));
#53534=CARTESIAN_POINT('Ctrl Pts',(19.1788758673769,72.5407109939177,14.3710867405461));
#53535=CARTESIAN_POINT('Ctrl Pts',(19.1762454420603,72.5584714221768,14.3530854277425));
#53536=CARTESIAN_POINT('Ctrl Pts',(19.171594545553,72.5892051859747,14.3200154530666));
#53537=CARTESIAN_POINT('Ctrl Pts',(19.1695648353517,72.6023846532207,14.3051497058049));
#53538=CARTESIAN_POINT('Ctrl Pts',(19.1662046464435,72.6238594666724,14.279750880089));
#53539=CARTESIAN_POINT('Ctrl Pts',(19.1648624754853,72.6323455915356,14.2693859415454));
#53540=CARTESIAN_POINT('Ctrl Pts',(19.1617611329487,72.6517375256676,14.2449208857967));
#53541=CARTESIAN_POINT('Ctrl Pts',(19.160010246894,72.6625133959531,14.2307220622127));
#53542=CARTESIAN_POINT('Ctrl Pts',(19.1509426712797,72.7172310820457,14.1553807178038));
#53543=CARTESIAN_POINT('Ctrl Pts',(19.143894823342,72.7559774795807,14.0906369583843));
#53544=CARTESIAN_POINT('Ctrl Pts',(19.1303175689313,72.818911238099,13.9604775362638));
#53545=CARTESIAN_POINT('Ctrl Pts',(19.1238142214403,72.84390514277,13.8957704017116));
#53546=CARTESIAN_POINT('Ctrl Pts',(19.1143394148699,72.8717646259092,13.8013354538625));
#53547=CARTESIAN_POINT('Ctrl Pts',(19.1115039033327,72.879060527093,13.77304252555));
#53548=CARTESIAN_POINT('Ctrl Pts',(19.1063506160155,72.8904118553302,13.7217710012879));
#53549=CARTESIAN_POINT('Ctrl Pts',(19.1040450788607,72.8948219270255,13.6988838750791));
#53550=CARTESIAN_POINT('Ctrl Pts',(19.0987925361396,72.9033543897519,13.6469490137557));
#53551=CARTESIAN_POINT('Ctrl Pts',(19.0958353489916,72.9071046998967,13.6178549847112));
#53552=CARTESIAN_POINT('Ctrl Pts',(19.0894161910244,72.9129929155851,13.5551100496096));
#53553=CARTESIAN_POINT('Ctrl Pts',(19.0859471218489,72.9148045023225,13.5214516022515));
#53554=CARTESIAN_POINT('Ctrl Pts',(19.0742303435482,72.9163828165642,13.408626133998));
#53555=CARTESIAN_POINT('Ctrl Pts',(19.0658611661164,72.9100893775512,13.3295609693194));
#53556=CARTESIAN_POINT('Ctrl Pts',(19.0538693498735,72.8903750437942,13.2166270079168));
#53557=CARTESIAN_POINT('Ctrl Pts',(19.0501809790984,72.882804174797,13.1819162505287));
#53558=CARTESIAN_POINT('Ctrl Pts',(19.0448997172875,72.8696841659878,13.1319327399609));
#53559=CARTESIAN_POINT('Ctrl Pts',(19.043260721097,72.8652826184975,13.1163791825758));
#53560=CARTESIAN_POINT('Ctrl Pts',(19.0402436319074,72.8565492115874,13.0876252813873));
#53561=CARTESIAN_POINT('Ctrl Pts',(19.0388622495715,72.8522960385402,13.074405728853));
#53562=CARTESIAN_POINT('Ctrl Pts',(19.035117765819,72.8400834202761,13.0384790878007));
#53563=CARTESIAN_POINT('Ctrl Pts',(19.0327771621028,72.8316940318986,13.0159234595001));
#53564=CARTESIAN_POINT('Ctrl Pts',(19.02366998032,72.7962316099296,12.9282864123973));
#53565=CARTESIAN_POINT('Ctrl Pts',(19.0170869015605,72.7643997805837,12.8652612611433));
#53566=CARTESIAN_POINT('Ctrl Pts',(19.0045421227482,72.6945057156641,12.7514948773903));
#53567=CARTESIAN_POINT('Ctrl Pts',(18.9986062259607,72.6575653927919,12.7003299088967));
#53568=CARTESIAN_POINT('Ctrl Pts',(18.9897603435738,72.5984021476572,12.6300479386718));
#53569=CARTESIAN_POINT('Ctrl Pts',(18.9869580827932,72.5790750827161,12.608615592185));
#53570=CARTESIAN_POINT('Ctrl Pts',(18.9818403476615,72.5428670831154,12.5711147153745));
#53571=CARTESIAN_POINT('Ctrl Pts',(18.9795364134486,72.5262414254013,12.5548168889939));
#53572=CARTESIAN_POINT('Ctrl Pts',(18.974255651198,72.4874683691361,12.5188439049089));
#53573=CARTESIAN_POINT('Ctrl Pts',(18.9712679912811,72.4650625735697,12.4994692398638));
#53574=CARTESIAN_POINT('Ctrl Pts',(18.9647634159167,72.4153591063018,12.4594391208407));
#53575=CARTESIAN_POINT('Ctrl Pts',(18.9612388917027,72.3878625187693,12.4390687497138));
#53576=CARTESIAN_POINT('Ctrl Pts',(18.9491014393378,72.2912839867501,12.3733891071756));
#53577=CARTESIAN_POINT('Ctrl Pts',(18.9403558203981,72.2186214255504,12.3337178595366));
#53578=CARTESIAN_POINT('Ctrl Pts',(18.9283418743341,72.1127763948276,12.2886820971379));
#53579=CARTESIAN_POINT('Ctrl Pts',(18.9249781396343,72.0824419792335,12.2771263742594));
#53580=CARTESIAN_POINT('Ctrl Pts',(18.9200618800202,72.0368182962898,12.2617209508099));
#53581=CARTESIAN_POINT('Ctrl Pts',(18.9184710891769,72.0218485675283,12.2569735752404));
#53582=CARTESIAN_POINT('Ctrl Pts',(18.9154869129122,71.9933298926065,12.2485082786859));
#53583=CARTESIAN_POINT('Ctrl Pts',(18.9140912663641,71.9798014736675,12.244735567167));
#53584=CARTESIAN_POINT('Ctrl Pts',(18.9102135005467,71.9417415770098,12.2347991018166));
#53585=CARTESIAN_POINT('Ctrl Pts',(18.9077569843954,71.91708341829,12.2291422290321));
#53586=CARTESIAN_POINT('Ctrl Pts',(18.8984085658149,71.8217219741621,12.2102448562571));
#53587=CARTESIAN_POINT('Ctrl Pts',(18.8916998279305,71.7501058354853,12.2022809748681));
#53588=CARTESIAN_POINT('Ctrl Pts',(18.8792840033826,71.6180414770388,12.1988697204498));
#53589=CARTESIAN_POINT('Ctrl Pts',(18.8736092625322,71.5578624743169,12.2015929706202));
#53590=CARTESIAN_POINT('Ctrl Pts',(18.8650594582929,71.4696977367608,12.2118875665636));
#53591=CARTESIAN_POINT('Ctrl Pts',(18.8622806145463,71.4414098282073,12.2161635289731));
#53592=CARTESIAN_POINT('Ctrl Pts',(18.8571879752119,71.3904233093375,12.225641541198));
#53593=CARTESIAN_POINT('Ctrl Pts',(18.8548852384085,71.3676769078525,12.2305199500766));
#53594=CARTESIAN_POINT('Ctrl Pts',(18.8495836494129,71.3160965154503,12.2430733693154));
#53595=CARTESIAN_POINT('Ctrl Pts',(18.8465734819824,71.2873747069891,12.2511451033514));
#53596=CARTESIAN_POINT('Ctrl Pts',(18.8400040797361,71.225999086447,12.2707499774348));
#53597=CARTESIAN_POINT('Ctrl Pts',(18.8364368254665,71.1934795449908,12.282622574761));
#53598=CARTESIAN_POINT('Ctrl Pts',(18.823935902502,71.0823117180925,12.3284373388257));
#53599=CARTESIAN_POINT('Ctrl Pts',(18.8148601818198,71.0066449877238,12.368989461398));
#53600=CARTESIAN_POINT('Ctrl Pts',(18.8027178693168,70.9100520828578,12.4340871836399));
#53601=CARTESIAN_POINT('Ctrl Pts',(18.7995271528156,70.8851004929632,12.4522588535239));
#53602=CARTESIAN_POINT('Ctrl Pts',(18.7948697603024,70.8491387638335,12.4805106378641));
#53603=CARTESIAN_POINT('Ctrl Pts',(18.7933667202013,70.8376058556007,12.489903141957));
#53604=CARTESIAN_POINT('Ctrl Pts',(18.7904143244938,70.8150668434862,12.508927362591));
#53605=CARTESIAN_POINT('Ctrl Pts',(18.7889648188221,70.8040568498784,12.5185508227034));
#53606=CARTESIAN_POINT('Ctrl Pts',(18.784663942629,70.7716272204922,12.5478997721756));
#53607=CARTESIAN_POINT('Ctrl Pts',(18.7818482492416,70.7507152604635,12.5681755475808));
#53608=CARTESIAN_POINT('Ctrl Pts',(18.7746483999433,70.6985451674196,12.6223616481549));
#53609=CARTESIAN_POINT('Ctrl Pts',(18.7703116485295,70.6684027017918,12.6572873441909));
#53610=CARTESIAN_POINT('Ctrl Pts',(18.7585556056968,70.5919216516156,12.7563271567465));
#53611=CARTESIAN_POINT('Ctrl Pts',(18.7511640655145,70.5495687772447,12.8232409382886));
#53612=CARTESIAN_POINT('Ctrl Pts',(18.7407699886034,70.5005699321449,12.9194525237505));
#53613=CARTESIAN_POINT('Ctrl Pts',(18.7379584565224,70.4883170101541,12.9456937354539));
#53614=CARTESIAN_POINT('Ctrl Pts',(18.7328321304185,70.4678521641224,12.9937408611873));
#53615=CARTESIAN_POINT('Ctrl Pts',(18.7305290970881,70.4593230011766,13.0153981419959));
#53616=CARTESIAN_POINT('Ctrl Pts',(18.7252616144557,70.4413441281442,13.0650068237519));
#53617=CARTESIAN_POINT('Ctrl Pts',(18.7222865689622,70.4322642568377,13.093076501623));
#53618=CARTESIAN_POINT('Ctrl Pts',(18.7158166358718,70.4148377236653,13.1541317813105));
#53619=CARTESIAN_POINT('Ctrl Pts',(18.7123143314326,70.4068230111986,13.1871876657736));
#53620=CARTESIAN_POINT('Ctrl Pts',(18.7003464736732,70.3841940147418,13.3001389914435));
#53621=CARTESIAN_POINT('Ctrl Pts',(18.6917527005371,70.3759165010865,13.3810998188951));
#53622=CARTESIAN_POINT('Ctrl Pts',(18.6797501782105,70.3752190653075,13.495934949769));
#53623=CARTESIAN_POINT('Ctrl Pts',(18.6762586192099,70.3763520245786,13.5295818994106));
#53624=CARTESIAN_POINT('Ctrl Pts',(18.6711961982458,70.3799870492725,13.579009208535));
#53625=CARTESIAN_POINT('Ctrl Pts',(18.6695840960226,70.3814514898272,13.5948486988157));
#53626=CARTESIAN_POINT('Ctrl Pts',(18.666586969508,70.3847591501794,13.6245298308791));
#53627=CARTESIAN_POINT('Ctrl Pts',(18.6651992053597,70.3865335358021,13.6383748335243));
#53628=CARTESIAN_POINT('Ctrl Pts',(18.6613906152334,70.3920730347633,13.6765899379778));
#53629=CARTESIAN_POINT('Ctrl Pts',(18.6589937916027,70.3963202053588,13.7008848856826));
#53630=CARTESIAN_POINT('Ctrl Pts',(18.6497808092936,70.4155432923951,13.794657012063));
#53631=CARTESIAN_POINT('Ctrl Pts',(18.6431473560594,70.4356331538749,13.8629583712339));
#53632=CARTESIAN_POINT('Ctrl Pts',(18.6306681141832,70.483656522586,13.986781233989));
#53633=CARTESIAN_POINT('Ctrl Pts',(18.6248507353769,70.5101420777077,14.0426243712303));
#53634=CARTESIAN_POINT('Ctrl Pts',(18.6161388635988,70.5547556313678,14.1213226222846));
#53635=CARTESIAN_POINT('Ctrl Pts',(18.6133467919828,70.5697753109458,14.1458383886472));
#53636=CARTESIAN_POINT('Ctrl Pts',(18.6082398745516,70.5984364656055,14.1892419418408));
#53637=CARTESIAN_POINT('Ctrl Pts',(18.6059363573694,70.611790888589,14.2083045721645));
#53638=CARTESIAN_POINT('Ctrl Pts',(18.6006461328833,70.6433697818026,14.2508445396661));
#53639=CARTESIAN_POINT('Ctrl Pts',(18.5976483805331,70.6619089636197,14.2740695035649));
#53640=CARTESIAN_POINT('Ctrl Pts',(18.5944580111549,70.682279675732,14.2978295571791));
#53641=CARTESIAN_POINT('Ctrl Pts',(18.594295635599,70.6833181886463,14.2990362614413));
#53642=CARTESIAN_POINT('Ctrl Pts',(18.5941331801233,70.6843589436049,14.3002409818378));
#53643=CARTESIAN_POINT('Origin',(21.26284859951,71.6454,13.47));
#53644=CARTESIAN_POINT('',(17.6289974407812,70.6843588693663,14.3002408959033));
#53645=CARTESIAN_POINT('',(17.7982694921739,70.6843589433904,14.3002409815896));
#53646=CARTESIAN_POINT('',(21.26284859951,70.6843589433668,14.3002409815622));
#53647=CARTESIAN_POINT('',(18.3157450659502,71.646363655002,14.7399998049553));
#53648=CARTESIAN_POINT('Ctrl Pts',(17.6289974407812,70.6843588693663,14.3002408959033));
#53649=CARTESIAN_POINT('Ctrl Pts',(17.6346389774939,70.6485735080814,14.2588177327719));
#53650=CARTESIAN_POINT('Ctrl Pts',(17.6403669691112,70.6154972945373,14.215116859955));
#53651=CARTESIAN_POINT('Ctrl Pts',(17.6533971916263,70.5472400007928,14.1116625438007));
#53652=CARTESIAN_POINT('Ctrl Pts',(17.6606960210929,70.5139186929955,14.0508942837002));
#53653=CARTESIAN_POINT('Ctrl Pts',(17.6695292415001,70.4788740695717,13.9723928410434));
#53654=CARTESIAN_POINT('Ctrl Pts',(17.6712402932642,70.4723403708938,13.9569420051821));
#53655=CARTESIAN_POINT('Ctrl Pts',(17.6742947714227,70.4611201916754,13.9288707664881));
#53656=CARTESIAN_POINT('Ctrl Pts',(17.6756432994331,70.4563248994782,13.9162975721615));
#53657=CARTESIAN_POINT('Ctrl Pts',(17.6787762667129,70.4455579271645,13.8866601624838));
#53658=CARTESIAN_POINT('Ctrl Pts',(17.6805519707749,70.4397490289603,13.8695404276859));
#53659=CARTESIAN_POINT('Ctrl Pts',(17.6844573943771,70.4276747265706,13.8312901816871));
#53660=CARTESIAN_POINT('Ctrl Pts',(17.6865788759155,70.4215896721122,13.8101086373422));
#53661=CARTESIAN_POINT('Ctrl Pts',(17.6935028490101,70.4034042156482,13.7399778279591));
#53662=CARTESIAN_POINT('Ctrl Pts',(17.6982342791462,70.3936659435074,13.6904636943652));
#53663=CARTESIAN_POINT('Ctrl Pts',(17.7097112951337,70.3772591901405,13.569359941036));
#53664=CARTESIAN_POINT('Ctrl Pts',(17.7164446483401,70.3736716260103,13.4975414310448));
#53665=CARTESIAN_POINT('Ctrl Pts',(17.7261618985194,70.3771853059989,13.396620296412));
#53666=CARTESIAN_POINT('Ctrl Pts',(17.7289968140244,70.37920815591,13.3674768579708));
#53667=CARTESIAN_POINT('Ctrl Pts',(17.7341460687762,70.3846442786766,13.3152855468846));
#53668=CARTESIAN_POINT('Ctrl Pts',(17.7364481141296,70.3876906327177,13.2922121436989));
#53669=CARTESIAN_POINT('Ctrl Pts',(17.741687251276,70.3959896419891,13.2403737581136));
#53670=CARTESIAN_POINT('Ctrl Pts',(17.7446344040215,70.4016051254094,13.2116815679193));
#53671=CARTESIAN_POINT('Ctrl Pts',(17.7510262896919,70.4157765058223,13.1505467534375));
#53672=CARTESIAN_POINT('Ctrl Pts',(17.7544779948524,70.4246381795664,13.1181983032634));
#53673=CARTESIAN_POINT('Ctrl Pts',(17.7660552335088,70.4583289762784,13.0119149312245));
#53674=CARTESIAN_POINT('Ctrl Pts',(17.7742991018947,70.4886837105304,12.9399196243682));
#53675=CARTESIAN_POINT('Ctrl Pts',(17.7864128375122,70.543238359833,12.8378892576638));
#53676=CARTESIAN_POINT('Ctrl Pts',(17.7903369087447,70.5625102307927,12.8054138628221));
#53677=CARTESIAN_POINT('Ctrl Pts',(17.7958322287774,70.5919900250051,12.7604336429856));
#53678=CARTESIAN_POINT('Ctrl Pts',(17.7974577246906,70.6010313571855,12.7471921273928));
#53679=CARTESIAN_POINT('Ctrl Pts',(17.8004628021912,70.6183768110263,12.7227941224856));
#53680=CARTESIAN_POINT('Ctrl Pts',(17.8018454348783,70.6266169225172,12.7115975128283));
#53681=CARTESIAN_POINT('Ctrl Pts',(17.8056100922388,70.6497350268353,12.6812418018446));
#53682=CARTESIAN_POINT('Ctrl Pts',(17.8079690951011,70.6649810721522,12.662369374025));
#53683=CARTESIAN_POINT('Ctrl Pts',(17.8170962709051,70.7266277224934,12.5903805983487));
#53684=CARTESIAN_POINT('Ctrl Pts',(17.8236819544005,70.7768824870622,12.5407247208408));
#53685=CARTESIAN_POINT('Ctrl Pts',(17.8362032511098,70.8791482612832,12.4552613237198));
#53686=CARTESIAN_POINT('Ctrl Pts',(17.8421126389966,70.9301995577544,12.4186565433208));
#53687=CARTESIAN_POINT('Ctrl Pts',(17.8509285564544,71.0083498696919,12.3709557235073));
#53688=CARTESIAN_POINT('Ctrl Pts',(17.8537285068914,71.0334603257136,12.3567791211486));
#53689=CARTESIAN_POINT('Ctrl Pts',(17.8588434776343,71.0796748595025,12.3327239587012));
#53690=CARTESIAN_POINT('Ctrl Pts',(17.8611469967352,71.100610307492,12.3225481522738));
#53691=CARTESIAN_POINT('Ctrl Pts',(17.8664287030941,71.1488054765756,12.3007388025683));
#53692=CARTESIAN_POINT('Ctrl Pts',(17.8694177609855,71.1762153265732,12.289473318576));
#53693=CARTESIAN_POINT('Ctrl Pts',(17.8759268747967,71.2360967077403,12.2672767542085));
#53694=CARTESIAN_POINT('Ctrl Pts',(17.8794545760762,71.2686668367627,12.2566805727704));
#53695=CARTESIAN_POINT('Ctrl Pts',(17.8916235674072,71.3813929910568,12.2249831889868));
#53696=CARTESIAN_POINT('Ctrl Pts',(17.9003984218593,71.4631661037746,12.2104144687572));
#53697=CARTESIAN_POINT('Ctrl Pts',(17.9125379967623,71.5790644495894,12.2012938538969));
#53698=CARTESIAN_POINT('Ctrl Pts',(17.9159990360092,71.6124581337761,12.1999877654215));
#53699=CARTESIAN_POINT('Ctrl Pts',(17.9209577942149,71.6610966323201,12.2000057022075));
#53700=CARTESIAN_POINT('Ctrl Pts',(17.9224985391921,71.6763249412809,12.200285217019));
#53701=CARTESIAN_POINT('Ctrl Pts',(17.9254620409761,71.7058831297117,12.2013599326175));
#53702=CARTESIAN_POINT('Ctrl Pts',(17.9268859070433,71.7202114131176,12.2021241645522));
#53703=CARTESIAN_POINT('Ctrl Pts',(17.9309845729074,71.7617436911101,12.205045973));
#53704=CARTESIAN_POINT('Ctrl Pts',(17.9336287166111,71.78889732772,12.2078377983099));
#53705=CARTESIAN_POINT('Ctrl Pts',(17.9402026343141,71.8568121087723,12.2170411543457));
#53706=CARTESIAN_POINT('Ctrl Pts',(17.944094941471,71.8973908433042,12.2245674752926));
#53707=CARTESIAN_POINT('Ctrl Pts',(17.9563652086868,72.0243511397494,12.2545765242186));
#53708=CARTESIAN_POINT('Ctrl Pts',(17.9646784241461,72.1087534135119,12.2841841545359));
#53709=CARTESIAN_POINT('Ctrl Pts',(17.9759850837983,72.2147211298855,12.3344113317521));
#53710=CARTESIAN_POINT('Ctrl Pts',(17.9787150497899,72.2396819697554,12.3472725921183));
#53711=CARTESIAN_POINT('Ctrl Pts',(17.9837640665872,72.2845481889901,12.3723056652532));
#53712=CARTESIAN_POINT('Ctrl Pts',(17.9860732187937,72.3045840240859,12.3842194032067));
#53713=CARTESIAN_POINT('Ctrl Pts',(17.9914568728277,72.3501079195851,12.4130133585766));
#53714=CARTESIAN_POINT('Ctrl Pts',(17.9945441413881,72.3753355944863,12.4302752090745));
#53715=CARTESIAN_POINT('Ctrl Pts',(17.9995895710402,72.4150937784589,12.4596398541954));
#53716=CARTESIAN_POINT('Ctrl Pts',(18.001527366384,72.4300211243848,12.4711878335554));
#53717=CARTESIAN_POINT('Ctrl Pts',(18.0092467665939,72.4881275980583,12.5182461973859));
#53718=CARTESIAN_POINT('Ctrl Pts',(18.0151038192601,72.5291952001873,12.5562550686432));
#53719=CARTESIAN_POINT('Ctrl Pts',(18.0277676721154,72.6119813358572,12.6436928755246));
#53720=CARTESIAN_POINT('Ctrl Pts',(18.0345653015757,72.6527108656485,12.6938624462724));
#53721=CARTESIAN_POINT('Ctrl Pts',(18.0431239767362,72.7001203159455,12.7623164442262));
#53722=CARTESIAN_POINT('Ctrl Pts',(18.0450342872524,72.7104455995707,12.7779530602499));
#53723=CARTESIAN_POINT('Ctrl Pts',(18.0482779914553,72.7275696059023,12.8051773473902));
#53724=CARTESIAN_POINT('Ctrl Pts',(18.0496205462495,72.7345365027106,12.8166532688021));
#53725=CARTESIAN_POINT('Ctrl Pts',(18.0528729390209,72.751109138655,12.8449540178626));
#53726=CARTESIAN_POINT('Ctrl Pts',(18.0547710939944,72.7605143396402,12.8618920000066));
#53727=CARTESIAN_POINT('Ctrl Pts',(18.0590156276763,72.7808555690324,12.9005852779468));
#53728=CARTESIAN_POINT('Ctrl Pts',(18.0613512102647,72.791561172505,12.9224534259517));
#53729=CARTESIAN_POINT('Ctrl Pts',(18.0696376337968,72.8275514280754,13.0016587942693));
#53730=CARTESIAN_POINT('Ctrl Pts',(18.0754851951364,72.8492154947339,13.0605433269499));
#53731=CARTESIAN_POINT('Ctrl Pts',(18.0872087205534,72.8834922402098,13.1803951172995));
#53732=CARTESIAN_POINT('Ctrl Pts',(18.0930682250896,72.8961493751874,13.2411602912818));
#53733=CARTESIAN_POINT('Ctrl Pts',(18.1016400192758,72.9078348968004,13.3290405035049));
#53734=CARTESIAN_POINT('Ctrl Pts',(18.1042406037443,72.9105165338626,13.3555825269681));
#53735=CARTESIAN_POINT('Ctrl Pts',(18.1091814819325,72.9139853824082,13.4056309028339));
#53736=CARTESIAN_POINT('Ctrl Pts',(18.1115149711916,72.914959113901,13.429113253711));
#53737=CARTESIAN_POINT('Ctrl Pts',(18.1171759757326,72.9157330273195,13.4856181668505));
#53738=CARTESIAN_POINT('Ctrl Pts',(18.1205213177689,72.9148977504257,13.5186301553941));
#53739=CARTESIAN_POINT('Ctrl Pts',(18.1280597341658,72.9101715518525,13.5920638626517));
#53740=CARTESIAN_POINT('Ctrl Pts',(18.1322673423076,72.9056262255898,13.6324063010571));
#53741=CARTESIAN_POINT('Ctrl Pts',(18.1440167519786,72.8877075829968,13.7433709623424));
#53742=CARTESIAN_POINT('Ctrl Pts',(18.1516163840293,72.8702612544447,13.8131829284471));
#53743=CARTESIAN_POINT('Ctrl Pts',(18.162343436967,72.8369511893909,13.9105344689111));
#53744=CARTESIAN_POINT('Ctrl Pts',(18.1655562045799,72.8258191547202,13.9395486564026));
#53745=CARTESIAN_POINT('Ctrl Pts',(18.1702389940427,72.8077854020337,13.9818421937544));
#53746=CARTESIAN_POINT('Ctrl Pts',(18.1717458793826,72.8016964699614,13.9954529522606));
#53747=CARTESIAN_POINT('Ctrl Pts',(18.1747004474569,72.7891713552702,14.0221778257484));
#53748=CARTESIAN_POINT('Ctrl Pts',(18.1761483551711,72.7827458861653,14.0352943178888));
#53749=CARTESIAN_POINT('Ctrl Pts',(18.1804357150977,72.7628935658343,14.0741098048386));
#53750=CARTESIAN_POINT('Ctrl Pts',(18.1832398383454,72.7488103961094,14.0994652055762));
#53751=CARTESIAN_POINT('Ctrl Pts',(18.1903959229063,72.7102975847404,14.1635318352467));
#53752=CARTESIAN_POINT('Ctrl Pts',(18.1947012106833,72.6846216048335,14.2014454540741));
#53753=CARTESIAN_POINT('Ctrl Pts',(18.2064854929538,72.6087834121687,14.3013478136545));
#53754=CARTESIAN_POINT('Ctrl Pts',(18.2139348965897,72.5547559660465,14.3601214992592));
#53755=CARTESIAN_POINT('Ctrl Pts',(18.2243869937911,72.4741059595387,14.4327992438687));
#53756=CARTESIAN_POINT('Ctrl Pts',(18.2271945836077,72.4519749014625,14.4514135608194));
#53757=CARTESIAN_POINT('Ctrl Pts',(18.2323169863518,72.4109178926607,14.4836192678949));
#53758=CARTESIAN_POINT('Ctrl Pts',(18.2346201247594,72.3922159986472,14.4974762049277));
#53759=CARTESIAN_POINT('Ctrl Pts',(18.2398921452152,72.3489374213081,14.5277370350171));
#53760=CARTESIAN_POINT('Ctrl Pts',(18.2428717145256,72.3241488654784,14.5438119733176));
#53761=CARTESIAN_POINT('Ctrl Pts',(18.2493542191822,72.2696028445018,14.5765406381842));
#53762=CARTESIAN_POINT('Ctrl Pts',(18.2528646451282,72.2396899265245,14.592889300668));
#53763=CARTESIAN_POINT('Ctrl Pts',(18.2648947632856,72.1359399545737,14.6442858327836));
#53764=CARTESIAN_POINT('Ctrl Pts',(18.2735443444823,72.0593933250985,14.6734053758334));
#53765=CARTESIAN_POINT('Ctrl Pts',(18.2855500966007,71.9485704074341,14.7037299972732));
#53766=CARTESIAN_POINT('Ctrl Pts',(18.2889936515305,71.9162159239663,14.7112337651819));
#53767=CARTESIAN_POINT('Ctrl Pts',(18.2940015296655,71.8680505476001,14.7204308714458));
#53768=CARTESIAN_POINT('Ctrl Pts',(18.2956059643778,71.8524446118942,14.7231094321163));
#53769=CARTESIAN_POINT('Ctrl Pts',(18.2984679648359,71.8242476018861,14.7274078639219));
#53770=CARTESIAN_POINT('Ctrl Pts',(18.2997304293162,71.8116764043031,14.7291319181347));
#53771=CARTESIAN_POINT('Ctrl Pts',(18.3024284729266,71.7845587862325,14.732437653291));
#53772=CARTESIAN_POINT('Ctrl Pts',(18.3038608346063,71.7700070826735,14.7339569356805));
#53773=CARTESIAN_POINT('Ctrl Pts',(18.3088224453373,71.7191640227705,14.7383785444306));
#53774=CARTESIAN_POINT('Ctrl Pts',(18.3122976264266,71.6827740069663,14.7399720473119));
#53775=CARTESIAN_POINT('Ctrl Pts',(18.3157454956419,71.6463622425315,14.7399996354682));
#53776=CARTESIAN_POINT('Ctrl Pts',(18.315745359276,71.6463636826444,14.7399996343762));
#53777=CARTESIAN_POINT('Ctrl Pts',(18.3256839003294,71.541406182485,14.7400792766994));
#53778=CARTESIAN_POINT('Ctrl Pts',(18.3353753375936,71.4368445038087,14.7271484664875));
#53779=CARTESIAN_POINT('Ctrl Pts',(18.3483273621578,71.3062132498836,14.6942293176145));
#53780=CARTESIAN_POINT('Ctrl Pts',(18.3512125677473,71.277632162101,14.6859488335247));
#53781=CARTESIAN_POINT('Ctrl Pts',(18.3564123717177,71.2272539108023,14.6694147261593));
#53782=CARTESIAN_POINT('Ctrl Pts',(18.3587135400297,71.205342846555,14.6615499832992));
#53783=CARTESIAN_POINT('Ctrl Pts',(18.3638991894459,71.1569055621928,14.6426457841576));
#53784=CARTESIAN_POINT('Ctrl Pts',(18.3667926908487,71.1305140061665,14.631299715972));
#53785=CARTESIAN_POINT('Ctrl Pts',(18.3759692296684,71.048922686953,14.5928946473237));
#53786=CARTESIAN_POINT('Ctrl Pts',(18.3823478497847,70.9952965746847,14.5627216455913));
#53787=CARTESIAN_POINT('Ctrl Pts',(18.3962593650635,70.8846926906335,14.4894594073753));
#53788=CARTESIAN_POINT('Ctrl Pts',(18.4037927950747,70.8287247474877,14.4452001769306));
#53789=CARTESIAN_POINT('Ctrl Pts',(18.4137450020772,70.7586899775641,14.3795377666154));
#53790=CARTESIAN_POINT('Ctrl Pts',(18.4162919818968,70.7411165966014,14.3620680524911));
#53791=CARTESIAN_POINT('Ctrl Pts',(18.4202240500033,70.7144463945094,14.3339563872702));
#53792=CARTESIAN_POINT('Ctrl Pts',(18.4216312040912,70.7049959745739,14.3236601302597));
#53793=CARTESIAN_POINT('Ctrl Pts',(18.4235989564324,70.6919012103889,14.3089118394509));
#53794=CARTESIAN_POINT('Ctrl Pts',(18.4241701294657,70.6881153666811,14.3045892094999));
#53795=CARTESIAN_POINT('Ctrl Pts',(18.4247393426037,70.684358943376,14.3002409815728));
#53796=CARTESIAN_POINT('',(18.4858211068938,71.645349016461,14.7399996799991));
#53797=CARTESIAN_POINT('Ctrl Pts',(18.5941331801233,70.6843589436049,14.3002409818378));
#53798=CARTESIAN_POINT('Ctrl Pts',(18.5907865350394,70.7057988947686,14.325058683886));
#53799=CARTESIAN_POINT('Ctrl Pts',(18.5874054687168,70.7281902732238,14.3490344495593));
#53800=CARTESIAN_POINT('Ctrl Pts',(18.5752698875643,70.8111251467179,14.4312156822484));
#53801=CARTESIAN_POINT('Ctrl Pts',(18.5663754828149,70.8764809986208,14.4842544402918));
#53802=CARTESIAN_POINT('Ctrl Pts',(18.5542369849415,70.9736114432448,14.5482614950515));
#53803=CARTESIAN_POINT('Ctrl Pts',(18.5508856285351,71.0013135803539,14.5650346634462));
#53804=CARTESIAN_POINT('Ctrl Pts',(18.5460485511096,71.0428260070941,14.5880484093272));
#53805=CARTESIAN_POINT('Ctrl Pts',(18.5445225702095,71.0561527869441,14.5951290877217));
#53806=CARTESIAN_POINT('Ctrl Pts',(18.541564339877,71.0824784619157,14.6085200871453));
#53807=CARTESIAN_POINT('Ctrl Pts',(18.5401313501845,71.0954648260161,14.6148493387851));
#53808=CARTESIAN_POINT('Ctrl Pts',(18.5359594460948,71.1338877916252,14.632771039288));
#53809=CARTESIAN_POINT('Ctrl Pts',(18.5332529837572,71.1596046085438,14.6437480355549));
#53810=CARTESIAN_POINT('Ctrl Pts',(18.5239302444666,71.2502775061027,14.6789592311908));
#53811=CARTESIAN_POINT('Ctrl Pts',(18.5174647761561,71.3168410088035,14.6987209114874));
#53812=CARTESIAN_POINT('Ctrl Pts',(18.5055123950072,71.441276410779,14.7248212602656));
#53813=CARTESIAN_POINT('Ctrl Pts',(18.500056217803,71.4986000308892,14.7328108636789));
#53814=CARTESIAN_POINT('Ctrl Pts',(18.4928819979801,71.5729290381079,14.7380406471959));
#53815=CARTESIAN_POINT('Ctrl Pts',(18.4912653341044,71.5896154585899,14.7388842152709));
#53816=CARTESIAN_POINT('Ctrl Pts',(18.4883724085359,71.619321579511,14.7397989225822));
#53817=CARTESIAN_POINT('Ctrl Pts',(18.487100038195,71.6323350556675,14.7399994731758));
#53818=CARTESIAN_POINT('Ctrl Pts',(18.4858216933514,71.6453486884009,14.7399999989634));
#53819=CARTESIAN_POINT('Ctrl Pts',(18.4858216558298,71.6453490703727,14.7399999989788));
#53820=CARTESIAN_POINT('Ctrl Pts',(18.4840637483041,71.663244680427,14.7400007166298));
#53821=CARTESIAN_POINT('Ctrl Pts',(18.482294843087,71.6811373155185,14.7396231841365));
#53822=CARTESIAN_POINT('Ctrl Pts',(18.4782654825454,71.7215925780454,14.7379137763227));
#53823=CARTESIAN_POINT('Ctrl Pts',(18.4759987726767,71.7441386739734,14.7363574390113));
#53824=CARTESIAN_POINT('Ctrl Pts',(18.4685594670071,71.8173651474842,14.7293354453857));
#53825=CARTESIAN_POINT('Ctrl Pts',(18.4633167768759,71.8677532169577,14.7214212683486));
#53826=CARTESIAN_POINT('Ctrl Pts',(18.4493532739256,71.9987014908871,14.692695895691));
#53827=CARTESIAN_POINT('Ctrl Pts',(18.4405463690157,72.0779316151334,14.6669639165977));
#53828=CARTESIAN_POINT('Ctrl Pts',(18.4296568718692,72.173736900525,14.6250846032055));
#53829=CARTESIAN_POINT('Ctrl Pts',(18.4274352410209,72.1931764897535,14.6159936230427));
#53830=CARTESIAN_POINT('Ctrl Pts',(18.4234138708816,72.2282528479709,14.5984933783508));
#53831=CARTESIAN_POINT('Ctrl Pts',(18.421608118556,72.2439616693562,14.5902405072629));
#53832=CARTESIAN_POINT('Ctrl Pts',(18.4184632784958,72.2712960892057,14.575140663398));
#53833=CARTESIAN_POINT('Ctrl Pts',(18.4171171918754,72.2829933447736,14.5684336907788));
#53834=CARTESIAN_POINT('Ctrl Pts',(18.4137399941561,72.3123084618777,14.5509988008193));
#53835=CARTESIAN_POINT('Ctrl Pts',(18.4117234080901,72.3297758978712,14.5400257527683));
#53836=CARTESIAN_POINT('Ctrl Pts',(18.400137615384,72.4294773205739,14.4739521750378));
#53837=CARTESIAN_POINT('Ctrl Pts',(18.390999655118,72.5053213920228,14.4098075870873));
#53838=CARTESIAN_POINT('Ctrl Pts',(18.3782410293835,72.5976497144407,14.3110872684802));
#53839=CARTESIAN_POINT('Ctrl Pts',(18.3748093649996,72.6212061965352,14.2836394715801));
#53840=CARTESIAN_POINT('Ctrl Pts',(18.3683925426735,72.6625300246403,14.2311097483416));
#53841=CARTESIAN_POINT('Ctrl Pts',(18.3654206773575,72.6806197171338,14.2063160472623));
#53842=CARTESIAN_POINT('Ctrl Pts',(18.3601313085065,72.7108408312795,14.1615773475406));
#53843=CARTESIAN_POINT('Ctrl Pts',(18.3578291968888,72.7233538303298,14.1419068059499));
#53844=CARTESIAN_POINT('Ctrl Pts',(18.3527196402942,72.7496784222156,14.0978947959057));
#53845=CARTESIAN_POINT('Ctrl Pts',(18.3499047110374,72.7632404814613,14.0734194702424));
#53846=CARTESIAN_POINT('Ctrl Pts',(18.3379039477335,72.8170377356596,13.9682850700007));
#53847=CARTESIAN_POINT('Ctrl Pts',(18.3284682238935,72.8494271547613,13.8839259139512));
#53848=CARTESIAN_POINT('Ctrl Pts',(18.3146944114495,72.8831294672406,13.7573932734595));
#53849=CARTESIAN_POINT('Ctrl Pts',(18.3104007072289,72.8917342225672,13.7174278508353));
#53850=CARTESIAN_POINT('Ctrl Pts',(18.3033353405523,72.9028224282651,13.6503467473071));
#53851=CARTESIAN_POINT('Ctrl Pts',(18.3005388771244,72.9063886847045,13.6234405012951));
#53852=CARTESIAN_POINT('Ctrl Pts',(18.2963252051142,72.9105162175549,13.5821875876307));
#53853=CARTESIAN_POINT('Ctrl Pts',(18.2948806267495,72.9117010161109,13.5679128447337));
#53854=CARTESIAN_POINT('Ctrl Pts',(18.2919249402125,72.9136486908722,13.5383960599083));
#53855=CARTESIAN_POINT('Ctrl Pts',(18.2904155684304,72.9143789032385,13.5231543835663));
#53856=CARTESIAN_POINT('Ctrl Pts',(18.2856188727244,72.9158379960445,13.4742855406007));
#53857=CARTESIAN_POINT('Ctrl Pts',(18.2823808775923,72.9155061169949,13.4406379507612));
#53858=CARTESIAN_POINT('Ctrl Pts',(18.2713021763805,72.9097426413883,13.3245247909113));
#53859=CARTESIAN_POINT('Ctrl Pts',(18.2636411054131,72.8976051508321,13.2426034582882));
#53860=CARTESIAN_POINT('Ctrl Pts',(18.2525956884939,72.8693120586383,13.1292520282826));
#53861=CARTESIAN_POINT('Ctrl Pts',(18.2493427518675,72.8596921526603,13.0964171786878));
#53862=CARTESIAN_POINT('Ctrl Pts',(18.2432068567256,72.8392949932667,13.0359592994719));
#53863=CARTESIAN_POINT('Ctrl Pts',(18.2403349265164,72.8288531504033,13.0082480057006));
#53864=CARTESIAN_POINT('Ctrl Pts',(18.2351490465228,72.8084924619636,12.9594537998925));
#53865=CARTESIAN_POINT('Ctrl Pts',(18.2328482340944,72.7989434883822,12.9382305558151));
#53866=CARTESIAN_POINT('Ctrl Pts',(18.227651005068,72.7762674632518,12.8913201476615));
#53867=CARTESIAN_POINT('Ctrl Pts',(18.2247453235574,72.7628378825125,12.8657948759892));
#53868=CARTESIAN_POINT('Ctrl Pts',(18.2154060802847,72.7173748613197,12.7860924546668));
#53869=CARTESIAN_POINT('Ctrl Pts',(18.2088712336361,72.6821835065995,12.7338363463221));
#53870=CARTESIAN_POINT('Ctrl Pts',(18.1948834508981,72.5997055018529,12.6290710077774));
#53871=CARTESIAN_POINT('Ctrl Pts',(18.18743600577,72.5516091393923,12.5774494804156));
#53872=CARTESIAN_POINT('Ctrl Pts',(18.1776332414141,72.48157927186,12.513815310477));
#53873=CARTESIAN_POINT('Ctrl Pts',(18.175148119483,72.4632167987984,12.4980633382184));
#53874=CARTESIAN_POINT('Ctrl Pts',(18.1712858161642,72.4336181126922,12.4741058777211));
#53875=CARTESIAN_POINT('Ctrl Pts',(18.1698878469869,72.4226788513101,12.4655446364968));
#53876=CARTESIAN_POINT('Ctrl Pts',(18.1669020070733,72.3988019514851,12.4474820225952));
#53877=CARTESIAN_POINT('Ctrl Pts',(18.165318002951,72.3858206037548,12.4380431512228));
#53878=CARTESIAN_POINT('Ctrl Pts',(18.1603550848147,72.344249433831,12.409004858421));
#53879=CARTESIAN_POINT('Ctrl Pts',(18.1570265323417,72.3150318396945,12.3903264116734));
#53880=CARTESIAN_POINT('Ctrl Pts',(18.146104194103,72.2158189557635,12.3324805174102));
#53881=CARTESIAN_POINT('Ctrl Pts',(18.1386639308201,72.1428842690816,12.2987447173984));
#53882=CARTESIAN_POINT('Ctrl Pts',(18.1278786644537,72.0353180146071,12.2608638434066));
#53883=CARTESIAN_POINT('Ctrl Pts',(18.1246574767609,72.0029489804888,12.2509000510684));
#53884=CARTESIAN_POINT('Ctrl Pts',(18.118571720353,71.9417882292341,12.2347190024447));
#53885=CARTESIAN_POINT('Ctrl Pts',(18.1157177937111,71.9131035623116,12.228186965682));
#53886=CARTESIAN_POINT('Ctrl Pts',(18.1105500675895,71.8613682897272,12.218281554135));
#53887=CARTESIAN_POINT('Ctrl Pts',(18.1082489994013,71.8384020656323,12.2145353862735));
#53888=CARTESIAN_POINT('Ctrl Pts',(18.1030329315977,71.7865915689535,12.2075393332325));
#53889=CARTESIAN_POINT('Ctrl Pts',(18.1001082989963,71.7577139120084,12.2046434354114));
#53890=CARTESIAN_POINT('Ctrl Pts',(18.0892228955812,71.6510312151929,12.1976254395082));
#53891=CARTESIAN_POINT('Ctrl Pts',(18.081089827151,71.5730068168395,12.1996758944694));
#53892=CARTESIAN_POINT('Ctrl Pts',(18.0679879977557,71.4492918110199,12.2143632947521));
#53893=CARTESIAN_POINT('Ctrl Pts',(18.063068441033,71.4032431413625,12.2224253826389));
#53894=CARTESIAN_POINT('Ctrl Pts',(18.0551504022456,71.3291696951112,12.2396509097847));
#53895=CARTESIAN_POINT('Ctrl Pts',(18.0521207649156,71.3008332617348,12.2472839005731));
#53896=CARTESIAN_POINT('Ctrl Pts',(18.0476438491228,71.2587755976031,12.2601916368784));
#53897=CARTESIAN_POINT('Ctrl Pts',(18.0461639997273,71.2448418263868,12.264733252419));
#53898=CARTESIAN_POINT('Ctrl Pts',(18.0432128237681,71.2169541504291,12.2743601758368));
#53899=CARTESIAN_POINT('Ctrl Pts',(18.0417420297667,71.2030045791085,12.2794510493998));
#53900=CARTESIAN_POINT('Ctrl Pts',(18.0372718794751,71.1605440245763,12.2957964376332));
#53901=CARTESIAN_POINT('Ctrl Pts',(18.0343126249969,71.1323459557959,12.3078402197336));
#53902=CARTESIAN_POINT('Ctrl Pts',(18.0231809422392,71.0269505745896,12.3574413891282));
#53903=CARTESIAN_POINT('Ctrl Pts',(18.0152293408142,70.9531931053143,12.4017686786448));
#53904=CARTESIAN_POINT('Ctrl Pts',(18.0038434143002,70.8567358864697,12.4739535123158));
#53905=CARTESIAN_POINT('Ctrl Pts',(18.0005508794765,70.8298677176999,12.4958303912643));
#53906=CARTESIAN_POINT('Ctrl Pts',(17.9943525436072,70.7815728334608,12.5385529841837));
#53907=CARTESIAN_POINT('Ctrl Pts',(17.991458259386,70.7599230154431,12.5591097218628));
#53908=CARTESIAN_POINT('Ctrl Pts',(17.9862496160912,70.7227154160695,12.5970195234435));
#53909=CARTESIAN_POINT('Ctrl Pts',(17.9839488984312,70.7068727845143,12.6140746273569));
#53910=CARTESIAN_POINT('Ctrl Pts',(17.9787736591296,70.6726104877898,12.6530544785039));
#53911=CARTESIAN_POINT('Ctrl Pts',(17.9758903074491,70.6544464551056,12.6751854547461));
#53912=CARTESIAN_POINT('Ctrl Pts',(17.9644907802717,70.5863305040555,12.7641450488083));
#53913=CARTESIAN_POINT('Ctrl Pts',(17.9557694668081,70.5422737533617,12.8352037232949));
#53914=CARTESIAN_POINT('Ctrl Pts',(17.9423837241819,70.4861668115996,12.9494209986068));
#53915=CARTESIAN_POINT('Ctrl Pts',(17.9377683655224,70.4688784489235,12.9897692841891));
#53916=CARTESIAN_POINT('Ctrl Pts',(17.9302615078548,70.4439298467833,13.057483261148));
#53917=CARTESIAN_POINT('Ctrl Pts',(17.9273419383479,70.4350365886228,13.0843558957413));
#53918=CARTESIAN_POINT('Ctrl Pts',(17.9229891842093,70.4229556585547,13.1254133142619));
#53919=CARTESIAN_POINT('Ctrl Pts',(17.921525915318,70.4191015775667,13.1393908411115));
#53920=CARTESIAN_POINT('Ctrl Pts',(17.9185739965236,70.4117420356213,13.167983794663));
#53921=CARTESIAN_POINT('Ctrl Pts',(17.9170864147555,70.4082549276517,13.1826014775612));
#53922=CARTESIAN_POINT('Ctrl Pts',(17.9125896385425,70.3984202553461,13.2273308864539));
#53923=CARTESIAN_POINT('Ctrl Pts',(17.9096203858763,70.3929061963926,13.2576169988945));
#53924=CARTESIAN_POINT('Ctrl Pts',(17.8998223083347,70.3782124163215,13.3591362158437));
#53925=CARTESIAN_POINT('Ctrl Pts',(17.8931374565105,70.3739710988272,13.4309446410726));
#53926=CARTESIAN_POINT('Ctrl Pts',(17.8825602727117,70.3768668947881,13.5432659352113));
#53927=CARTESIAN_POINT('Ctrl Pts',(17.8787269955245,70.3798524706749,13.5837238676785));
#53928=CARTESIAN_POINT('Ctrl Pts',(17.8716882588164,70.3887678897535,13.6567204655158));
#53929=CARTESIAN_POINT('Ctrl Pts',(17.8685017504575,70.3940427608706,13.6893021430525));
#53930=CARTESIAN_POINT('Ctrl Pts',(17.8629796112522,70.4052347088154,13.7446671426077));
#53931=CARTESIAN_POINT('Ctrl Pts',(17.8606643023507,70.4105276398742,13.7675601851188));
#53932=CARTESIAN_POINT('Ctrl Pts',(17.8556767514497,70.423178391136,13.8161007073866));
#53933=CARTESIAN_POINT('Ctrl Pts',(17.8529998485143,70.4307155321467,13.8416890302233));
#53934=CARTESIAN_POINT('Ctrl Pts',(17.8440140117216,70.4584369427401,13.9259209911582));
#53935=CARTESIAN_POINT('Ctrl Pts',(17.8376003499489,70.4821062392049,13.9833128969222));
#53936=CARTESIAN_POINT('Ctrl Pts',(17.824552203637,70.5379202404912,14.0947503930631));
#53937=CARTESIAN_POINT('Ctrl Pts',(17.8179334451509,70.5700799455042,14.1486097409248));
#53938=CARTESIAN_POINT('Ctrl Pts',(17.8088461515945,70.6200693884098,14.2197929446072));
#53939=CARTESIAN_POINT('Ctrl Pts',(17.8063171815365,70.6346271663127,14.2393053947095));
#53940=CARTESIAN_POINT('Ctrl Pts',(17.8019493230965,70.6609776077316,14.2725835627279));
#53941=CARTESIAN_POINT('Ctrl Pts',(17.8001000974776,70.6725205624489,14.2865375263508));
#53942=CARTESIAN_POINT('Ctrl Pts',(17.7982694921739,70.6843589433905,14.3002409815896));
#53943=CARTESIAN_POINT('Origin',(21.26284859951,71.6454,13.47));
#53944=CARTESIAN_POINT('',(16.8359541306755,70.6843588624425,14.3002408878887));
#53945=CARTESIAN_POINT('',(17.0063123822734,70.684359077848,14.3002411372302));
#53946=CARTESIAN_POINT('',(21.26284859951,70.6843589433668,14.3002409815622));
#53947=CARTESIAN_POINT('Ctrl Pts',(16.8359541306755,70.6843588624425,14.3002408878887));
#53948=CARTESIAN_POINT('Ctrl Pts',(16.8379502674075,70.6704802270336,14.2841757437171));
#53949=CARTESIAN_POINT('Ctrl Pts',(16.839950549689,70.6570003623999,14.2677579081367));
#53950=CARTESIAN_POINT('Ctrl Pts',(16.845164028052,70.6230991339372,14.224286865956));
#53951=CARTESIAN_POINT('Ctrl Pts',(16.8483871622081,70.6033442919936,14.1967511909312));
#53952=CARTESIAN_POINT('Ctrl Pts',(16.8544761522747,70.5685314353906,14.1438842720158));
#53953=CARTESIAN_POINT('Ctrl Pts',(16.8573313450209,70.553208424895,14.1187550882452));
#53954=CARTESIAN_POINT('Ctrl Pts',(16.86250082345,70.5273547155229,14.0728402269413));
#53955=CARTESIAN_POINT('Ctrl Pts',(16.8648023568894,70.5164968416139,14.0522534499787));
#53956=CARTESIAN_POINT('Ctrl Pts',(16.8700189304026,70.4933846757216,14.0053528887906));
#53957=CARTESIAN_POINT('Ctrl Pts',(16.8729435958922,70.4814551667086,13.9788949833143));
#53958=CARTESIAN_POINT('Ctrl Pts',(16.883833999383,70.440855195297,13.8799368366222));
#53959=CARTESIAN_POINT('Ctrl Pts',(16.8919723041514,70.4179755336285,13.8052624961549));
#53960=CARTESIAN_POINT('Ctrl Pts',(16.9050765319503,70.3925658381841,13.6832745343453));
#53961=CARTESIAN_POINT('Ctrl Pts',(16.9099932350481,70.3855727693127,13.6370785016066));
#53962=CARTESIAN_POINT('Ctrl Pts',(16.9179075539254,70.3783543322301,13.5614071749565));
#53963=CARTESIAN_POINT('Ctrl Pts',(16.9209362945866,70.3765811922217,13.5321227495037));
#53964=CARTESIAN_POINT('Ctrl Pts',(16.9254123744121,70.3754451816052,13.4881515204587));
#53965=CARTESIAN_POINT('Ctrl Pts',(16.9268922624674,70.3753202490823,13.4734963106848));
#53966=CARTESIAN_POINT('Ctrl Pts',(16.929844092251,70.37557953879,13.4439881082713));
#53967=CARTESIAN_POINT('Ctrl Pts',(16.9313154919548,70.375970619472,13.4291374594395));
#53968=CARTESIAN_POINT('Ctrl Pts',(16.9357893372522,70.3779679132012,13.3836449829257));
#53969=CARTESIAN_POINT('Ctrl Pts',(16.9387515883091,70.3804240206811,13.3530489802766));
#53970=CARTESIAN_POINT('Ctrl Pts',(16.9498826574407,70.3939460650015,13.2373555601887));
#53971=CARTESIAN_POINT('Ctrl Pts',(16.9578311141366,70.4125149637098,13.1533660574458));
#53972=CARTESIAN_POINT('Ctrl Pts',(16.9692135431134,70.4502697839419,13.0389973621562));
#53973=CARTESIAN_POINT('Ctrl Pts',(16.9725058433213,70.462466561564,13.0065697162679));
#53974=CARTESIAN_POINT('Ctrl Pts',(16.9787039585334,70.4876134337804,12.947198712339));
#53975=CARTESIAN_POINT('Ctrl Pts',(16.981598261852,70.5002188097435,12.92013580511));
#53976=CARTESIAN_POINT('Ctrl Pts',(16.9868073685666,70.5243313483591,12.8728006726035));
#53977=CARTESIAN_POINT('Ctrl Pts',(16.9891085369967,70.5354656490704,12.8523532411427));
#53978=CARTESIAN_POINT('Ctrl Pts',(16.9942854473045,70.5615359031707,12.8074604000989));
#53979=CARTESIAN_POINT('Ctrl Pts',(16.9971700354299,70.576749147576,12.7831920746164));
#53980=CARTESIAN_POINT('Ctrl Pts',(17.008560415326,70.6393835052347,12.6904020618607));
#53981=CARTESIAN_POINT('Ctrl Pts',(17.0172706903457,70.6926723967465,12.6261121605154));
#53982=CARTESIAN_POINT('Ctrl Pts',(17.0306508725578,70.7830640764349,12.5366162070676));
#53983=CARTESIAN_POINT('Ctrl Pts',(17.0352716721509,70.8158543917736,12.5073562171363));
#53984=CARTESIAN_POINT('Ctrl Pts',(17.0427860399314,70.8721718040111,12.4621210967851));
#53985=CARTESIAN_POINT('Ctrl Pts',(17.0457077329421,70.8948367125143,12.445130811959));
#53986=CARTESIAN_POINT('Ctrl Pts',(17.0500630526936,70.9299408716333,12.4206056392062));
#53987=CARTESIAN_POINT('Ctrl Pts',(17.0515268098408,70.9419709965363,12.4125038956092));
#53988=CARTESIAN_POINT('Ctrl Pts',(17.0544793513002,70.9667442439723,12.3964301761461));
#53989=CARTESIAN_POINT('Ctrl Pts',(17.0559670726542,70.979495279746,12.3884747877085));
#53990=CARTESIAN_POINT('Ctrl Pts',(17.0604637907267,71.0187745105876,12.3649266313307));
#53991=CARTESIAN_POINT('Ctrl Pts',(17.0634328534424,71.0457330009495,12.3500684711583));
#53992=CARTESIAN_POINT('Ctrl Pts',(17.0732315787877,71.1373148376821,12.3038499911104));
#53993=CARTESIAN_POINT('Ctrl Pts',(17.0799172088496,71.2040548050841,12.2769901861361));
#53994=CARTESIAN_POINT('Ctrl Pts',(17.0904951641001,71.3114743432413,12.2440155964545));
#53995=CARTESIAN_POINT('Ctrl Pts',(17.0943284069696,71.350781175896,12.233980832988));
#53996=CARTESIAN_POINT('Ctrl Pts',(17.1013672436168,71.422824624803,12.219220609583));
#53997=CARTESIAN_POINT('Ctrl Pts',(17.1045538890003,71.4553937696643,12.2138606404425));
#53998=CARTESIAN_POINT('Ctrl Pts',(17.1100765744997,71.511449267714,12.2068652560344));
#53999=CARTESIAN_POINT('Ctrl Pts',(17.1123922954551,71.5348411825001,12.2046033235569));
#54000=CARTESIAN_POINT('Ctrl Pts',(17.1173811510999,71.584897777677,12.2011614333445));
#54001=CARTESIAN_POINT('Ctrl Pts',(17.1200589558797,71.6115634051959,12.2001706246371));
#54002=CARTESIAN_POINT('Ctrl Pts',(17.1290858369526,71.7006423614078,12.199668268823));
#54003=CARTESIAN_POINT('Ctrl Pts',(17.1355413113164,71.7629756245786,12.2039164303789));
#54004=CARTESIAN_POINT('Ctrl Pts',(17.1486007471835,71.8864515560885,12.2215286294965));
#54005=CARTESIAN_POINT('Ctrl Pts',(17.1551872759319,71.9474367062982,12.2348642216444));
#54006=CARTESIAN_POINT('Ctrl Pts',(17.1642373003921,72.0304771966761,12.2595432882361));
#54007=CARTESIAN_POINT('Ctrl Pts',(17.1667609477631,72.05355725548,12.2671293746634));
#54008=CARTESIAN_POINT('Ctrl Pts',(17.1712504847815,72.0945997776521,12.2819370349647));
#54009=CARTESIAN_POINT('Ctrl Pts',(17.1732246725733,72.1126418150013,12.2889160560463));
#54010=CARTESIAN_POINT('Ctrl Pts',(17.1765321714097,72.1429248879647,12.3014328506582));
#54011=CARTESIAN_POINT('Ctrl Pts',(17.1778759447413,72.1552487368115,12.3067568927788));
#54012=CARTESIAN_POINT('Ctrl Pts',(17.1810706229633,72.1845901472999,12.3199887159938));
#54013=CARTESIAN_POINT('Ctrl Pts',(17.1829112245127,72.2015210873649,12.3280799311336));
#54014=CARTESIAN_POINT('Ctrl Pts',(17.1907897820885,72.2738470390506,12.36463471619));
#54015=CARTESIAN_POINT('Ctrl Pts',(17.1966549018235,72.3272936975534,12.3967798227777));
#54016=CARTESIAN_POINT('Ctrl Pts',(17.2098037094555,72.4415776912482,12.4775144449506));
#54017=CARTESIAN_POINT('Ctrl Pts',(17.2170589253695,72.5007355077009,12.5280202908593));
#54018=CARTESIAN_POINT('Ctrl Pts',(17.2274260378182,72.5760580239803,12.6053070860478));
#54019=CARTESIAN_POINT('Ctrl Pts',(17.2303624003649,72.5964214923708,12.6277553958142));
#54020=CARTESIAN_POINT('Ctrl Pts',(17.2356149248811,72.630985811239,12.6687114724665));
#54021=CARTESIAN_POINT('Ctrl Pts',(17.2379165027369,72.6455165714169,12.6869231436508));
#54022=CARTESIAN_POINT('Ctrl Pts',(17.2430557330966,72.6765538054759,12.7280963887751));
#54023=CARTESIAN_POINT('Ctrl Pts',(17.2459014712567,72.6928101230684,12.7512296235364));
#54024=CARTESIAN_POINT('Ctrl Pts',(17.2576524165042,72.7560685944708,12.8479560830587));
#54025=CARTESIAN_POINT('Ctrl Pts',(17.26678806957,72.7961846969771,12.9257467497746));
#54026=CARTESIAN_POINT('Ctrl Pts',(17.2803943905939,72.8433386395253,13.0461922455354));
#54027=CARTESIAN_POINT('Ctrl Pts',(17.2848181234015,72.8567206689711,13.0861085465591));
#54028=CARTESIAN_POINT('Ctrl Pts',(17.2920629203467,72.8755626411892,13.1532000122908));
#54029=CARTESIAN_POINT('Ctrl Pts',(17.2949101057792,72.8821600598556,13.1800219613069));
#54030=CARTESIAN_POINT('Ctrl Pts',(17.2991812538307,72.890858887507,13.2211237710634));
#54031=CARTESIAN_POINT('Ctrl Pts',(17.3006336956985,72.8936001077483,13.2352580206003));
#54032=CARTESIAN_POINT('Ctrl Pts',(17.3035880319527,72.8987337964409,13.2643686046479));
#54033=CARTESIAN_POINT('Ctrl Pts',(17.305088469304,72.9010995836649,13.2793471405344));
#54034=CARTESIAN_POINT('Ctrl Pts',(17.3098053885583,72.9077462890829,13.3269472257574));
#54035=CARTESIAN_POINT('Ctrl Pts',(17.3129748929082,72.9110287781448,13.3596975801237));
#54036=CARTESIAN_POINT('Ctrl Pts',(17.3240643116881,72.9181214440081,13.4757733198151));
#54037=CARTESIAN_POINT('Ctrl Pts',(17.3317950769148,72.9149980632514,13.559306641125));
#54038=CARTESIAN_POINT('Ctrl Pts',(17.3429225431855,72.8990624982484,13.6759312020774));
#54039=CARTESIAN_POINT('Ctrl Pts',(17.3461853877226,72.8930418323433,13.7097223903609));
#54040=CARTESIAN_POINT('Ctrl Pts',(17.3523370701615,72.8792781125012,13.7722003649012));
#54041=CARTESIAN_POINT('Ctrl Pts',(17.3552147605128,72.8718824100622,13.8009393175549));
#54042=CARTESIAN_POINT('Ctrl Pts',(17.3604069398278,72.8569013444631,13.8517148885454));
#54043=CARTESIAN_POINT('Ctrl Pts',(17.3627081686528,72.8497027366733,13.8738520842561));
#54044=CARTESIAN_POINT('Ctrl Pts',(17.3679013402921,72.8322471485367,13.9229050109656));
#54045=CARTESIAN_POINT('Ctrl Pts',(17.370802451131,72.8216749507958,13.9496936592688));
#54046=CARTESIAN_POINT('Ctrl Pts',(17.3800770330949,72.7853596538845,14.0332747275669));
#54047=CARTESIAN_POINT('Ctrl Pts',(17.3865494879895,72.7563447683254,14.0885349994856));
#54048=CARTESIAN_POINT('Ctrl Pts',(17.4005066698503,72.6859939171446,14.2014843657338));
#54049=CARTESIAN_POINT('Ctrl Pts',(17.4079882576799,72.6436376248547,14.2583067620268));
#54050=CARTESIAN_POINT('Ctrl Pts',(17.4178503181667,72.580592356801,14.3295996075902));
#54051=CARTESIAN_POINT('Ctrl Pts',(17.4203599717543,72.5638908540786,14.3474229552307));
#54052=CARTESIAN_POINT('Ctrl Pts',(17.4242500419274,72.5368745890423,14.3746363432778));
#54053=CARTESIAN_POINT('Ctrl Pts',(17.4256517500158,72.526902363284,14.3843563497114));
#54054=CARTESIAN_POINT('Ctrl Pts',(17.4286345206178,72.5051477424299,14.4048738343657));
#54055=CARTESIAN_POINT('Ctrl Pts',(17.4302119054587,72.4933177095941,14.415616686145));
#54056=CARTESIAN_POINT('Ctrl Pts',(17.43544837966,72.4530451967044,14.4508243635592));
#54057=CARTESIAN_POINT('Ctrl Pts',(17.4390458233716,72.4237192820745,14.4742544900942));
#54058=CARTESIAN_POINT('Ctrl Pts',(17.4500385044826,72.3301687276508,14.5424330059884));
#54059=CARTESIAN_POINT('Ctrl Pts',(17.4573028450546,72.2628186307826,14.5825717474207));
#54060=CARTESIAN_POINT('Ctrl Pts',(17.4678801303163,72.1619009041245,14.6307126383981));
#54061=CARTESIAN_POINT('Ctrl Pts',(17.4710751384315,72.1310421460964,14.6439584234647));
#54062=CARTESIAN_POINT('Ctrl Pts',(17.4771196613344,72.0723790579472,14.6664299692564));
#54063=CARTESIAN_POINT('Ctrl Pts',(17.4799588515385,72.044710173669,14.6759464585642));
#54064=CARTESIAN_POINT('Ctrl Pts',(17.4851123503572,71.9944855997353,14.691302909296));
#54065=CARTESIAN_POINT('Ctrl Pts',(17.4874142683972,71.9720504218978,14.6974937383329));
#54066=CARTESIAN_POINT('Ctrl Pts',(17.4926485278792,71.9211233612057,14.7100517715196));
#54067=CARTESIAN_POINT('Ctrl Pts',(17.4955908365224,71.8925577576327,14.7160595736707));
#54068=CARTESIAN_POINT('Ctrl Pts',(17.5060571430106,71.7913219326228,14.733733346607));
#54069=CARTESIAN_POINT('Ctrl Pts',(17.5137303089856,71.7178815674439,14.7400620565365));
#54070=CARTESIAN_POINT('Ctrl Pts',(17.5287987453517,71.5745430262868,14.739940241369));
#54071=CARTESIAN_POINT('Ctrl Pts',(17.5361615722082,71.5048822405677,14.7341303825615));
#54072=CARTESIAN_POINT('Ctrl Pts',(17.545050853754,71.4195441546375,14.7198676074413));
#54073=CARTESIAN_POINT('Ctrl Pts',(17.546757456842,71.403097516912,14.716783662814));
#54074=CARTESIAN_POINT('Ctrl Pts',(17.5498071241747,71.3735452815013,14.7106353082214));
#54075=CARTESIAN_POINT('Ctrl Pts',(17.5511552126588,71.3604192363079,14.7076861446184));
#54076=CARTESIAN_POINT('Ctrl Pts',(17.5542920712509,71.329727142343,14.7002759672918));
#54077=CARTESIAN_POINT('Ctrl Pts',(17.5560720033473,71.3122052388149,14.6956466404526));
#54078=CARTESIAN_POINT('Ctrl Pts',(17.5636398789525,71.2374923738237,14.6741863840508));
#54079=CARTESIAN_POINT('Ctrl Pts',(17.5692665344334,71.1814181620463,14.6537130723811));
#54080=CARTESIAN_POINT('Ctrl Pts',(17.5830649599599,71.0474544455944,14.5938106406161));
#54081=CARTESIAN_POINT('Ctrl Pts',(17.5911891660671,70.9718063104397,14.5501658537986));
#54082=CARTESIAN_POINT('Ctrl Pts',(17.6023102316911,70.8783030703642,14.4825524270219));
#54083=CARTESIAN_POINT('Ctrl Pts',(17.6050598076266,70.8559439559007,14.4652180592734));
#54084=CARTESIAN_POINT('Ctrl Pts',(17.6101050040048,70.8164321065771,14.4324159961435));
#54085=CARTESIAN_POINT('Ctrl Pts',(17.6123899221667,70.7990866290489,14.4171989355864));
#54086=CARTESIAN_POINT('Ctrl Pts',(17.6177045644565,70.7600656457738,14.3810384135039));
#54087=CARTESIAN_POINT('Ctrl Pts',(17.6207465576715,70.7387031385107,14.3597799322167));
#54088=CARTESIAN_POINT('Ctrl Pts',(17.6255371798314,70.7066136276283,14.3254903017749));
#54089=CARTESIAN_POINT('Ctrl Pts',(17.6272633913326,70.6953582812584,14.3129732092515));
#54090=CARTESIAN_POINT('Ctrl Pts',(17.6289974407812,70.6843588693663,14.3002408959033));
#54091=CARTESIAN_POINT('Ctrl Pts',(17.7982694921739,70.6843589433905,14.3002409815896));
#54092=CARTESIAN_POINT('Ctrl Pts',(17.798141983499,70.6851835319912,14.3011954797627));
#54093=CARTESIAN_POINT('Ctrl Pts',(17.7980145652821,70.6860095539031,14.3021487625671));
#54094=CARTESIAN_POINT('Ctrl Pts',(17.7965324570601,70.6956413124015,14.3132310313189));
#54095=CARTESIAN_POINT('Ctrl Pts',(17.7951888424883,70.7046057250814,14.3232211516946));
#54096=CARTESIAN_POINT('Ctrl Pts',(17.7919976091691,70.7264548485502,14.3468069948779));
#54097=CARTESIAN_POINT('Ctrl Pts',(17.7901602215311,70.739484893446,14.3602632509054));
#54098=CARTESIAN_POINT('Ctrl Pts',(17.7819760592256,70.7993647803753,14.4194248688467));
#54099=CARTESIAN_POINT('Ctrl Pts',(17.7758222886051,70.8494141499656,14.4617623107905));
#54100=CARTESIAN_POINT('Ctrl Pts',(17.7644724956504,70.9474075010228,14.5324360714136));
#54101=CARTESIAN_POINT('Ctrl Pts',(17.75928803274,70.9943686310677,14.5618431805322));
#54102=CARTESIAN_POINT('Ctrl Pts',(17.7522416694991,71.0596171213908,14.5969918223241));
#54103=CARTESIAN_POINT('Ctrl Pts',(17.7504498254515,71.0763325757062,14.6055238222977));
#54104=CARTESIAN_POINT('Ctrl Pts',(17.745723218479,71.1206518772488,14.6269211874799));
#54105=CARTESIAN_POINT('Ctrl Pts',(17.742773076104,71.1485381055385,14.6391685674617));
#54106=CARTESIAN_POINT('Ctrl Pts',(17.7375066056104,71.198489415022,14.6589969442097));
#54107=CARTESIAN_POINT('Ctrl Pts',(17.7352051797044,71.2203744606912,14.6669945359056));
#54108=CARTESIAN_POINT('Ctrl Pts',(17.7300789351109,71.2691560696397,14.6833147313981));
#54109=CARTESIAN_POINT('Ctrl Pts',(17.7272462799696,71.2961334417485,14.6913536297841));
#54110=CARTESIAN_POINT('Ctrl Pts',(17.7133070449797,71.4287812536618,14.7261271037611));
#54111=CARTESIAN_POINT('Ctrl Pts',(17.7018121006364,71.5373093967425,14.740072679018));
#54112=CARTESIAN_POINT('Ctrl Pts',(17.6859997248145,71.6880673818012,14.7399717082816));
#54113=CARTESIAN_POINT('Ctrl Pts',(17.6816401613189,71.729862731941,14.7378783747104));
#54114=CARTESIAN_POINT('Ctrl Pts',(17.6756593004317,71.7880195507758,14.7320759996778));
#54115=CARTESIAN_POINT('Ctrl Pts',(17.673971865577,71.8045232333242,14.7301016081262));
#54116=CARTESIAN_POINT('Ctrl Pts',(17.670924941542,71.8345475793578,14.7259103172365));
#54117=CARTESIAN_POINT('Ctrl Pts',(17.669561000977,71.8480780531925,14.7237979005548));
#54118=CARTESIAN_POINT('Ctrl Pts',(17.6659654593287,71.8839391742023,14.7176033821732));
#54119=CARTESIAN_POINT('Ctrl Pts',(17.6637531621711,71.9061994763753,14.7131407789932));
#54120=CARTESIAN_POINT('Ctrl Pts',(17.6585907781158,71.9583372227301,14.7012261023741));
#54121=CARTESIAN_POINT('Ctrl Pts',(17.6556600673009,71.9880874774465,14.6932796331891));
#54122=CARTESIAN_POINT('Ctrl Pts',(17.6444306207584,72.101582752939,14.6584978452878));
#54123=CARTESIAN_POINT('Ctrl Pts',(17.6362799460414,72.1827384372069,14.6240784404604));
#54124=CARTESIAN_POINT('Ctrl Pts',(17.6244143563793,72.2916626430337,14.5638826345195));
#54125=CARTESIAN_POINT('Ctrl Pts',(17.6208997167792,72.32285636335,14.5448427571435));
#54126=CARTESIAN_POINT('Ctrl Pts',(17.6150303068731,72.3728327829704,14.5112980357386));
#54127=CARTESIAN_POINT('Ctrl Pts',(17.6127042130437,72.3921081442529,14.497563535446));
#54128=CARTESIAN_POINT('Ctrl Pts',(17.6078383874262,72.4312534810866,14.467987719911));
#54129=CARTESIAN_POINT('Ctrl Pts',(17.6052966199824,72.4510539678347,14.4520726214928));
#54130=CARTESIAN_POINT('Ctrl Pts',(17.5978271729298,72.5072813189877,14.4040334777152));
#54131=CARTESIAN_POINT('Ctrl Pts',(17.5928421707213,72.5423547401596,14.3704047414771));
#54132=CARTESIAN_POINT('Ctrl Pts',(17.5789078217696,72.6336292891831,14.2722537912588));
#54133=CARTESIAN_POINT('Ctrl Pts',(17.5698486539841,72.68537154262,14.2039386287823));
#54134=CARTESIAN_POINT('Ctrl Pts',(17.557709771735,72.7459720791204,14.1045075597123));
#54135=CARTESIAN_POINT('Ctrl Pts',(17.5545074457054,72.761116175044,14.0774838469117));
#54136=CARTESIAN_POINT('Ctrl Pts',(17.5498365061385,72.7820591896073,14.0366812778136));
#54137=CARTESIAN_POINT('Ctrl Pts',(17.5483312785713,72.7886266611957,14.0233124453545));
#54138=CARTESIAN_POINT('Ctrl Pts',(17.5453776050037,72.801168773399,13.9966042514787));
#54139=CARTESIAN_POINT('Ctrl Pts',(17.5439289695145,72.807151347179,13.9832712435363));
#54140=CARTESIAN_POINT('Ctrl Pts',(17.5396346667906,72.8243386559848,13.9431256818056));
#54141=CARTESIAN_POINT('Ctrl Pts',(17.53682451205,72.8348557878354,13.9160264765483));
#54142=CARTESIAN_POINT('Ctrl Pts',(17.5296454289577,72.8595745239038,13.8452200890158));
#54143=CARTESIAN_POINT('Ctrl Pts',(17.5253235621992,72.872351471927,13.8010599695277));
#54144=CARTESIAN_POINT('Ctrl Pts',(17.5135547910652,72.9005905795693,13.679018946995));
#54145=CARTESIAN_POINT('Ctrl Pts',(17.5061364901567,72.9111912264958,13.6002407992517));
#54146=CARTESIAN_POINT('Ctrl Pts',(17.4957159300682,72.9155375001407,13.4920859852939));
#54147=CARTESIAN_POINT('Ctrl Pts',(17.492906582814,72.9157109144287,13.4631488791133));
#54148=CARTESIAN_POINT('Ctrl Pts',(17.4877829598304,72.9142409633729,13.410974289667));
#54149=CARTESIAN_POINT('Ctrl Pts',(17.4854804063338,72.9129466223417,13.3877393871097));
#54150=CARTESIAN_POINT('Ctrl Pts',(17.480212541908,72.9085653535684,13.3351527491892));
#54151=CARTESIAN_POINT('Ctrl Pts',(17.4772366060782,72.9050921350123,13.3058480712265));
#54152=CARTESIAN_POINT('Ctrl Pts',(17.470764007199,72.8954241158511,13.2430703679757));
#54153=CARTESIAN_POINT('Ctrl Pts',(17.4672599069287,72.8888976230325,13.2096722547715));
#54154=CARTESIAN_POINT('Ctrl Pts',(17.4552785663747,72.8622539155276,13.0974714049901));
#54155=CARTESIAN_POINT('Ctrl Pts',(17.4466727026678,72.835915210799,13.0203525431545));
#54156=CARTESIAN_POINT('Ctrl Pts',(17.4346671529625,72.7885467973745,12.9157054899961));
#54157=CARTESIAN_POINT('Ctrl Pts',(17.4311837785312,72.7734942208113,12.8856790532571));
#54158=CARTESIAN_POINT('Ctrl Pts',(17.4261308528543,72.7495888537697,12.8423699661083));
#54159=CARTESIAN_POINT('Ctrl Pts',(17.424520240526,72.7416491391683,12.828602775594));
#54160=CARTESIAN_POINT('Ctrl Pts',(17.4215244800588,72.726252905447,12.8030278476934));
#54161=CARTESIAN_POINT('Ctrl Pts',(17.4201366167005,72.718857017671,12.7911885940485));
#54162=CARTESIAN_POINT('Ctrl Pts',(17.4163260743003,72.6978503306809,12.7587636595334));
#54163=CARTESIAN_POINT('Ctrl Pts',(17.4139274502792,72.6838320316976,12.738448206734));
#54164=CARTESIAN_POINT('Ctrl Pts',(17.4047102847599,72.6271666217993,12.661243018992));
#54165=CARTESIAN_POINT('Ctrl Pts',(17.3980744836124,72.5803616724605,12.607560070858));
#54166=CARTESIAN_POINT('Ctrl Pts',(17.3855969523363,72.485010437708,12.51513903227));
#54167=CARTESIAN_POINT('Ctrl Pts',(17.3797837431378,72.4376530323125,12.4754957220317));
#54168=CARTESIAN_POINT('Ctrl Pts',(17.3710765894386,72.3642853098365,12.4226557457685));
#54169=CARTESIAN_POINT('Ctrl Pts',(17.3682848859161,72.3404016426804,12.4066569253156));
#54170=CARTESIAN_POINT('Ctrl Pts',(17.3631783751437,72.2962346105837,12.3791948356042));
#54171=CARTESIAN_POINT('Ctrl Pts',(17.3608748893241,72.2761388957315,12.3674530097827));
#54172=CARTESIAN_POINT('Ctrl Pts',(17.355584371041,72.2296754885995,12.3419906479214));
#54173=CARTESIAN_POINT('Ctrl Pts',(17.352586286185,72.2031271530486,12.3286310852776));
#54174=CARTESIAN_POINT('Ctrl Pts',(17.3460515616181,72.1448887439963,12.3018415765696));
#54175=CARTESIAN_POINT('Ctrl Pts',(17.342507122817,72.1130723463133,12.2887442290114));
#54176=CARTESIAN_POINT('Ctrl Pts',(17.330199531502,72.0018369041351,12.2481520945748));
#54177=CARTESIAN_POINT('Ctrl Pts',(17.3212990734474,71.920244606951,12.2272536875131));
#54178=CARTESIAN_POINT('Ctrl Pts',(17.3091615420306,71.805258828653,12.2096869520533));
#54179=CARTESIAN_POINT('Ctrl Pts',(17.3058165878547,71.7731425209669,12.206027617619));
#54180=CARTESIAN_POINT('Ctrl Pts',(17.300986611431,71.7258801783921,12.2024628763886));
#54181=CARTESIAN_POINT('Ctrl Pts',(17.2994614907288,71.7108221358062,12.2015964985493));
#54182=CARTESIAN_POINT('Ctrl Pts',(17.2965033515242,71.6813097716337,12.2004255184732));
#54183=CARTESIAN_POINT('Ctrl Pts',(17.2950696171364,71.6668588974209,12.2000990396116));
#54184=CARTESIAN_POINT('Ctrl Pts',(17.2908922410192,71.6244055833428,12.1998648881052));
#54185=CARTESIAN_POINT('Ctrl Pts',(17.2881811816254,71.5964056443573,12.2006364165488));
#54186=CARTESIAN_POINT('Ctrl Pts',(17.2813680828183,71.5254472352879,12.20494369563));
#54187=CARTESIAN_POINT('Ctrl Pts',(17.2773071733419,71.4826004675668,12.2097408646399));
#54188=CARTESIAN_POINT('Ctrl Pts',(17.2652595552661,71.3561276267572,12.2304605116588));
#54189=CARTESIAN_POINT('Ctrl Pts',(17.2573205669821,71.2737826252714,12.2526115082165));
#54190=CARTESIAN_POINT('Ctrl Pts',(17.246382167238,71.1676543898231,12.2929400448824));
#54191=CARTESIAN_POINT('Ctrl Pts',(17.2436148525212,71.1413837927782,12.3039475234733));
#54192=CARTESIAN_POINT('Ctrl Pts',(17.2387604746136,71.0964674642345,12.3245690723053));
#54193=CARTESIAN_POINT('Ctrl Pts',(17.2366876816335,71.0776480651545,12.333779708639));
#54194=CARTESIAN_POINT('Ctrl Pts',(17.2317448022951,71.0336793031375,12.3566640749602));
#54195=CARTESIAN_POINT('Ctrl Pts',(17.2288620527013,71.0087488329837,12.3707302178225));
#54196=CARTESIAN_POINT('Ctrl Pts',(17.2192338781193,70.927946956376,12.4199906085542));
#54197=CARTESIAN_POINT('Ctrl Pts',(17.2123729633305,70.8743528616671,12.4586929999178));
#54198=CARTESIAN_POINT('Ctrl Pts',(17.1969043749297,70.7619554551436,12.554004823185));
#54199=CARTESIAN_POINT('Ctrl Pts',(17.1882917929023,70.7050899597244,12.6124798420882));
#54200=CARTESIAN_POINT('Ctrl Pts',(17.1781621912139,70.6433154010782,12.6895962824722));
#54201=CARTESIAN_POINT('Ctrl Pts',(17.1763901216421,70.6327034709,12.7034170891637));
#54202=CARTESIAN_POINT('Ctrl Pts',(17.1732749092283,70.6143638683315,12.7283481756195));
#54203=CARTESIAN_POINT('Ctrl Pts',(17.171925481105,70.6065242720765,12.7393699992256));
#54204=CARTESIAN_POINT('Ctrl Pts',(17.1684960116535,70.5868910510645,12.7679279008583));
#54205=CARTESIAN_POINT('Ctrl Pts',(17.1664316471524,70.5753561939184,12.7856368880158));
#54206=CARTESIAN_POINT('Ctrl Pts',(17.1617108520211,70.549761173074,12.8271626154225));
#54207=CARTESIAN_POINT('Ctrl Pts',(17.159069362936,70.5360258941914,12.8511674602022));
#54208=CARTESIAN_POINT('Ctrl Pts',(17.1482066816013,70.4824396322375,12.9523469459207));
#54209=CARTESIAN_POINT('Ctrl Pts',(17.1401610702817,70.4497735727928,13.0330565493502));
#54210=CARTESIAN_POINT('Ctrl Pts',(17.1280650425046,70.4143337348233,13.1553361020459));
#54211=CARTESIAN_POINT('Ctrl Pts',(17.1241858023781,70.4049344902848,13.194714443131));
#54212=CARTESIAN_POINT('Ctrl Pts',(17.1178742009827,70.3929044227454,13.2584564757103));
#54213=CARTESIAN_POINT('Ctrl Pts',(17.1154798966656,70.3890703477681,13.2825661655011));
#54214=CARTESIAN_POINT('Ctrl Pts',(17.1106174439605,70.3827576480057,13.3312741583634));
#54215=CARTESIAN_POINT('Ctrl Pts',(17.1081498100667,70.3802978913764,13.3558640793717));
#54216=CARTESIAN_POINT('Ctrl Pts',(17.101346884584,70.3755411730672,13.4231998794733));
#54217=CARTESIAN_POINT('Ctrl Pts',(17.0969706808001,70.3746857316654,13.4660104356851));
#54218=CARTESIAN_POINT('Ctrl Pts',(17.0859018536995,70.3779506641692,13.572892161135));
#54219=CARTESIAN_POINT('Ctrl Pts',(17.0791547862547,70.3847637419577,13.6367609420507));
#54220=CARTESIAN_POINT('Ctrl Pts',(17.067050200821,70.4055949277603,13.7499674835915));
#54221=CARTESIAN_POINT('Ctrl Pts',(17.0617036569602,70.4178309180044,13.7995052637551));
#54222=CARTESIAN_POINT('Ctrl Pts',(17.0545203528982,70.4386360901675,13.8662037324912));
#54223=CARTESIAN_POINT('Ctrl Pts',(17.0525944326425,70.4446606084608,13.8841033494241));
#54224=CARTESIAN_POINT('Ctrl Pts',(17.0493356287976,70.4556459059956,13.914483150699));
#54225=CARTESIAN_POINT('Ctrl Pts',(17.0479932601698,70.460408792843,13.9270295105315));
#54226=CARTESIAN_POINT('Ctrl Pts',(17.0447573498571,70.4724689026983,13.957341080051));
#54227=CARTESIAN_POINT('Ctrl Pts',(17.0428751147352,70.4799717218789,13.9750205575763));
#54228=CARTESIAN_POINT('Ctrl Pts',(17.0354731465754,70.5113260111044,14.044478359014));
#54229=CARTESIAN_POINT('Ctrl Pts',(17.0300925955928,70.5382534603744,14.0948021249747));
#54230=CARTESIAN_POINT('Ctrl Pts',(17.0185997033284,70.6030362158332,14.1984429932677));
#54231=CARTESIAN_POINT('Ctrl Pts',(17.0125116167312,70.6417826788887,14.2509570679605));
#54232=CARTESIAN_POINT('Ctrl Pts',(17.0063123822734,70.684359077848,14.3002411372302));
#54233=CARTESIAN_POINT('Origin',(21.26284859951,71.6454,13.47));
#54234=CARTESIAN_POINT('',(16.0430985027246,70.6843589375946,14.3002409748806));
#54235=CARTESIAN_POINT('',(16.2122439422732,70.6843594233383,14.3002415371503));
#54236=CARTESIAN_POINT('',(21.26284859951,70.6843589433668,14.3002409815622));
#54237=CARTESIAN_POINT('',(16.7267333334667,71.6459398759342,14.7399998852496));
#54238=CARTESIAN_POINT('Ctrl Pts',(16.0430985027246,70.6843589375946,14.3002409748806));
#54239=CARTESIAN_POINT('Ctrl Pts',(16.0457968979002,70.6674222330724,14.2806359818724));
#54240=CARTESIAN_POINT('Ctrl Pts',(16.0484768065757,70.6510861315913,14.2605135379007));
#54241=CARTESIAN_POINT('Ctrl Pts',(16.0527622312145,70.6256610843513,14.2271586801896));
#54242=CARTESIAN_POINT('Ctrl Pts',(16.0543868472531,70.6161889809723,14.214232150367));
#54243=CARTESIAN_POINT('Ctrl Pts',(16.0573913841616,70.598958209715,14.1897589394869));
#54244=CARTESIAN_POINT('Ctrl Pts',(16.0587743359645,70.5911407522425,14.1782590115397));
#54245=CARTESIAN_POINT('Ctrl Pts',(16.062541736419,70.5701951498698,14.1463312665806));
#54246=CARTESIAN_POINT('Ctrl Pts',(16.0649031021133,70.5574609504884,14.1256510850315));
#54247=CARTESIAN_POINT('Ctrl Pts',(16.0740356478369,70.5100715005747,14.0435039596709));
#54248=CARTESIAN_POINT('Ctrl Pts',(16.0806243220723,70.4799661824146,13.9795527786189));
#54249=CARTESIAN_POINT('Ctrl Pts',(16.0931429713713,70.4334428877496,13.8546925219963));
#54250=CARTESIAN_POINT('Ctrl Pts',(16.0990465919072,70.4159394548933,13.79442807718));
#54251=CARTESIAN_POINT('Ctrl Pts',(16.1078560149509,70.3969842815363,13.704923595019));
#54252=CARTESIAN_POINT('Ctrl Pts',(16.1106555016447,70.3919745181581,13.6765312641368));
#54253=CARTESIAN_POINT('Ctrl Pts',(16.1157700230282,70.3846731502045,13.6249501327009));
#54254=CARTESIAN_POINT('Ctrl Pts',(16.1180735670501,70.3820454634826,13.6018213627777));
#54255=CARTESIAN_POINT('Ctrl Pts',(16.1233558714868,70.3775199257024,13.5491095100516));
#54256=CARTESIAN_POINT('Ctrl Pts',(16.1263455138177,70.3760194991303,13.5195073329416));
#54257=CARTESIAN_POINT('Ctrl Pts',(16.132856267677,70.3750194387979,13.45563679349));
#54258=CARTESIAN_POINT('Ctrl Pts',(16.1363850341362,70.3758688426986,13.4213869355575));
#54259=CARTESIAN_POINT('Ctrl Pts',(16.1485626788231,70.3835070596596,13.304456328561));
#54260=CARTESIAN_POINT('Ctrl Pts',(16.1573453525061,70.3970073472099,13.2224265162086));
#54261=CARTESIAN_POINT('Ctrl Pts',(16.1694847267194,70.4270053216461,13.1101034867471));
#54262=CARTESIAN_POINT('Ctrl Pts',(16.1729384506198,70.4368717438836,13.0782461280851));
#54263=CARTESIAN_POINT('Ctrl Pts',(16.1778891261556,70.4530531023261,13.0324608572622));
#54264=CARTESIAN_POINT('Ctrl Pts',(16.1794289167543,70.4583824481663,13.0182024360809));
#54265=CARTESIAN_POINT('Ctrl Pts',(16.1823920958983,70.469233471263,12.9906897528119));
#54266=CARTESIAN_POINT('Ctrl Pts',(16.1838165694037,70.4747259248912,12.9774268798847));
#54267=CARTESIAN_POINT('Ctrl Pts',(16.1879200104552,70.4913256204301,12.9391900256512));
#54268=CARTESIAN_POINT('Ctrl Pts',(16.1905682066448,70.5030165192185,12.914475699644));
#54269=CARTESIAN_POINT('Ctrl Pts',(16.1971564154835,70.5343774926917,12.8533647998398));
#54270=CARTESIAN_POINT('Ctrl Pts',(16.2010587474533,70.5550449202772,12.8175152148751));
#54271=CARTESIAN_POINT('Ctrl Pts',(16.2133148394049,70.6255639530281,12.7079323550637));
#54272=CARTESIAN_POINT('Ctrl Pts',(16.2216049834242,70.6814206568381,12.6384027979274));
#54273=CARTESIAN_POINT('Ctrl Pts',(16.232889006636,70.7638751976796,12.5553395806403));
#54274=CARTESIAN_POINT('Ctrl Pts',(16.2356214223749,70.784326892134,12.536060771956));
#54275=CARTESIAN_POINT('Ctrl Pts',(16.2406726793659,70.8228793148967,12.5020625543492));
#54276=CARTESIAN_POINT('Ctrl Pts',(16.2429815654238,70.8407788325318,12.4871328802961));
#54277=CARTESIAN_POINT('Ctrl Pts',(16.2483612149538,70.8830482039205,12.4538053636938));
#54278=CARTESIAN_POINT('Ctrl Pts',(16.2514446714262,70.9076898003573,12.435778039574));
#54279=CARTESIAN_POINT('Ctrl Pts',(16.2612931713798,70.9875625533193,12.3816519974347));
#54280=CARTESIAN_POINT('Ctrl Pts',(16.2681664630672,71.0449615646673,12.3489637362893));
#54281=CARTESIAN_POINT('Ctrl Pts',(16.2829762029345,71.1725051602726,12.2889420006337));
#54282=CARTESIAN_POINT('Ctrl Pts',(16.2909028634937,71.243084278038,12.2630734331405));
#54283=CARTESIAN_POINT('Ctrl Pts',(16.3004361507145,71.3327718454888,12.2389508386255));
#54284=CARTESIAN_POINT('Ctrl Pts',(16.3022535096169,71.3501006586327,12.2346794669514));
#54285=CARTESIAN_POINT('Ctrl Pts',(16.3054072904684,71.3806378251507,12.2278317949933));
#54286=CARTESIAN_POINT('Ctrl Pts',(16.3067509586642,71.3938058723744,12.225097873495));
#54287=CARTESIAN_POINT('Ctrl Pts',(16.3100682562025,71.4266897744507,12.2188137684601));
#54288=CARTESIAN_POINT('Ctrl Pts',(16.3120287117846,71.4464506851388,12.2155198353924));
#54289=CARTESIAN_POINT('Ctrl Pts',(16.3164494241793,71.4915824854841,12.2090903230319));
#54290=CARTESIAN_POINT('Ctrl Pts',(16.3188974282113,71.5169870352588,12.2062502681149));
#54291=CARTESIAN_POINT('Ctrl Pts',(16.3280224752007,71.6126231325824,12.198473047548));
#54292=CARTESIAN_POINT('Ctrl Pts',(16.3345741363555,71.6831402226275,12.1986102755095));
#54293=CARTESIAN_POINT('Ctrl Pts',(16.3461695590771,71.8056954850464,12.2090590389518));
#54294=CARTESIAN_POINT('Ctrl Pts',(16.3511627399253,71.8577702626365,12.2167783960845));
#54295=CARTESIAN_POINT('Ctrl Pts',(16.3588053718384,71.9350439962628,12.2331880600946));
#54296=CARTESIAN_POINT('Ctrl Pts',(16.361381637426,71.9606968865318,12.2394777316628));
#54297=CARTESIAN_POINT('Ctrl Pts',(16.366305144797,72.0088335147517,12.2528839972188));
#54298=CARTESIAN_POINT('Ctrl Pts',(16.3686461991881,72.0313516823379,12.2598362103956));
#54299=CARTESIAN_POINT('Ctrl Pts',(16.3743790819279,72.0855139863246,12.2782235192926));
#54300=CARTESIAN_POINT('Ctrl Pts',(16.3777900561168,72.1169201757066,12.2902967742913));
#54301=CARTESIAN_POINT('Ctrl Pts',(16.3884831092456,72.2127057857513,12.3315548066305));
#54302=CARTESIAN_POINT('Ctrl Pts',(16.3958819671871,72.2751484555832,12.3648723377557));
#54303=CARTESIAN_POINT('Ctrl Pts',(16.4097904124291,72.3862180546076,12.4366166187168));
#54304=CARTESIAN_POINT('Ctrl Pts',(16.4162725582957,72.4354551667727,12.4737535123514));
#54305=CARTESIAN_POINT('Ctrl Pts',(16.4245334987823,72.4959311524592,12.5266819004187));
#54306=CARTESIAN_POINT('Ctrl Pts',(16.4264475117904,72.5097805834224,12.5393558027144));
#54307=CARTESIAN_POINT('Ctrl Pts',(16.4296948513491,72.5330448506227,12.561613069218));
#54308=CARTESIAN_POINT('Ctrl Pts',(16.4310374147878,72.542596666844,12.5710459435503));
#54309=CARTESIAN_POINT('Ctrl Pts',(16.4342861248444,72.5655363158127,12.5944299779381));
#54310=CARTESIAN_POINT('Ctrl Pts',(16.4361806747742,72.5787584468723,12.6085385306702));
#54311=CARTESIAN_POINT('Ctrl Pts',(16.4437093813169,72.6304700397462,12.6663061199528));
#54312=CARTESIAN_POINT('Ctrl Pts',(16.4491985022156,72.6662651905521,12.7122908582067));
#54313=CARTESIAN_POINT('Ctrl Pts',(16.4627012773735,72.7464985118428,12.8314247455208));
#54314=CARTESIAN_POINT('Ctrl Pts',(16.4706719241718,72.7869384116978,12.90689797198));
#54315=CARTESIAN_POINT('Ctrl Pts',(16.4816418452697,72.8303412577702,13.0121533431639));
#54316=CARTESIAN_POINT('Ctrl Pts',(16.484406477761,72.8402987091472,13.0388084760384));
#54317=CARTESIAN_POINT('Ctrl Pts',(16.4894657680989,72.8566930970429,13.0876376318978));
#54318=CARTESIAN_POINT('Ctrl Pts',(16.4917493785743,72.863436511984,13.109696196646));
#54319=CARTESIAN_POINT('Ctrl Pts',(16.497041839608,72.8775424293203,13.1607738630282));
#54320=CARTESIAN_POINT('Ctrl Pts',(16.5000625507064,72.8844864841561,13.189892737007));
#54321=CARTESIAN_POINT('Ctrl Pts',(16.506660675449,72.8972627991428,13.2533223385596));
#54322=CARTESIAN_POINT('Ctrl Pts',(16.510246259894,72.9027262477712,13.2876819193343));
#54323=CARTESIAN_POINT('Ctrl Pts',(16.5229015036442,72.9168880680095,13.4085588906867));
#54324=CARTESIAN_POINT('Ctrl Pts',(16.5321173608654,72.9181116066767,13.4957021797642));
#54325=CARTESIAN_POINT('Ctrl Pts',(16.5442613612533,72.9078021753878,13.6118516610837));
#54326=CARTESIAN_POINT('Ctrl Pts',(16.5473280716812,72.9041415624331,13.6413220482175));
#54327=CARTESIAN_POINT('Ctrl Pts',(16.5518469196775,72.8971273743986,13.6851624261185));
#54328=CARTESIAN_POINT('Ctrl Pts',(16.5533324775568,72.8945516433668,13.6996443741214));
#54329=CARTESIAN_POINT('Ctrl Pts',(16.5562845024886,72.8888808433309,13.7286007425306));
#54330=CARTESIAN_POINT('Ctrl Pts',(16.5577506007882,72.8857832100899,13.7430723719536));
#54331=CARTESIAN_POINT('Ctrl Pts',(16.5621818089575,72.8755755493909,13.7869949786106));
#54332=CARTESIAN_POINT('Ctrl Pts',(16.5651078589645,72.8676635913933,13.816251183943));
#54333=CARTESIAN_POINT('Ctrl Pts',(16.5727350589945,72.8440929937661,13.8924731543663));
#54334=CARTESIAN_POINT('Ctrl Pts',(16.5773813486742,72.8267228578877,13.9388556034495));
#54335=CARTESIAN_POINT('Ctrl Pts',(16.5889057482074,72.7770485600492,14.0510616891612));
#54336=CARTESIAN_POINT('Ctrl Pts',(16.5957693602683,72.7416776939111,14.1153172774884));
#54337=CARTESIAN_POINT('Ctrl Pts',(16.6056231888466,72.6847402958427,14.2004272484636));
#54338=CARTESIAN_POINT('Ctrl Pts',(16.6084567155664,72.6676779472616,14.2241218101357));
#54339=CARTESIAN_POINT('Ctrl Pts',(16.6136045941521,72.6355746532537,14.2656102737153));
#54340=CARTESIAN_POINT('Ctrl Pts',(16.6159066835507,72.6208313240242,14.2836185268508));
#54341=CARTESIAN_POINT('Ctrl Pts',(16.6211474212582,72.5864613865069,14.3233222143153));
#54342=CARTESIAN_POINT('Ctrl Pts',(16.6240961612231,72.5665639342111,14.3447639619623));
#54343=CARTESIAN_POINT('Ctrl Pts',(16.6304924747682,72.5222842886282,14.3892932357848));
#54344=CARTESIAN_POINT('Ctrl Pts',(16.6339470456236,72.4976910599992,14.4121388427561));
#54345=CARTESIAN_POINT('Ctrl Pts',(16.6455457431029,72.4129073320717,14.484859386742));
#54346=CARTESIAN_POINT('Ctrl Pts',(16.6538087375679,72.3490231210971,14.5301508471307));
#54347=CARTESIAN_POINT('Ctrl Pts',(16.6659248330474,72.2488482508594,14.5881071698422));
#54348=CARTESIAN_POINT('Ctrl Pts',(16.6698334605561,72.2154821875759,14.6054824716453));
#54349=CARTESIAN_POINT('Ctrl Pts',(16.6753098507987,72.1668898627127,14.6281036878441));
#54350=CARTESIAN_POINT('Ctrl Pts',(16.6769315198381,72.1522619251528,14.6345801429689));
#54351=CARTESIAN_POINT('Ctrl Pts',(16.6799342636315,72.1246845391829,14.6461717617547));
#54352=CARTESIAN_POINT('Ctrl Pts',(16.6813183016168,72.1117676062248,14.6513530277532));
#54353=CARTESIAN_POINT('Ctrl Pts',(16.6850949991853,72.0760079642927,14.6650189822818));
#54354=CARTESIAN_POINT('Ctrl Pts',(16.6874643684248,72.053001423548,14.6730606542094));
#54355=CARTESIAN_POINT('Ctrl Pts',(16.7023510980548,71.9056438873701,14.7198541786761));
#54356=CARTESIAN_POINT('Ctrl Pts',(16.7142149269752,71.776189436049,14.7399445162659));
#54357=CARTESIAN_POINT('Ctrl Pts',(16.7267333334667,71.6459398759342,14.7399998852496));
#54358=CARTESIAN_POINT('Ctrl Pts',(16.7267334568494,71.6459385921818,14.7399998857947));
#54359=CARTESIAN_POINT('Ctrl Pts',(16.7283087818113,71.6295479013485,14.740006836896));
#54360=CARTESIAN_POINT('Ctrl Pts',(16.7298917004701,71.6131592909544,14.7396964791053));
#54361=CARTESIAN_POINT('Ctrl Pts',(16.7330390453341,71.580778104527,14.7384559543814));
#54362=CARTESIAN_POINT('Ctrl Pts',(16.7346027597629,71.5647882063487,14.737540209352));
#54363=CARTESIAN_POINT('Ctrl Pts',(16.7382648806629,71.5276094436234,14.734704677072));
#54364=CARTESIAN_POINT('Ctrl Pts',(16.7403696744464,71.5064438224708,14.7325543873976));
#54365=CARTESIAN_POINT('Ctrl Pts',(16.7453608999044,71.4567999988391,14.7262475601839));
#54366=CARTESIAN_POINT('Ctrl Pts',(16.7482597949872,71.4283908518236,14.7216527421321));
#54367=CARTESIAN_POINT('Ctrl Pts',(16.7575898068153,71.3384385650118,14.7039499174054));
#54368=CARTESIAN_POINT('Ctrl Pts',(16.7641223705281,71.2777112705777,14.6872345896589));
#54369=CARTESIAN_POINT('Ctrl Pts',(16.7781172477619,71.1520650620468,14.6423880758682));
#54370=CARTESIAN_POINT('Ctrl Pts',(16.7855743677902,71.0877359687437,14.6131906449981));
#54371=CARTESIAN_POINT('Ctrl Pts',(16.7953939221386,71.004987842676,14.5669778454279));
#54372=CARTESIAN_POINT('Ctrl Pts',(16.7978859896184,70.9841553711275,14.5545477964833));
#54373=CARTESIAN_POINT('Ctrl Pts',(16.8017562938427,70.9519619005673,14.5340661676507));
#54374=CARTESIAN_POINT('Ctrl Pts',(16.8031554588882,70.9403563019843,14.5264121756627));
#54375=CARTESIAN_POINT('Ctrl Pts',(16.8061409864774,70.9156406799535,14.509523135718));
#54376=CARTESIAN_POINT('Ctrl Pts',(16.8077235302394,70.9025754642845,14.5002275561205));
#54377=CARTESIAN_POINT('Ctrl Pts',(16.8126723557012,70.861939127614,14.4701405988433));
#54378=CARTESIAN_POINT('Ctrl Pts',(16.8159887023894,70.8350353009879,14.4484691314138));
#54379=CARTESIAN_POINT('Ctrl Pts',(16.8248913408023,70.7645987474944,14.3868301062798));
#54380=CARTESIAN_POINT('Ctrl Pts',(16.8304053615477,70.7229380551678,14.3448980371615));
#54381=CARTESIAN_POINT('Ctrl Pts',(16.8359541306755,70.6843588624425,14.3002408878887));
#54382=CARTESIAN_POINT('',(16.8971557431799,71.644308511249,14.7399995524375));
#54383=CARTESIAN_POINT('Ctrl Pts',(17.0063123822734,70.684359077848,14.3002411372302));
#54384=CARTESIAN_POINT('Ctrl Pts',(17.004197651672,70.698883066962,14.3170532984994));
#54385=CARTESIAN_POINT('Ctrl Pts',(17.0020705965369,70.7138527786965,14.3334896321051));
#54386=CARTESIAN_POINT('Ctrl Pts',(16.9972041541103,70.7488190402137,14.3699114831557));
#54387=CARTESIAN_POINT('Ctrl Pts',(16.9944579065253,70.7690565036005,14.3896302987457));
#54388=CARTESIAN_POINT('Ctrl Pts',(16.9893944179429,70.8071477492386,14.4243456783912));
#54389=CARTESIAN_POINT('Ctrl Pts',(16.9870874591459,70.824789601238,14.4395570667382));
#54390=CARTESIAN_POINT('Ctrl Pts',(16.9817318988848,70.8663295627702,14.4734281181958));
#54391=CARTESIAN_POINT('Ctrl Pts',(16.9786710336641,70.8904963976887,14.4917332802506));
#54392=CARTESIAN_POINT('Ctrl Pts',(16.9676687233899,70.9787221351955,14.5537204766961));
#54393=CARTESIAN_POINT('Ctrl Pts',(16.959562782828,71.0460874754797,14.5923767615868));
#54394=CARTESIAN_POINT('Ctrl Pts',(16.9448515577804,71.1732459639556,14.6506187042339));
#54395=CARTESIAN_POINT('Ctrl Pts',(16.9382850872234,71.2317927333729,14.6723812401327));
#54396=CARTESIAN_POINT('Ctrl Pts',(16.9299447864436,71.3097225241116,14.6949785555521));
#54397=CARTESIAN_POINT('Ctrl Pts',(16.9280320252777,71.3278528476496,14.6998031435263));
#54398=CARTESIAN_POINT('Ctrl Pts',(16.9247861977611,71.3591281407649,14.7073877921821));
#54399=CARTESIAN_POINT('Ctrl Pts',(16.9234439153868,71.3722203610649,14.7103439313893));
#54400=CARTESIAN_POINT('Ctrl Pts',(16.9207753841692,71.3985577590331,14.7158534155939));
#54401=CARTESIAN_POINT('Ctrl Pts',(16.9194490701011,71.411800421194,14.7184042274095));
#54402=CARTESIAN_POINT('Ctrl Pts',(16.9161224519484,71.4453424246085,14.724312633018));
#54403=CARTESIAN_POINT('Ctrl Pts',(16.9141347009732,71.465688166774,14.7273889680941));
#54404=CARTESIAN_POINT('Ctrl Pts',(16.9070905615411,71.5385729425552,14.7366038270448));
#54405=CARTESIAN_POINT('Ctrl Pts',(16.9021236939593,71.5914116579932,14.7399540766915));
#54406=CARTESIAN_POINT('Ctrl Pts',(16.8971556908388,71.644308689214,14.7399995311183));
#54407=CARTESIAN_POINT('Ctrl Pts',(16.8971557078627,71.6443085079506,14.7399995309626));
#54408=CARTESIAN_POINT('Ctrl Pts',(16.8898238968171,71.7223742875591,14.7400666240407));
#54409=CARTESIAN_POINT('Ctrl Pts',(16.882508327921,71.8002722681029,14.7329359717819));
#54410=CARTESIAN_POINT('Ctrl Pts',(16.8727912006366,71.8993012955568,14.7145672832214));
#54411=CARTESIAN_POINT('Ctrl Pts',(16.8705895249596,71.9214674462307,14.7098387834532));
#54412=CARTESIAN_POINT('Ctrl Pts',(16.8660858590211,71.9661548910853,14.699048318925));
#54413=CARTESIAN_POINT('Ctrl Pts',(16.8637836867908,71.9886591633842,14.6929539814569));
#54414=CARTESIAN_POINT('Ctrl Pts',(16.8586773709661,72.0377433907596,14.6782001431898));
#54415=CARTESIAN_POINT('Ctrl Pts',(16.8558658082793,72.0642299333635,14.6692756567084));
#54416=CARTESIAN_POINT('Ctrl Pts',(16.8439362426966,72.1741923750001,14.6281376483414));
#54417=CARTESIAN_POINT('Ctrl Pts',(16.8345724598089,72.2544218625557,14.588029396472));
#54418=CARTESIAN_POINT('Ctrl Pts',(16.8208188623443,72.364563975149,14.5175736741248));
#54419=CARTESIAN_POINT('Ctrl Pts',(16.8164753270358,72.3982672151862,14.4936204339921));
#54420=CARTESIAN_POINT('Ctrl Pts',(16.8093410991244,72.4522114516593,14.4511735044182));
#54421=CARTESIAN_POINT('Ctrl Pts',(16.8065250984956,72.4731304823411,14.4335915921712));
#54422=CARTESIAN_POINT('Ctrl Pts',(16.8022893732432,72.5041490837958,14.4057648737795));
#54423=CARTESIAN_POINT('Ctrl Pts',(16.8008418512951,72.5146678438209,14.396001831948));
#54424=CARTESIAN_POINT('Ctrl Pts',(16.7978870823546,72.5359959971195,14.3755221262385));
#54425=CARTESIAN_POINT('Ctrl Pts',(16.79638145965,72.5467826692345,14.3647854026018));
#54426=CARTESIAN_POINT('Ctrl Pts',(16.7916178843376,72.5805686988698,14.3299245332641));
#54427=CARTESIAN_POINT('Ctrl Pts',(16.7884082804306,72.6028148749541,14.3050856558141));
#54428=CARTESIAN_POINT('Ctrl Pts',(16.7773253388925,72.6769157129473,14.2154886056859));
#54429=CARTESIAN_POINT('Ctrl Pts',(16.7696355309042,72.7233863344534,14.1465537832464));
#54430=CARTESIAN_POINT('Ctrl Pts',(16.758556340246,72.7790822133142,14.0434435984024));
#54431=CARTESIAN_POINT('Ctrl Pts',(16.7552993748435,72.794131917593,14.01266707184));
#54432=CARTESIAN_POINT('Ctrl Pts',(16.7491571198527,72.8198488467096,13.954198254189));
#54433=CARTESIAN_POINT('Ctrl Pts',(16.7462829079392,72.8308249652517,13.9266676830575));
#54434=CARTESIAN_POINT('Ctrl Pts',(16.7410947149974,72.8486841728902,13.8768767856202));
#54435=CARTESIAN_POINT('Ctrl Pts',(16.7387939227902,72.8559366580059,13.8547627098241));
#54436=CARTESIAN_POINT('Ctrl Pts',(16.7335990037933,72.8708010811997,13.8048469867171));
#54437=CARTESIAN_POINT('Ctrl Pts',(16.730695657524,72.8780819001586,13.7769614150034));
#54438=CARTESIAN_POINT('Ctrl Pts',(16.7213875882034,72.8981626607147,13.6877386912922));
#54439=CARTESIAN_POINT('Ctrl Pts',(16.714882684886,72.9073744481245,13.625699308249));
#54440=CARTESIAN_POINT('Ctrl Pts',(16.7009097523629,72.9171544489058,13.4928537296476));
#54441=CARTESIAN_POINT('Ctrl Pts',(16.6934460971044,72.9164598121784,13.4221515159564));
#54442=CARTESIAN_POINT('Ctrl Pts',(16.6836151426093,72.9076342362242,13.3276798310376));
#54443=CARTESIAN_POINT('Ctrl Pts',(16.6811183426748,72.9046803614261,13.3035562331351));
#54444=CARTESIAN_POINT('Ctrl Pts',(16.6772429129132,72.8989504209894,13.2657827898844));
#54445=CARTESIAN_POINT('Ctrl Pts',(16.6758432547822,72.8966392856017,13.2520695727065));
#54446=CARTESIAN_POINT('Ctrl Pts',(16.6728592699188,72.8911832000533,13.2226529515872));
#54447=CARTESIAN_POINT('Ctrl Pts',(16.6712787153827,72.8879656900088,13.2069658901296));
#54448=CARTESIAN_POINT('Ctrl Pts',(16.6663453493649,72.8769068257915,13.1577925972059));
#54449=CARTESIAN_POINT('Ctrl Pts',(16.6630420265283,72.8680010488162,13.1245585085759));
#54450=CARTESIAN_POINT('Ctrl Pts',(16.6521171240674,72.8337932408401,13.0149245286979));
#54451=CARTESIAN_POINT('Ctrl Pts',(16.6446521472556,72.8025869702987,12.9405741658649));
#54452=CARTESIAN_POINT('Ctrl Pts',(16.6338376972792,72.7485319296961,12.8398024620172));
#54453=CARTESIAN_POINT('Ctrl Pts',(16.6306128764712,72.7313208429047,12.8105877093923));
#54454=CARTESIAN_POINT('Ctrl Pts',(16.624521374348,72.6970194685702,12.7573549754655));
#54455=CARTESIAN_POINT('Ctrl Pts',(16.6216653789363,72.6802218495953,12.7331758277679));
#54456=CARTESIAN_POINT('Ctrl Pts',(16.616495560632,72.6486698053715,12.6909678536147));
#54457=CARTESIAN_POINT('Ctrl Pts',(16.6141945154045,72.6342302321114,12.6727196331824));
#54458=CARTESIAN_POINT('Ctrl Pts',(16.6089806080293,72.6006880935583,12.6326437718998));
#54459=CARTESIAN_POINT('Ctrl Pts',(16.6060581555061,72.5813233460385,12.6110541684249));
#54460=CARTESIAN_POINT('Ctrl Pts',(16.5951373623247,72.5070105948463,12.5337019418147));
#54461=CARTESIAN_POINT('Ctrl Pts',(16.586964625559,72.4476908140349,12.4824010763034));
#54462=CARTESIAN_POINT('Ctrl Pts',(16.5738449414483,72.3462099571882,12.4098451833775));
#54463=CARTESIAN_POINT('Ctrl Pts',(16.5689473042014,72.3069196023169,12.3848939863757));
#54464=CARTESIAN_POINT('Ctrl Pts',(16.5610586935099,72.2408223042171,12.3478464930218));
#54465=CARTESIAN_POINT('Ctrl Pts',(16.5580367864398,72.2148072901669,12.3344243942052));
#54466=CARTESIAN_POINT('Ctrl Pts',(16.5535685769488,72.1751124023486,12.3156520644182));
#54467=CARTESIAN_POINT('Ctrl Pts',(16.5520898803886,72.1617675122463,12.3096211577383));
#54468=CARTESIAN_POINT('Ctrl Pts',(16.5491387126947,72.134675934975,12.2979377812818));
#54469=CARTESIAN_POINT('Ctrl Pts',(16.5476668100528,72.1209283926963,12.2922930712419));
#54470=CARTESIAN_POINT('Ctrl Pts',(16.5431876756537,72.078456251728,12.2757192066058));
#54471=CARTESIAN_POINT('Ctrl Pts',(16.5402207867651,72.0494289784177,12.2655891885108));
#54472=CARTESIAN_POINT('Ctrl Pts',(16.5290909242515,71.9381383450991,12.2312284329666));
#54473=CARTESIAN_POINT('Ctrl Pts',(16.5211475557702,71.8538618847231,12.2142944037521));
#54474=CARTESIAN_POINT('Ctrl Pts',(16.5097712556462,71.7340551849804,12.2026251064423));
#54475=CARTESIAN_POINT('Ctrl Pts',(16.5064798142118,71.6994736477007,12.2006794951786));
#54476=CARTESIAN_POINT('Ctrl Pts',(16.5002832041892,71.6350202433553,12.1996918564423));
#54477=CARTESIAN_POINT('Ctrl Pts',(16.497389538913,71.6051782909937,12.2002864869158));
#54478=CARTESIAN_POINT('Ctrl Pts',(16.4921815380517,71.5521476492758,12.2032144063171));
#54479=CARTESIAN_POINT('Ctrl Pts',(16.4898808301082,71.528949368463,12.205136048595));
#54480=CARTESIAN_POINT('Ctrl Pts',(16.4847050369037,71.477361280463,12.2108404704477));
#54481=CARTESIAN_POINT('Ctrl Pts',(16.4818211101908,71.4490213727214,12.2149482735687));
#54482=CARTESIAN_POINT('Ctrl Pts',(16.4704274426051,71.3388016828337,12.2347485379884));
#54483=CARTESIAN_POINT('Ctrl Pts',(16.4617129656493,71.2584232391943,12.2575264454181));
#54484=CARTESIAN_POINT('Ctrl Pts',(16.4483307050129,71.1400180036888,12.3040600982079));
#54485=CARTESIAN_POINT('Ctrl Pts',(16.4437120140976,71.1000218819484,12.3222239138478));
#54486=CARTESIAN_POINT('Ctrl Pts',(16.4362006204221,71.0359127986102,12.3554478021766));
#54487=CARTESIAN_POINT('Ctrl Pts',(16.4332798130589,71.0112202768836,12.3693103510359));
#54488=CARTESIAN_POINT('Ctrl Pts',(16.4289256651814,70.9746111516071,12.3915045096295));
#54489=CARTESIAN_POINT('Ctrl Pts',(16.4274622125727,70.9623415891651,12.3992332214284));
#54490=CARTESIAN_POINT('Ctrl Pts',(16.424510324749,70.9376334031449,12.4153947945783));
#54491=CARTESIAN_POINT('Ctrl Pts',(16.4230229512688,70.9252067403691,12.4238415784146));
#54492=CARTESIAN_POINT('Ctrl Pts',(16.418527791186,70.887807170194,12.450245623516));
#54493=CARTESIAN_POINT('Ctrl Pts',(16.4155599037374,70.8633318731906,12.4688927062628));
#54494=CARTESIAN_POINT('Ctrl Pts',(16.4057626400288,70.7840574338568,12.5339739358004));
#54495=CARTESIAN_POINT('Ctrl Pts',(16.399077350198,70.7325196459017,12.5841631690511));
#54496=CARTESIAN_POINT('Ctrl Pts',(16.3884990156058,70.6589424000847,12.6690966385489));
#54497=CARTESIAN_POINT('Ctrl Pts',(16.3846650008126,70.6338732437256,12.7010019877807));
#54498=CARTESIAN_POINT('Ctrl Pts',(16.3776251335946,70.5912511671718,12.7609447818084));
#54499=CARTESIAN_POINT('Ctrl Pts',(16.3744382434487,70.5731850605043,12.7885722600957));
#54500=CARTESIAN_POINT('Ctrl Pts',(16.3689156801596,70.5441338948886,12.8370189780933));
#54501=CARTESIAN_POINT('Ctrl Pts',(16.3666003378791,70.5326135603664,12.8574984334671));
#54502=CARTESIAN_POINT('Ctrl Pts',(16.3616129423117,70.5092428383312,12.9018819068115));
#54503=CARTESIAN_POINT('Ctrl Pts',(16.3589362322345,70.4975646688587,12.9258630252757));
#54504=CARTESIAN_POINT('Ctrl Pts',(16.3499637333487,70.4613233356284,13.0066516777853));
#54505=CARTESIAN_POINT('Ctrl Pts',(16.3435637629278,70.4401609084647,13.0648762941052));
#54506=CARTESIAN_POINT('Ctrl Pts',(16.3305192953921,70.4062530715105,13.1847775819259));
#54507=CARTESIAN_POINT('Ctrl Pts',(16.323889959174,70.3936766742012,13.2463360191253));
#54508=CARTESIAN_POINT('Ctrl Pts',(16.314790398906,70.3826056291999,13.3327283247775));
#54509=CARTESIAN_POINT('Ctrl Pts',(16.3122596482475,70.3802052275293,13.3569711872318));
#54510=CARTESIAN_POINT('Ctrl Pts',(16.3077592854686,70.3771496701396,13.4005987307025));
#54511=CARTESIAN_POINT('Ctrl Pts',(16.305781318091,70.3762383182268,13.4199579299138));
#54512=CARTESIAN_POINT('Ctrl Pts',(16.3024702415047,70.3754462288665,13.4527500364809));
#54513=CARTESIAN_POINT('Ctrl Pts',(16.3011265890288,70.375334822483,13.4661722607109));
#54514=CARTESIAN_POINT('Ctrl Pts',(16.2979361231732,70.3755776894921,13.498314059199));
#54515=CARTESIAN_POINT('Ctrl Pts',(16.2960995219557,70.3761329523695,13.5170285701444));
#54516=CARTESIAN_POINT('Ctrl Pts',(16.2878658788132,70.380515568799,13.6015990975334));
#54517=CARTESIAN_POINT('Ctrl Pts',(16.2816652417856,70.3890566987688,13.6671174483649));
#54518=CARTESIAN_POINT('Ctrl Pts',(16.2702951158908,70.413997414888,13.7855615517722));
#54519=CARTESIAN_POINT('Ctrl Pts',(16.2651374889677,70.4288330941904,13.8386405024776));
#54520=CARTESIAN_POINT('Ctrl Pts',(16.2581238708754,70.4532608742622,13.9082400229729));
#54521=CARTESIAN_POINT('Ctrl Pts',(16.2563372939143,70.4598456501824,13.9257530393238));
#54522=CARTESIAN_POINT('Ctrl Pts',(16.2516214080036,70.4781362916253,13.9713173413683));
#54523=CARTESIAN_POINT('Ctrl Pts',(16.2486767319952,70.4904656348527,13.9991029299502));
#54524=CARTESIAN_POINT('Ctrl Pts',(16.2434159765917,70.5139846694955,14.0473577981535));
#54525=CARTESIAN_POINT('Ctrl Pts',(16.2411146758863,70.524764307304,14.0680118269868));
#54526=CARTESIAN_POINT('Ctrl Pts',(16.2359839859797,70.5498299777805,14.1129781865077));
#54527=CARTESIAN_POINT('Ctrl Pts',(16.2331466684602,70.5643695712019,14.1371338078886));
#54528=CARTESIAN_POINT('Ctrl Pts',(16.2243594646087,70.611385522011,14.2096672950747));
#54529=CARTESIAN_POINT('Ctrl Pts',(16.2183306860113,70.6463625582953,14.2562585184042));
#54530=CARTESIAN_POINT('Ctrl Pts',(16.2122439422732,70.6843594233383,14.3002415371503));
#54531=CARTESIAN_POINT('Origin',(21.26284859951,71.6454,13.47));
#54532=CARTESIAN_POINT('',(15.2474530402596,70.6843589428744,14.3002409809922));
#54533=CARTESIAN_POINT('',(15.4172344952204,70.6843589433712,14.3002409815673));
#54534=CARTESIAN_POINT('',(21.26284859951,70.6843589433668,14.3002409815622));
#54535=CARTESIAN_POINT('Ctrl Pts',(15.2474530402596,70.6843589428744,14.3002409809922));
#54536=CARTESIAN_POINT('Ctrl Pts',(15.2478512541151,70.6817427021451,14.2972125653711));
#54537=CARTESIAN_POINT('Ctrl Pts',(15.2482500501357,70.6791407556303,14.2941717597417));
#54538=CARTESIAN_POINT('Ctrl Pts',(15.2515639828624,70.6576700862129,14.2688382842419));
#54539=CARTESIAN_POINT('Ctrl Pts',(15.2545084970404,70.6395632294921,14.2459156060063));
#54540=CARTESIAN_POINT('Ctrl Pts',(15.2647675752268,70.5798883327756,14.164767005487));
#54541=CARTESIAN_POINT('Ctrl Pts',(15.2722210661029,70.5424644562559,14.1036764139342));
#54542=CARTESIAN_POINT('Ctrl Pts',(15.2850536696927,70.4876847424598,13.9945528002066));
#54543=CARTESIAN_POINT('Ctrl Pts',(15.2903883927735,70.4677060149305,13.9480141297845));
#54544=CARTESIAN_POINT('Ctrl Pts',(15.2988584625137,70.4401642786459,13.8715559548569));
#54545=CARTESIAN_POINT('Ctrl Pts',(15.3020291120978,70.430818933401,13.8423353515714));
#54546=CARTESIAN_POINT('Ctrl Pts',(15.3066646878291,70.4185313342746,13.7985023820193));
#54547=CARTESIAN_POINT('Ctrl Pts',(15.3081654726918,70.4147736088042,13.7841326150186));
#54548=CARTESIAN_POINT('Ctrl Pts',(15.3111189513089,70.4078101425326,13.7554577359762));
#54549=CARTESIAN_POINT('Ctrl Pts',(15.3125717072818,70.4045982479306,13.7411565155594));
#54550=CARTESIAN_POINT('Ctrl Pts',(15.3168971783076,70.3957024048684,13.6980713580252));
#54551=CARTESIAN_POINT('Ctrl Pts',(15.319733590595,70.3907669208225,13.6691403883147));
#54552=CARTESIAN_POINT('Ctrl Pts',(15.3308977342618,70.3751450463372,13.5535282360151));
#54553=CARTESIAN_POINT('Ctrl Pts',(15.3389841601027,70.372406978328,13.4660143014262));
#54554=CARTESIAN_POINT('Ctrl Pts',(15.3505276621419,70.381169525788,13.3441648318202));
#54555=CARTESIAN_POINT('Ctrl Pts',(15.3538379834649,70.3850957784489,13.3095441266975));
#54556=CARTESIAN_POINT('Ctrl Pts',(15.3600645033139,70.3950361392639,13.2455279894205));
#54557=CARTESIAN_POINT('Ctrl Pts',(15.3629689659463,70.4006784071798,13.2160998363465));
#54558=CARTESIAN_POINT('Ctrl Pts',(15.368167172403,70.4124967696492,13.1644158835225));
#54559=CARTESIAN_POINT('Ctrl Pts',(15.3704467125983,70.4182495791076,13.1420766845061));
#54560=CARTESIAN_POINT('Ctrl Pts',(15.375579917579,70.4324433682094,13.0925820068369));
#54561=CARTESIAN_POINT('Ctrl Pts',(15.3784423821996,70.4411942683768,13.0655295264295));
#54562=CARTESIAN_POINT('Ctrl Pts',(15.3900456237335,70.4799307391602,12.9582186830499));
#54563=CARTESIAN_POINT('Ctrl Pts',(15.3990059087545,70.5170892740688,12.8808076629618));
#54564=CARTESIAN_POINT('Ctrl Pts',(15.4141202090388,70.5920148030536,12.7582067408705));
#54565=CARTESIAN_POINT('Ctrl Pts',(15.420225737011,70.6256506433206,12.7108012891064));
#54566=CARTESIAN_POINT('Ctrl Pts',(15.4281874274097,70.6746462290135,12.6509089046388));
#54567=CARTESIAN_POINT('Ctrl Pts',(15.4301590415946,70.6872174604953,12.6362377592349));
#54568=CARTESIAN_POINT('Ctrl Pts',(15.4334639646169,70.7090844811646,12.6118663011737));
#54569=CARTESIAN_POINT('Ctrl Pts',(15.4348076826581,70.718207123861,12.6020174942395));
#54570=CARTESIAN_POINT('Ctrl Pts',(15.4380046289984,70.7404678138127,12.5787365104635));
#54571=CARTESIAN_POINT('Ctrl Pts',(15.4398475003202,70.753750767017,12.5654478155695));
#54572=CARTESIAN_POINT('Ctrl Pts',(15.4496880002559,70.8268828966169,12.4954614202003));
#54573=CARTESIAN_POINT('Ctrl Pts',(15.4573700261058,70.8918590770472,12.4443897486525));
#54574=CARTESIAN_POINT('Ctrl Pts',(15.4694247059687,70.9999473436235,12.3752896554734));
#54575=CARTESIAN_POINT('Ctrl Pts',(15.4737400371088,71.0398609455861,12.3527167867678));
#54576=CARTESIAN_POINT('Ctrl Pts',(15.4815072719078,71.1127652144443,12.3165420581704));
#54577=CARTESIAN_POINT('Ctrl Pts',(15.4849323846649,71.1452725270213,12.3020800374201));
#54578=CARTESIAN_POINT('Ctrl Pts',(15.4907231644892,71.2004598791729,12.2802546192861));
#54579=CARTESIAN_POINT('Ctrl Pts',(15.493062773703,71.2228185879646,12.2721308302012));
#54580=CARTESIAN_POINT('Ctrl Pts',(15.497978570993,71.2698262624349,12.2565309076831));
#54581=CARTESIAN_POINT('Ctrl Pts',(15.5005572007895,71.2945006739808,12.2491673780782));
#54582=CARTESIAN_POINT('Ctrl Pts',(15.5083943330171,71.369423309474,12.2292671845683));
#54583=CARTESIAN_POINT('Ctrl Pts',(15.5137203365454,71.4202243477045,12.2190502539735));
#54584=CARTESIAN_POINT('Ctrl Pts',(15.526710103593,71.5437443460363,12.2019758560591));
#54585=CARTESIAN_POINT('Ctrl Pts',(15.5344217127366,71.6167139400239,12.1982314601836));
#54586=CARTESIAN_POINT('Ctrl Pts',(15.5447621526674,71.7154967085733,12.2016711166485));
#54587=CARTESIAN_POINT('Ctrl Pts',(15.5474596662302,71.7413667227091,12.2033657566169));
#54588=CARTESIAN_POINT('Ctrl Pts',(15.5522146077091,71.7872981001534,12.2077900800486));
#54589=CARTESIAN_POINT('Ctrl Pts',(15.5542817443091,71.8073803986679,12.2102097524672));
#54590=CARTESIAN_POINT('Ctrl Pts',(15.5576854938171,71.8407178315876,12.2150370224709));
#54591=CARTESIAN_POINT('Ctrl Pts',(15.5590344441554,71.8540063682806,12.2171773522098));
#54592=CARTESIAN_POINT('Ctrl Pts',(15.5621309792488,71.8846909747798,12.2226214639219));
#54593=CARTESIAN_POINT('Ctrl Pts',(15.5638706558884,71.9020564801243,12.2260783973999));
#54594=CARTESIAN_POINT('Ctrl Pts',(15.5742285588332,72.0058888612285,12.2490155602008));
#54595=CARTESIAN_POINT('Ctrl Pts',(15.582466671416,72.0902089971549,12.2771438233463));
#54596=CARTESIAN_POINT('Ctrl Pts',(15.5954802408073,72.2162159244106,12.3344189248631));
#54597=CARTESIAN_POINT('Ctrl Pts',(15.6001743058787,72.2602548631365,12.3576475888896));
#54598=CARTESIAN_POINT('Ctrl Pts',(15.6079872505939,72.3299841552851,12.3998350997683));
#54599=CARTESIAN_POINT('Ctrl Pts',(15.6110584837034,72.3565246267629,12.4172845775312));
#54600=CARTESIAN_POINT('Ctrl Pts',(15.6164545500316,72.4014270835153,12.4492796772511));
#54601=CARTESIAN_POINT('Ctrl Pts',(15.618761734872,72.4200929868029,12.4633731937572));
#54602=CARTESIAN_POINT('Ctrl Pts',(15.6238070466411,72.4596881563805,12.4950228273709));
#54603=CARTESIAN_POINT('Ctrl Pts',(15.6265512285425,72.4804608920149,12.5127546255014));
#54604=CARTESIAN_POINT('Ctrl Pts',(15.6348171993673,72.5406791838915,12.5676098365466));
#54605=CARTESIAN_POINT('Ctrl Pts',(15.6404106256085,72.5783336638097,12.6065964175463));
#54606=CARTESIAN_POINT('Ctrl Pts',(15.6530625299896,72.656716081412,12.6988832001763));
#54607=CARTESIAN_POINT('Ctrl Pts',(15.6601381860156,72.6959482007232,12.7532507905421));
#54608=CARTESIAN_POINT('Ctrl Pts',(15.6697529225791,72.7437124850371,12.8318492563327));
#54609=CARTESIAN_POINT('Ctrl Pts',(15.6723561459346,72.7560788184445,12.853623939215));
#54610=CARTESIAN_POINT('Ctrl Pts',(15.6769675177142,72.777034369683,12.8932040060956));
#54611=CARTESIAN_POINT('Ctrl Pts',(15.678984601826,72.7858671045772,12.9108712995588));
#54612=CARTESIAN_POINT('Ctrl Pts',(15.6823360845555,72.800010913826,12.94089307122));
#54613=CARTESIAN_POINT('Ctrl Pts',(15.6836818128242,72.8055437755759,12.9531373557262));
#54614=CARTESIAN_POINT('Ctrl Pts',(15.6868097388824,72.8180568776009,12.9820430192726));
#54615=CARTESIAN_POINT('Ctrl Pts',(15.688583219359,72.8248779306584,12.9987695847326));
#54616=CARTESIAN_POINT('Ctrl Pts',(15.6992715270306,72.8641669953806,13.1013187576491));
#54617=CARTESIAN_POINT('Ctrl Pts',(15.7077835988779,72.887617413542,13.1903203566669));
#54618=CARTESIAN_POINT('Ctrl Pts',(15.7205891076685,72.9078627850662,13.3249083827248));
#54619=CARTESIAN_POINT('Ctrl Pts',(15.7247755731598,72.9121559945579,13.3690420230747));
#54620=CARTESIAN_POINT('Ctrl Pts',(15.7321243262165,72.9155808947046,13.445687367422));
#54621=CARTESIAN_POINT('Ctrl Pts',(15.7352566549272,72.9157875237194,13.4781083081998));
#54622=CARTESIAN_POINT('Ctrl Pts',(15.7407194217992,72.9140065458678,13.5339296518394));
#54623=CARTESIAN_POINT('Ctrl Pts',(15.7430308052484,72.9126104268437,13.5573334094022));
#54624=CARTESIAN_POINT('Ctrl Pts',(15.7480440714304,72.9082182599346,13.6075381604161));
#54625=CARTESIAN_POINT('Ctrl Pts',(15.750751244167,72.9050146563437,13.634308681989));
#54626=CARTESIAN_POINT('Ctrl Pts',(15.7635593044991,72.8860222649612,13.7591872298019));
#54627=CARTESIAN_POINT('Ctrl Pts',(15.7739803759795,72.8596089083683,13.8553055344059));
#54628=CARTESIAN_POINT('Ctrl Pts',(15.7901226486762,72.8019071013486,13.9975693883632));
#54629=CARTESIAN_POINT('Ctrl Pts',(15.7958041458861,72.7783362795895,14.0464503822243));
#54630=CARTESIAN_POINT('Ctrl Pts',(15.8030951858812,72.7433755361682,14.1084651652291));
#54631=CARTESIAN_POINT('Ctrl Pts',(15.8048198843547,72.7347445475935,14.1230823900889));
#54632=CARTESIAN_POINT('Ctrl Pts',(15.8078959918652,72.7186684103895,14.1491024742073));
#54633=CARTESIAN_POINT('Ctrl Pts',(15.8092526620489,72.7113292292146,14.1605651080059));
#54634=CARTESIAN_POINT('Ctrl Pts',(15.8127696617139,72.6916695098266,14.1902099131262));
#54635=CARTESIAN_POINT('Ctrl Pts',(15.8149124090466,72.6790590824631,14.2081946325573));
#54636=CARTESIAN_POINT('Ctrl Pts',(15.8261845652096,72.609640658552,14.30192753067));
#54637=CARTESIAN_POINT('Ctrl Pts',(15.834938780409,72.544955901381,14.371480780459));
#54638=CARTESIAN_POINT('Ctrl Pts',(15.8473553903786,72.4451342709734,14.457262780635));
#54639=CARTESIAN_POINT('Ctrl Pts',(15.8508564136436,72.4161036794485,14.4800881829059));
#54640=CARTESIAN_POINT('Ctrl Pts',(15.8573817139584,72.3608632699526,14.5197520035265));
#54641=CARTESIAN_POINT('Ctrl Pts',(15.8603917794223,72.3349491295754,14.5369529481081));
#54642=CARTESIAN_POINT('Ctrl Pts',(15.8657220426888,72.288526544451,14.5653688662634));
#54643=CARTESIAN_POINT('Ctrl Pts',(15.8680259876459,72.2682903674222,14.5770014086535));
#54644=CARTESIAN_POINT('Ctrl Pts',(15.8731094775948,72.2233541058685,14.6012103032845));
#54645=CARTESIAN_POINT('Ctrl Pts',(15.8758959322651,72.1985404097865,14.6135484619975));
#54646=CARTESIAN_POINT('Ctrl Pts',(15.8881195547797,72.0890749083297,14.6635818836657));
#54647=CARTESIAN_POINT('Ctrl Pts',(15.8978248720789,72.0008601499585,14.6927533269636));
#54648=CARTESIAN_POINT('Ctrl Pts',(15.9136849533829,71.8533891361559,14.7242027223829));
#54649=CARTESIAN_POINT('Ctrl Pts',(15.9197922923734,71.7957229682606,14.73241382832));
#54650=CARTESIAN_POINT('Ctrl Pts',(15.9275069415758,71.7206197978507,14.737886008838));
#54651=CARTESIAN_POINT('Ctrl Pts',(15.929246800121,71.7035242756897,14.7387847045918));
#54652=CARTESIAN_POINT('Ctrl Pts',(15.9323352071073,71.6728402161795,14.7397761541977));
#54653=CARTESIAN_POINT('Ctrl Pts',(15.9336893449234,71.6592606999698,14.7399969953444));
#54654=CARTESIAN_POINT('Ctrl Pts',(15.9371770049191,71.6239961993076,14.7400047172771));
#54655=CARTESIAN_POINT('Ctrl Pts',(15.9392935850993,71.6023154015255,14.73945422267));
#54656=CARTESIAN_POINT('Ctrl Pts',(15.9428438068594,71.5656439317579,14.73758232507));
#54657=CARTESIAN_POINT('Ctrl Pts',(15.9442874294977,71.5506447699087,14.736549437199));
#54658=CARTESIAN_POINT('Ctrl Pts',(15.950620318836,71.4846089808678,14.7308222499309));
#54659=CARTESIAN_POINT('Ctrl Pts',(15.9554280594632,71.4338619219898,14.7233072209986));
#54660=CARTESIAN_POINT('Ctrl Pts',(15.966867913353,71.3146601021156,14.6982058486337));
#54661=CARTESIAN_POINT('Ctrl Pts',(15.9734893848709,71.2469560046675,14.6779399789805));
#54662=CARTESIAN_POINT('Ctrl Pts',(15.9830880599361,71.1541057150504,14.6414874404991));
#54663=CARTESIAN_POINT('Ctrl Pts',(15.9859226685923,71.127300108516,14.629881498222));
#54664=CARTESIAN_POINT('Ctrl Pts',(15.9910716177074,71.0798965434959,14.6073862101299));
#54665=CARTESIAN_POINT('Ctrl Pts',(15.9933736711862,71.059152485979,14.5968341608947));
#54666=CARTESIAN_POINT('Ctrl Pts',(15.9986131555517,71.0130286892704,14.5717536797824));
#54667=CARTESIAN_POINT('Ctrl Pts',(16.0015606541105,70.9878384618905,14.5569071339245));
#54668=CARTESIAN_POINT('Ctrl Pts',(16.0079535052726,70.9348981434087,14.523191253929));
#54669=CARTESIAN_POINT('Ctrl Pts',(16.0114058355853,70.9073387644444,14.5040647270978));
#54670=CARTESIAN_POINT('Ctrl Pts',(16.0229877539323,70.8182938882145,14.4368924574447));
#54671=CARTESIAN_POINT('Ctrl Pts',(16.0312357930627,70.7604807604503,14.3842766089763));
#54672=CARTESIAN_POINT('Ctrl Pts',(16.0406373207261,70.6999070861735,14.3179872322856));
#54673=CARTESIAN_POINT('Ctrl Pts',(16.041869838494,70.6920707520904,14.3091677450839));
#54674=CARTESIAN_POINT('Ctrl Pts',(16.0430985027246,70.6843589375946,14.3002409748806));
#54675=CARTESIAN_POINT('Ctrl Pts',(16.2122439422732,70.6843594233383,14.3002415371503));
#54676=CARTESIAN_POINT('Ctrl Pts',(16.2069536758919,70.7173842304241,14.3384691832336));
#54677=CARTESIAN_POINT('Ctrl Pts',(16.2016207101553,70.7526902012096,14.3747267551267));
#54678=CARTESIAN_POINT('Ctrl Pts',(16.1931820657435,70.8121650122961,14.4289109947777));
#54679=CARTESIAN_POINT('Ctrl Pts',(16.1900649309448,70.8349319996618,14.4482293885376));
#54680=CARTESIAN_POINT('Ctrl Pts',(16.1846813895207,70.8758144275889,14.4805110798706));
#54681=CARTESIAN_POINT('Ctrl Pts',(16.1824016250686,70.893629460446,14.4938339024359));
#54682=CARTESIAN_POINT('Ctrl Pts',(16.1787681662706,70.9229201699043,14.5145615872622));
#54683=CARTESIAN_POINT('Ctrl Pts',(16.1773978628202,70.9341803566216,14.5222607668843));
#54684=CARTESIAN_POINT('Ctrl Pts',(16.1743640415744,70.9596058599809,14.5390507694005));
#54685=CARTESIAN_POINT('Ctrl Pts',(16.1727063310864,70.9738317668644,14.5480442309101));
#54686=CARTESIAN_POINT('Ctrl Pts',(16.1664281650735,71.0288412626854,14.5813088201462));
#54687=CARTESIAN_POINT('Ctrl Pts',(16.1619102065471,71.0707998866339,14.6035731467499));
#54688=CARTESIAN_POINT('Ctrl Pts',(16.1508501650601,71.1771769448403,14.6525900885648));
#54689=CARTESIAN_POINT('Ctrl Pts',(16.1443641666752,71.2427313411019,14.6764866760144));
#54690=CARTESIAN_POINT('Ctrl Pts',(16.1347186985584,71.3409310256024,14.7033826840723));
#54691=CARTESIAN_POINT('Ctrl Pts',(16.1316529651547,71.3722566348716,14.7106960113178));
#54692=CARTESIAN_POINT('Ctrl Pts',(16.1258136010689,71.4317554096505,14.7222242037693));
#54693=CARTESIAN_POINT('Ctrl Pts',(16.1230487883803,71.4598583785599,14.7266954619482));
#54694=CARTESIAN_POINT('Ctrl Pts',(16.117967926395,71.5111879972875,14.7331029997539));
#54695=CARTESIAN_POINT('Ctrl Pts',(16.1156625851046,71.5343635911352,14.7353508558387));
#54696=CARTESIAN_POINT('Ctrl Pts',(16.1103865756748,71.587054319568,14.7390028893651));
#54697=CARTESIAN_POINT('Ctrl Pts',(16.1074052385265,71.6165816385375,14.7400164141687));
#54698=CARTESIAN_POINT('Ctrl Pts',(16.096514243595,71.7233954818661,14.7399563214959));
#54699=CARTESIAN_POINT('Ctrl Pts',(16.0884386510695,71.800496625268,14.7328590556421));
#54700=CARTESIAN_POINT('Ctrl Pts',(16.0736029800222,71.9391978527656,14.7071958721665));
#54701=CARTESIAN_POINT('Ctrl Pts',(16.0668825316892,72.0009784490667,14.6908752944312));
#54702=CARTESIAN_POINT('Ctrl Pts',(16.0583969433781,72.0789827105932,14.6638413676742));
#54703=CARTESIAN_POINT('Ctrl Pts',(16.056486011671,72.0965529886664,14.6573130568684));
#54704=CARTESIAN_POINT('Ctrl Pts',(16.0532419800624,72.1264484728621,14.6454456608615));
#54705=CARTESIAN_POINT('Ctrl Pts',(16.0518997015855,72.1388435905834,14.6402963792231));
#54706=CARTESIAN_POINT('Ctrl Pts',(16.0486491853745,72.1689090608831,14.6272436233034));
#54707=CARTESIAN_POINT('Ctrl Pts',(16.0467525976929,72.1864846085862,14.6191310358496));
#54708=CARTESIAN_POINT('Ctrl Pts',(16.04251232184,72.2257049395534,14.5999279883125));
#54709=CARTESIAN_POINT('Ctrl Pts',(16.0401793972825,72.2472307702321,14.5886111988781));
#54710=CARTESIAN_POINT('Ctrl Pts',(16.031910923693,72.3228748070702,14.5460264729737));
#54711=CARTESIAN_POINT('Ctrl Pts',(16.026078203658,72.374995959972,14.5113913035721));
#54712=CARTESIAN_POINT('Ctrl Pts',(16.0143505754315,72.4734894476723,14.4349028563842));
#54713=CARTESIAN_POINT('Ctrl Pts',(16.0084716325567,72.5197442915997,14.3931954999564));
#54714=CARTESIAN_POINT('Ctrl Pts',(15.9998795016945,72.5811989265552,14.3290062797088));
#54715=CARTESIAN_POINT('Ctrl Pts',(15.9972789894971,72.599031128145,14.3091655647484));
#54716=CARTESIAN_POINT('Ctrl Pts',(15.9923387811045,72.6313710283327,14.2708202725509));
#54717=CARTESIAN_POINT('Ctrl Pts',(15.9900058976087,72.6460153389615,14.2524453577068));
#54718=CARTESIAN_POINT('Ctrl Pts',(15.9843475054561,72.6799807927779,14.2073135164107));
#54719=CARTESIAN_POINT('Ctrl Pts',(15.9810042043377,72.6987837460787,14.1801906965875));
#54720=CARTESIAN_POINT('Ctrl Pts',(15.9734715810184,72.7382917441383,14.1181754634069));
#54721=CARTESIAN_POINT('Ctrl Pts',(15.9692677647825,72.7584234083624,14.0829616390773));
#54722=CARTESIAN_POINT('Ctrl Pts',(15.9575253866954,72.8094485285397,13.982880744287));
#54723=CARTESIAN_POINT('Ctrl Pts',(15.9499288974573,72.8365777569735,13.9162633524045));
#54724=CARTESIAN_POINT('Ctrl Pts',(15.9392337000661,72.8670866522122,13.8183233624603));
#54725=CARTESIAN_POINT('Ctrl Pts',(15.9360495874178,72.8751708051521,13.7886089442862));
#54726=CARTESIAN_POINT('Ctrl Pts',(15.9313815895581,72.8855829108748,13.7439929858682));
#54727=CARTESIAN_POINT('Ctrl Pts',(15.9298621260338,72.8887383173865,13.7292985076369));
#54728=CARTESIAN_POINT('Ctrl Pts',(15.9269054575026,72.8944236724162,13.7003258349149));
#54729=CARTESIAN_POINT('Ctrl Pts',(15.9254676845174,72.8969714053757,13.6860537010658));
#54730=CARTESIAN_POINT('Ctrl Pts',(15.9212586446076,72.9037675530326,13.6438136216966));
#54731=CARTESIAN_POINT('Ctrl Pts',(15.9185207440167,72.9073270648636,13.615741389039));
#54732=CARTESIAN_POINT('Ctrl Pts',(15.9116099942222,72.9140046563963,13.5439194899895));
#54733=CARTESIAN_POINT('Ctrl Pts',(15.9074798185523,72.9158005284265,13.5000838619579));
#54734=CARTESIAN_POINT('Ctrl Pts',(15.8955138427457,72.914421096906,13.3727779359948));
#54735=CARTESIAN_POINT('Ctrl Pts',(15.8877198970543,72.9052916300286,13.2896187949757));
#54736=CARTESIAN_POINT('Ctrl Pts',(15.876924827781,72.8821678164368,13.1799577962869));
#54737=CARTESIAN_POINT('Ctrl Pts',(15.8741443679683,72.8753182796234,13.1521638116845));
#54738=CARTESIAN_POINT('Ctrl Pts',(15.8690486463106,72.8612067654419,13.1022287846414));
#54739=CARTESIAN_POINT('Ctrl Pts',(15.8667444498011,72.8542630004628,13.0800104784567));
#54740=CARTESIAN_POINT('Ctrl Pts',(15.8614387727845,72.8370282514575,13.0297575796099));
#54741=CARTESIAN_POINT('Ctrl Pts',(15.8584259556878,72.826351520773,13.0018713737063));
#54742=CARTESIAN_POINT('Ctrl Pts',(15.8518498003061,72.8011824038681,12.9424893326376));
#54743=CARTESIAN_POINT('Ctrl Pts',(15.8482784182537,72.7863630186745,12.9111589108167));
#54744=CARTESIAN_POINT('Ctrl Pts',(15.8357440536633,72.7304007268286,12.8043759948167));
#54745=CARTESIAN_POINT('Ctrl Pts',(15.8266382249414,72.6829025171005,12.7325253309429));
#54746=CARTESIAN_POINT('Ctrl Pts',(15.8144982442271,72.6091601381511,12.6423518862821));
#54747=CARTESIAN_POINT('Ctrl Pts',(15.811336815638,72.5889517742661,12.61938522073));
#54748=CARTESIAN_POINT('Ctrl Pts',(15.8067116875847,72.5577346553901,12.5863905802694));
#54749=CARTESIAN_POINT('Ctrl Pts',(15.8052123499448,72.5473488152746,12.5757916679543));
#54750=CARTESIAN_POINT('Ctrl Pts',(15.8022596002214,72.5263344873181,12.5550850193422));
#54751=CARTESIAN_POINT('Ctrl Pts',(15.8008061580451,72.5157119719336,12.5449745222973));
#54752=CARTESIAN_POINT('Ctrl Pts',(15.7964740187286,72.4832732991461,12.5151531012146));
#54753=CARTESIAN_POINT('Ctrl Pts',(15.7936318032601,72.4609436491529,12.4960116745226));
#54754=CARTESIAN_POINT('Ctrl Pts',(15.7863309763494,72.4013272670519,12.4483969576202));
#54755=CARTESIAN_POINT('Ctrl Pts',(15.7819214878312,72.3630918888059,12.4211826119618));
#54756=CARTESIAN_POINT('Ctrl Pts',(15.7702293480454,72.2578480723481,12.3547313890348));
#54757=CARTESIAN_POINT('Ctrl Pts',(15.7629705486992,72.1886124456067,12.3194197956234));
#54758=CARTESIAN_POINT('Ctrl Pts',(15.7527109809555,72.089632020526,12.2798735726927));
#54759=CARTESIAN_POINT('Ctrl Pts',(15.7498921373544,72.0623110116881,12.2700300404668));
#54760=CARTESIAN_POINT('Ctrl Pts',(15.7447592194768,72.0125317692914,12.254000150787));
#54761=CARTESIAN_POINT('Ctrl Pts',(15.7424570827514,71.9901945073682,12.247478858865));
#54762=CARTESIAN_POINT('Ctrl Pts',(15.7372008795558,71.9392595700194,12.2341154449411));
#54763=CARTESIAN_POINT('Ctrl Pts',(15.7342364096056,71.9105793352779,12.2276459266755));
#54764=CARTESIAN_POINT('Ctrl Pts',(15.727795894836,71.8484684323509,12.215883823091));
#54765=CARTESIAN_POINT('Ctrl Pts',(15.7243125973126,71.8149989349126,12.2109210085884));
#54766=CARTESIAN_POINT('Ctrl Pts',(15.7124938778567,71.7018717016388,12.1987388322188));
#54767=CARTESIAN_POINT('Ctrl Pts',(15.704034031141,71.6217408758815,12.1977058039898));
#54768=CARTESIAN_POINT('Ctrl Pts',(15.6920231010298,71.507286949311,12.2070504313153));
#54769=CARTESIAN_POINT('Ctrl Pts',(15.6884002605089,71.4726469703922,12.2113206116902));
#54770=CARTESIAN_POINT('Ctrl Pts',(15.6831916643632,71.4223621283758,12.2196350330034));
#54771=CARTESIAN_POINT('Ctrl Pts',(15.6815613857106,71.4065510959083,12.2225587240702));
#54772=CARTESIAN_POINT('Ctrl Pts',(15.6785537789849,71.3772018334364,12.2285643984775));
#54773=CARTESIAN_POINT('Ctrl Pts',(15.6771732832589,71.3636523235524,12.2315691810899));
#54774=CARTESIAN_POINT('Ctrl Pts',(15.6734255340765,71.3267125564333,12.2403987821823));
#54775=CARTESIAN_POINT('Ctrl Pts',(15.6710809334944,71.3034337737362,12.2466683992065));
#54776=CARTESIAN_POINT('Ctrl Pts',(15.6619757980103,71.2128953905287,12.2738399089759));
#54777=CARTESIAN_POINT('Ctrl Pts',(15.6553982928698,71.1472379037731,12.2996598077427));
#54778=CARTESIAN_POINT('Ctrl Pts',(15.6428589077792,71.0275115229793,12.358655297591));
#54779=CARTESIAN_POINT('Ctrl Pts',(15.6369227566369,70.9731292604227,12.3906836947697));
#54780=CARTESIAN_POINT('Ctrl Pts',(15.6280770332459,70.8976512919767,12.4430607623033));
#54781=CARTESIAN_POINT('Ctrl Pts',(15.6252752727666,70.8745187034793,12.4603099216606));
#54782=CARTESIAN_POINT('Ctrl Pts',(15.6201590351721,70.8338252883133,12.4928674735473));
#54783=CARTESIAN_POINT('Ctrl Pts',(15.6178561081095,70.8160597266575,12.5079002020276));
#54784=CARTESIAN_POINT('Ctrl Pts',(15.6125786702471,70.7766613346707,12.5431403092564));
#54785=CARTESIAN_POINT('Ctrl Pts',(15.6095933534295,70.7553029696858,12.5636321565306));
#54786=CARTESIAN_POINT('Ctrl Pts',(15.603094464543,70.7108599706198,12.6093588770371));
#54787=CARTESIAN_POINT('Ctrl Pts',(15.5995733028404,70.6880399560309,12.6348176994625));
#54788=CARTESIAN_POINT('Ctrl Pts',(15.5874557765618,70.6137731297783,12.7247201212873));
#54789=CARTESIAN_POINT('Ctrl Pts',(15.5787272068727,70.5675845670795,12.7932368813912));
#54790=CARTESIAN_POINT('Ctrl Pts',(15.5667196782044,70.5128855554526,12.8943529511359));
#54791=CARTESIAN_POINT('Ctrl Pts',(15.5633465106992,70.4985091748802,12.923556565982));
#54792=CARTESIAN_POINT('Ctrl Pts',(15.5584194238919,70.4788742384884,12.9676408893398));
#54793=CARTESIAN_POINT('Ctrl Pts',(15.5568270297503,70.4727460091658,12.982117089778));
#54794=CARTESIAN_POINT('Ctrl Pts',(15.5538413186338,70.4616540380434,13.0097362582877));
#54795=CARTESIAN_POINT('Ctrl Pts',(15.5524457112825,70.456637105262,13.0228534524509));
#54796=CARTESIAN_POINT('Ctrl Pts',(15.5485710456865,70.4432076268704,13.0597909325706));
#54797=CARTESIAN_POINT('Ctrl Pts',(15.5461174907474,70.4352861821186,13.0837839645116));
#54798=CARTESIAN_POINT('Ctrl Pts',(15.5367756251387,70.4075969807519,13.176895814171));
#54799=CARTESIAN_POINT('Ctrl Pts',(15.5300703702451,70.3929925450788,13.2474144590393));
#54800=CARTESIAN_POINT('Ctrl Pts',(15.5176505444871,70.377259326907,13.3786227701155));
#54801=CARTESIAN_POINT('Ctrl Pts',(15.5119681015055,70.3743530396791,13.438875722459));
#54802=CARTESIAN_POINT('Ctrl Pts',(15.5034086926108,70.3763893068207,13.5277146557221));
#54803=CARTESIAN_POINT('Ctrl Pts',(15.5006282171801,70.3780120894559,13.5562943250599));
#54804=CARTESIAN_POINT('Ctrl Pts',(15.4955324715968,70.3827023879678,13.6079728310771));
#54805=CARTESIAN_POINT('Ctrl Pts',(15.4932282669454,70.3854429042861,13.6310891106407));
#54806=CARTESIAN_POINT('Ctrl Pts',(15.4879225741783,70.3931447677185,13.6836541974094));
#54807=CARTESIAN_POINT('Ctrl Pts',(15.4849097495037,70.3985125680241,13.7130280675454));
#54808=CARTESIAN_POINT('Ctrl Pts',(15.4783335782917,70.4123351546843,13.7760254271594));
#54809=CARTESIAN_POINT('Ctrl Pts',(15.4747621879987,70.4211417787942,13.8095464420371));
#54810=CARTESIAN_POINT('Ctrl Pts',(15.462227782131,70.4565179797245,13.9247982961317));
#54811=CARTESIAN_POINT('Ctrl Pts',(15.4531219198104,70.4899967856893,14.0041571189042));
#54812=CARTESIAN_POINT('Ctrl Pts',(15.4409819341652,70.5459036781837,14.1063511827171));
#54813=CARTESIAN_POINT('Ctrl Pts',(15.4378205312029,70.5615449875661,14.1326414949653));
#54814=CARTESIAN_POINT('Ctrl Pts',(15.4331954302685,70.586163708468,14.170812819673));
#54815=CARTESIAN_POINT('Ctrl Pts',(15.4316960947869,70.5944238694899,14.183140504408));
#54816=CARTESIAN_POINT('Ctrl Pts',(15.4287433527419,70.6112729861074,14.2073576543103));
#54817=CARTESIAN_POINT('Ctrl Pts',(15.4272899160967,70.6198555624758,14.2192487357362));
#54818=CARTESIAN_POINT('Ctrl Pts',(15.4229577860276,70.6462585003573,14.2545256703274));
#54819=CARTESIAN_POINT('Ctrl Pts',(15.4201155744588,70.6646883045403,14.2774461408655));
#54820=CARTESIAN_POINT('Ctrl Pts',(15.4172793358864,70.6840526097242,14.299886287465));
#54821=CARTESIAN_POINT('Ctrl Pts',(15.4172569145787,70.684205752265,14.3000636560126));
#54822=CARTESIAN_POINT('Ctrl Pts',(15.4172344952204,70.6843589433712,14.3002409815672));
#54823=CARTESIAN_POINT('Origin',(21.26284859951,71.6454,13.47));
#54824=CARTESIAN_POINT('',(14.4555370852546,70.6843589127286,14.3002409460971));
#54825=CARTESIAN_POINT('',(14.625502981677,70.6843589433681,14.3002409815636));
#54826=CARTESIAN_POINT('',(21.26284859951,70.6843589433668,14.3002409815622));
#54827=CARTESIAN_POINT('',(15.1394311199487,71.6444811469566,14.7399994594157));
#54828=CARTESIAN_POINT('Ctrl Pts',(14.4555370852546,70.6843589127286,14.3002409460971));
#54829=CARTESIAN_POINT('Ctrl Pts',(14.4623859954626,70.6371020472158,14.2455390073082));
#54830=CARTESIAN_POINT('Ctrl Pts',(14.4691094373412,70.5945863966558,14.1868844469984));
#54831=CARTESIAN_POINT('Ctrl Pts',(14.4791850657878,70.5396106440812,14.0955433899042));
#54832=CARTESIAN_POINT('Ctrl Pts',(14.4824433690888,70.5231342982942,14.0654779376296));
#54833=CARTESIAN_POINT('Ctrl Pts',(14.4885836748825,70.4947294907501,14.0082692683133));
#54834=CARTESIAN_POINT('Ctrl Pts',(14.491454478698,70.4824964662219,13.981303701591));
#54835=CARTESIAN_POINT('Ctrl Pts',(14.4966272647768,70.4623951160937,13.9325316271323));
#54836=CARTESIAN_POINT('Ctrl Pts',(14.4989158873162,70.4541603647051,13.9108900299642));
#54837=CARTESIAN_POINT('Ctrl Pts',(14.5040674383531,70.4371152865573,13.8621235595589));
#54838=CARTESIAN_POINT('Ctrl Pts',(14.5069392300526,70.428618261718,13.8349036962588));
#54839=CARTESIAN_POINT('Ctrl Pts',(14.5196627816136,70.395393565045,13.7143465831408));
#54840=CARTESIAN_POINT('Ctrl Pts',(14.5298064666729,70.3804448576273,13.618666643329));
#54841=CARTESIAN_POINT('Ctrl Pts',(14.5454537646757,70.3743247183194,13.4700151286904));
#54842=CARTESIAN_POINT('Ctrl Pts',(14.5509313223629,70.3754007001904,13.4176973733095));
#54843=CARTESIAN_POINT('Ctrl Pts',(14.5580345509482,70.3811000639259,13.3486081815444));
#54844=CARTESIAN_POINT('Ctrl Pts',(14.5597667491123,70.3828425463694,13.3316559140685));
#54845=CARTESIAN_POINT('Ctrl Pts',(14.5628437800497,70.3865813785695,13.3013018515283));
#54846=CARTESIAN_POINT('Ctrl Pts',(14.5641941507816,70.388451646137,13.287889425704));
#54847=CARTESIAN_POINT('Ctrl Pts',(14.5676665389007,70.3938554964315,13.2532022095279));
#54848=CARTESIAN_POINT('Ctrl Pts',(14.5697718242952,70.3977169838792,13.2319827395152));
#54849=CARTESIAN_POINT('Ctrl Pts',(14.5789568529845,70.4170965148864,13.139001595652));
#54850=CARTESIAN_POINT('Ctrl Pts',(14.5858149806443,70.4382810627897,13.0685571753205));
#54851=CARTESIAN_POINT('Ctrl Pts',(14.5987647869399,70.489264576998,12.9404702473549));
#54852=CARTESIAN_POINT('Ctrl Pts',(14.6048281180988,70.5176084360242,12.8825177248292));
#54853=CARTESIAN_POINT('Ctrl Pts',(14.6138195994487,70.5648991836087,12.8019744274072));
#54854=CARTESIAN_POINT('Ctrl Pts',(14.6166341133883,70.5804253819109,12.7774908386727));
#54855=CARTESIAN_POINT('Ctrl Pts',(14.6217672516889,70.6099251429435,12.7343130504535));
#54856=CARTESIAN_POINT('Ctrl Pts',(14.6240741211823,70.6236026045024,12.7154316647374));
#54857=CARTESIAN_POINT('Ctrl Pts',(14.6293539044472,70.6557964403548,12.6734701664474));
#54858=CARTESIAN_POINT('Ctrl Pts',(14.632337502544,70.6746145473083,12.6506403578733));
#54859=CARTESIAN_POINT('Ctrl Pts',(14.6388303449703,70.7168336807592,12.6029185013257));
#54860=CARTESIAN_POINT('Ctrl Pts',(14.6423471070369,70.7404764771294,12.5782720847042));
#54861=CARTESIAN_POINT('Ctrl Pts',(14.6544366052751,70.8243509191185,12.4976110567644));
#54862=CARTESIAN_POINT('Ctrl Pts',(14.663140400138,70.8890154553614,12.4465047058285));
#54863=CARTESIAN_POINT('Ctrl Pts',(14.6751219747651,70.9855045620111,12.3844146510052));
#54864=CARTESIAN_POINT('Ctrl Pts',(14.6784929690035,71.0135207757879,12.3678717488517));
#54865=CARTESIAN_POINT('Ctrl Pts',(14.6834195067839,71.0559896318912,12.3449475739994));
#54866=CARTESIAN_POINT('Ctrl Pts',(14.6850133449625,71.0699737924309,12.3377313432969));
#54867=CARTESIAN_POINT('Ctrl Pts',(14.688004649971,71.0967255854598,12.3245503875933));
#54868=CARTESIAN_POINT('Ctrl Pts',(14.6894043515429,71.1094638380836,12.3185353245126));
#54869=CARTESIAN_POINT('Ctrl Pts',(14.6933023674832,71.1454990476914,12.3022469747278));
#54870=CARTESIAN_POINT('Ctrl Pts',(14.6957747299264,71.169009672123,12.2924599163341));
#54871=CARTESIAN_POINT('Ctrl Pts',(14.705389226784,71.2624437855811,12.2568222720668));
#54872=CARTESIAN_POINT('Ctrl Pts',(14.7123344283293,71.334297335484,12.2364387673053));
#54873=CARTESIAN_POINT('Ctrl Pts',(14.7252861341219,71.4695970539378,12.2106408197926));
#54874=CARTESIAN_POINT('Ctrl Pts',(14.7312551922974,71.5324508028325,12.2034563342344));
#54875=CARTESIAN_POINT('Ctrl Pts',(14.7399439019398,71.6222436711666,12.1999306001911));
#54876=CARTESIAN_POINT('Ctrl Pts',(14.7425464224137,71.6489396660501,12.1997245494217));
#54877=CARTESIAN_POINT('Ctrl Pts',(14.7474900203272,71.6991209173944,12.2009189688201));
#54878=CARTESIAN_POINT('Ctrl Pts',(14.7498242687672,71.7225995988123,12.2021306695582));
#54879=CARTESIAN_POINT('Ctrl Pts',(14.7554856085747,71.7789348195803,12.2066085052873));
#54880=CARTESIAN_POINT('Ctrl Pts',(14.7588304984984,71.8117218740769,12.2105055957614));
#54881=CARTESIAN_POINT('Ctrl Pts',(14.7663664006841,71.8843745344286,12.2220271704995));
#54882=CARTESIAN_POINT('Ctrl Pts',(14.7705719091205,71.9241007175369,12.2302943078007));
#54883=CARTESIAN_POINT('Ctrl Pts',(14.7823181606159,72.0328925240294,12.2584275713604));
#54884=CARTESIAN_POINT('Ctrl Pts',(14.7899168574425,72.1007733730978,12.2822739837804));
#54885=CARTESIAN_POINT('Ctrl Pts',(14.8006174980588,72.1943734917263,12.3243659614619));
#54886=CARTESIAN_POINT('Ctrl Pts',(14.8038047871038,72.2220071058663,12.3380221101555));
#54887=CARTESIAN_POINT('Ctrl Pts',(14.8084766631513,72.2623464789848,12.3598184524329));
#54888=CARTESIAN_POINT('Ctrl Pts',(14.8099969046158,72.275446563061,12.3672001841706));
#54889=CARTESIAN_POINT('Ctrl Pts',(14.8129535390303,72.30090674186,12.3821485423193));
#54890=CARTESIAN_POINT('Ctrl Pts',(14.8143905197065,72.3132743516951,12.3896973607616));
#54891=CARTESIAN_POINT('Ctrl Pts',(14.8185950123231,72.349365970552,12.4125834350591));
#54892=CARTESIAN_POINT('Ctrl Pts',(14.8213292413831,72.3727126730733,12.428503696659));
#54893=CARTESIAN_POINT('Ctrl Pts',(14.8282269812653,72.4308072017112,12.4710261585479));
#54894=CARTESIAN_POINT('Ctrl Pts',(14.832347991805,72.4647477257508,12.4986693730336));
#54895=CARTESIAN_POINT('Ctrl Pts',(14.8443238389772,72.559257798012,12.5841304456661));
#54896=CARTESIAN_POINT('Ctrl Pts',(14.8521360561802,72.6156139081804,12.6462381828907));
#54897=CARTESIAN_POINT('Ctrl Pts',(14.8629486455118,72.6824861333793,12.7363992199886));
#54898=CARTESIAN_POINT('Ctrl Pts',(14.8657268142804,72.6987394144301,12.759934132309));
#54899=CARTESIAN_POINT('Ctrl Pts',(14.8708193040879,72.7267508801369,12.8035755116529));
#54900=CARTESIAN_POINT('Ctrl Pts',(14.8731225895676,72.738776961114,12.8234955771858));
#54901=CARTESIAN_POINT('Ctrl Pts',(14.8784270980967,72.7649688135127,12.8697027490863));
#54902=CARTESIAN_POINT('Ctrl Pts',(14.8814396754385,72.7787674898374,12.8961804488411));
#54903=CARTESIAN_POINT('Ctrl Pts',(14.8880155927676,72.8065390222253,12.9543871652908));
#54904=CARTESIAN_POINT('Ctrl Pts',(14.8915869870584,72.8201711365309,12.9862514037533));
#54905=CARTESIAN_POINT('Ctrl Pts',(14.9041216913923,72.8630187619736,13.0989386431305));
#54906=CARTESIAN_POINT('Ctrl Pts',(14.9132279746881,72.8853243854313,13.1821320421558));
#54907=CARTESIAN_POINT('Ctrl Pts',(14.9253711114549,72.90395367473,13.2971442475199));
#54908=CARTESIAN_POINT('Ctrl Pts',(14.9285351549297,72.907753836088,13.327522961839));
#54909=CARTESIAN_POINT('Ctrl Pts',(14.933162831648,72.9117611847237,13.372791591261));
#54910=CARTESIAN_POINT('Ctrl Pts',(14.9346621914832,72.9128104976783,13.3875934970797));
#54911=CARTESIAN_POINT('Ctrl Pts',(14.9376146228393,72.9143803639284,13.4170498272747));
#54912=CARTESIAN_POINT('Ctrl Pts',(14.9390677357706,72.9149070651269,13.43170160893));
#54913=CARTESIAN_POINT('Ctrl Pts',(14.9433957740632,72.9157264578889,13.4757145920993));
#54914=CARTESIAN_POINT('Ctrl Pts',(14.9462343331721,72.9152549560158,13.5050826407288));
#54915=CARTESIAN_POINT('Ctrl Pts',(14.953520749945,72.9113931473839,13.5811278212527));
#54916=CARTESIAN_POINT('Ctrl Pts',(14.9579197400882,72.9064413720226,13.6276814781811));
#54917=CARTESIAN_POINT('Ctrl Pts',(14.9696215869441,72.8864458116629,13.7506342367532));
#54918=CARTESIAN_POINT('Ctrl Pts',(14.9769000523872,72.8669349702154,13.8260904959691));
#54919=CARTESIAN_POINT('Ctrl Pts',(14.9871802758568,72.8308345331101,13.9266045876419));
#54920=CARTESIAN_POINT('Ctrl Pts',(14.9899988142451,72.8200886645546,13.9535793809008));
#54921=CARTESIAN_POINT('Ctrl Pts',(14.9951324792282,72.7990784358473,14.0014771110744));
#54922=CARTESIAN_POINT('Ctrl Pts',(14.9974356938212,72.7891442484205,14.022531239347));
#54923=CARTESIAN_POINT('Ctrl Pts',(15.0026964721551,72.7653530654631,14.0695591918255));
#54924=CARTESIAN_POINT('Ctrl Pts',(15.005664488695,72.7511608225082,14.0953468946793));
#54925=CARTESIAN_POINT('Ctrl Pts',(15.0121144821189,72.7187296772208,14.1497142051035));
#54926=CARTESIAN_POINT('Ctrl Pts',(15.0156037572945,72.7002164094905,14.1781030073912));
#54927=CARTESIAN_POINT('Ctrl Pts',(15.0274681411383,72.6340506589288,14.2712019345502));
#54928=CARTESIAN_POINT('Ctrl Pts',(15.0359687842437,72.5814012425502,14.3321221581525));
#54929=CARTESIAN_POINT('Ctrl Pts',(15.0479739647793,72.4984452249864,14.4114895455686));
#54930=CARTESIAN_POINT('Ctrl Pts',(15.0515536626689,72.4725694811561,14.4343028249508));
#54931=CARTESIAN_POINT('Ctrl Pts',(15.0567150271168,72.4333506005646,14.4661379036494));
#54932=CARTESIAN_POINT('Ctrl Pts',(15.0583400993012,72.4207157184319,14.4760032311401));
#54933=CARTESIAN_POINT('Ctrl Pts',(15.0613454038267,72.3967737347498,14.4939780040941));
#54934=CARTESIAN_POINT('Ctrl Pts',(15.0627286679121,72.385515204214,14.5021448367948));
#54935=CARTESIAN_POINT('Ctrl Pts',(15.0664975443531,72.3542292074216,14.5240641309082));
#54936=CARTESIAN_POINT('Ctrl Pts',(15.0688600499269,72.3339371394535,14.5374300511625));
#54937=CARTESIAN_POINT('Ctrl Pts',(15.0779950954556,72.253250337638,14.5873171930225));
#54938=CARTESIAN_POINT('Ctrl Pts',(15.0845851450513,72.190232864405,14.6193647444231));
#54939=CARTESIAN_POINT('Ctrl Pts',(15.0976326765066,72.0616363800101,14.6717947938584));
#54940=CARTESIAN_POINT('Ctrl Pts',(15.1040669574391,71.9964332881293,14.6924307606925));
#54941=CARTESIAN_POINT('Ctrl Pts',(15.1132679287311,71.9036371587971,14.7137602009614));
#54942=CARTESIAN_POINT('Ctrl Pts',(15.115893303152,71.8771969504096,14.7189578812514));
#54943=CARTESIAN_POINT('Ctrl Pts',(15.1207903773722,71.8281046082427,14.7269961290577));
#54944=CARTESIAN_POINT('Ctrl Pts',(15.123053648869,71.8055022330863,14.7300743429641));
#54945=CARTESIAN_POINT('Ctrl Pts',(15.1274646543716,71.7616870260599,14.7348437423548));
#54946=CARTESIAN_POINT('Ctrl Pts',(15.1296091768705,71.7404902318351,14.7366136258512));
#54947=CARTESIAN_POINT('Ctrl Pts',(15.1343033818943,71.6943578204931,14.739301139189));
#54948=CARTESIAN_POINT('Ctrl Pts',(15.1368579689929,71.669420131619,14.7400177389146));
#54949=CARTESIAN_POINT('Ctrl Pts',(15.1394309042231,71.6444797315774,14.7399996665771));
#54950=CARTESIAN_POINT('Ctrl Pts',(15.1394307620321,71.6444811098864,14.7399996675751));
#54951=CARTESIAN_POINT('Ctrl Pts',(15.1509210808744,71.533101228028,14.739919080253));
#54952=CARTESIAN_POINT('Ctrl Pts',(15.1627791610613,71.4222292170545,14.7251882517743));
#54953=CARTESIAN_POINT('Ctrl Pts',(15.1768284770286,71.2913020977506,14.6898779156159));
#54954=CARTESIAN_POINT('Ctrl Pts',(15.1793190930862,71.2680836105176,14.6828973793084));
#54955=CARTESIAN_POINT('Ctrl Pts',(15.1831877343141,71.2318876403853,14.6708749610823));
#54956=CARTESIAN_POINT('Ctrl Pts',(15.1845866594627,71.218769932039,14.666277569344));
#54957=CARTESIAN_POINT('Ctrl Pts',(15.1875722086513,71.190685709647,14.65591400007));
#54958=CARTESIAN_POINT('Ctrl Pts',(15.1891550046976,71.1757479795498,14.6500780374656));
#54959=CARTESIAN_POINT('Ctrl Pts',(15.1944197183191,71.1260255163516,14.6295582891983));
#54960=CARTESIAN_POINT('Ctrl Pts',(15.1980392416794,71.0917821032234,14.613605397761));
#54961=CARTESIAN_POINT('Ctrl Pts',(15.2090248745081,70.9891787709298,14.5601143564284));
#54962=CARTESIAN_POINT('Ctrl Pts',(15.2162629792696,70.9235239537745,14.5177936068783));
#54963=CARTESIAN_POINT('Ctrl Pts',(15.2268090935942,70.8357704161096,14.4490423742027));
#54964=CARTESIAN_POINT('Ctrl Pts',(15.2300000230711,70.8102101963678,14.4273305006902));
#54965=CARTESIAN_POINT('Ctrl Pts',(15.2360380432644,70.7640304866041,14.3848453839361));
#54966=CARTESIAN_POINT('Ctrl Pts',(15.2388748568639,70.7432120586773,14.3643214764988));
#54967=CARTESIAN_POINT('Ctrl Pts',(15.2436330533099,70.7098761913435,14.3291079197914));
#54968=CARTESIAN_POINT('Ctrl Pts',(15.2455362747428,70.6969519753471,14.3148179791374));
#54969=CARTESIAN_POINT('Ctrl Pts',(15.2474530402596,70.6843589428744,14.3002409809922));
#54970=CARTESIAN_POINT('',(15.3085945258992,71.645458134439,14.7400003205931));
#54971=CARTESIAN_POINT('Ctrl Pts',(15.4172344952204,70.6843589433712,14.3002409815672));
#54972=CARTESIAN_POINT('Ctrl Pts',(15.4127706930735,70.7148600299651,14.3355473530177));
#54973=CARTESIAN_POINT('Ctrl Pts',(15.4083832547445,70.7472863263589,14.3691492972001));
#54974=CARTESIAN_POINT('Ctrl Pts',(15.3967131226841,70.8383472626173,14.4536577777352));
#54975=CARTESIAN_POINT('Ctrl Pts',(15.3894543105498,70.8999107323482,14.5010966726018));
#54976=CARTESIAN_POINT('Ctrl Pts',(15.3791947372806,70.98993336973,14.5581665738801));
#54977=CARTESIAN_POINT('Ctrl Pts',(15.3763759031919,71.0149788345287,14.5728652884407));
#54978=CARTESIAN_POINT('Ctrl Pts',(15.371243010044,71.0609622006778,14.5977738342165));
#54979=CARTESIAN_POINT('Ctrl Pts',(15.3689408886463,71.0817196132603,14.6082906516138));
#54980=CARTESIAN_POINT('Ctrl Pts',(15.3636847355834,71.1293289710434,14.6307905726155));
#54981=CARTESIAN_POINT('Ctrl Pts',(15.3607203007963,71.1563305661364,14.6424226167686));
#54982=CARTESIAN_POINT('Ctrl Pts',(15.354279875988,71.2152194070113,14.6654031936946));
#54983=CARTESIAN_POINT('Ctrl Pts',(15.3507966335996,71.2472054438283,14.6764347331971));
#54984=CARTESIAN_POINT('Ctrl Pts',(15.3393010133244,71.3531858267669,14.7083122361119));
#54985=CARTESIAN_POINT('Ctrl Pts',(15.331176493587,71.4286354225623,14.7237215690252));
#54986=CARTESIAN_POINT('Ctrl Pts',(15.3198877989525,71.5357798711219,14.7356390330013));
#54987=CARTESIAN_POINT('Ctrl Pts',(15.3166634990233,71.5666714167958,14.7379356869999));
#54988=CARTESIAN_POINT('Ctrl Pts',(15.3118384439432,71.6135569828337,14.7397009132116));
#54989=CARTESIAN_POINT('Ctrl Pts',(15.3102091325305,71.6295062635558,14.7400007281653));
#54990=CARTESIAN_POINT('Ctrl Pts',(15.3085939729866,71.6454580784378,14.739999998672));
#54991=CARTESIAN_POINT('Ctrl Pts',(14.625502981677,70.6843589433682,14.3002409815638));
#54992=CARTESIAN_POINT('Ctrl Pts',(14.6281650357797,70.6666703255623,14.2797656155869));
#54993=CARTESIAN_POINT('Ctrl Pts',(14.6308005194417,70.6496391110251,14.2587284948775));
#54994=CARTESIAN_POINT('Ctrl Pts',(14.6411179044699,70.5851039435374,14.1735878753866));
#54995=CARTESIAN_POINT('Ctrl Pts',(14.648593760091,70.5430096721227,14.1056113942086));
#54996=CARTESIAN_POINT('Ctrl Pts',(14.6625924101878,70.4767980028742,13.9720636382048));
#54997=CARTESIAN_POINT('Ctrl Pts',(14.6690915769207,70.4511624437155,13.9075979717112));
#54998=CARTESIAN_POINT('Ctrl Pts',(14.6774573056598,70.426010423835,13.8253450487112));
#54999=CARTESIAN_POINT('Ctrl Pts',(14.6791009835702,70.4214265022496,13.8092194279602));
#55000=CARTESIAN_POINT('Ctrl Pts',(14.6820939757825,70.4137425546004,13.7800013626373));
#55001=CARTESIAN_POINT('Ctrl Pts',(14.6834373704991,70.4105290649238,13.7669421350229));
#55002=CARTESIAN_POINT('Ctrl Pts',(14.686612591975,70.4034860000019,13.7362254274108));
#55003=CARTESIAN_POINT('Ctrl Pts',(14.6884521353256,70.3998250761717,13.7185343971115));
#55004=CARTESIAN_POINT('Ctrl Pts',(14.6967219037202,70.3851863146071,13.6393149227284));
#55005=CARTESIAN_POINT('Ctrl Pts',(14.7032974414655,70.3783830775501,13.5771093715393));
#55006=CARTESIAN_POINT('Ctrl Pts',(14.7186402538576,70.3732534566918,13.4313400215769));
#55007=CARTESIAN_POINT('Ctrl Pts',(14.7273599950559,70.3785330673784,13.3479132534191));
#55008=CARTESIAN_POINT('Ctrl Pts',(14.7387587019873,70.3965651282886,13.237339522462));
#55009=CARTESIAN_POINT('Ctrl Pts',(14.7416426692286,70.4021268058687,13.2092481444338));
#55010=CARTESIAN_POINT('Ctrl Pts',(14.7468190743007,70.4139241861666,13.1586976489804));
#55011=CARTESIAN_POINT('Ctrl Pts',(14.7491203423951,70.4198370640752,13.1361774421891));
#55012=CARTESIAN_POINT('Ctrl Pts',(14.7543305600558,70.4347384645587,13.0851755539095));
#55013=CARTESIAN_POINT('Ctrl Pts',(14.7572258578014,70.4441191849167,13.0568221458506));
#55014=CARTESIAN_POINT('Ctrl Pts',(14.7634268590528,70.4665278387567,12.9963324610459));
#55015=CARTESIAN_POINT('Ctrl Pts',(14.766721030978,70.4798894970243,12.9643458324319));
#55016=CARTESIAN_POINT('Ctrl Pts',(14.7781217399889,70.5309020910025,12.8550311987522));
#55017=CARTESIAN_POINT('Ctrl Pts',(14.7860860949509,70.5750749040709,12.7810194578937));
#55018=CARTESIAN_POINT('Ctrl Pts',(14.7972187739038,70.6445886321964,12.6875631584461));
#55019=CARTESIAN_POINT('Ctrl Pts',(14.8001643096785,70.6636708562699,12.663750525638));
#55020=CARTESIAN_POINT('Ctrl Pts',(14.80461855296,70.6932741349911,12.6294190745434));
#55021=CARTESIAN_POINT('Ctrl Pts',(14.8060876079797,70.703154313686,12.6183586759229));
#55022=CARTESIAN_POINT('Ctrl Pts',(14.8090396473062,70.7231955128251,12.5966991301657));
#55023=CARTESIAN_POINT('Ctrl Pts',(14.8105221701063,70.7333512188006,12.5860981572875));
#55024=CARTESIAN_POINT('Ctrl Pts',(14.8150187030111,70.7644645464167,12.554727763174));
#55025=CARTESIAN_POINT('Ctrl Pts',(14.8180656787368,70.7859630046302,12.5345117963949));
#55026=CARTESIAN_POINT('Ctrl Pts',(14.8260499202662,70.8436170630015,12.483962527035));
#55027=CARTESIAN_POINT('Ctrl Pts',(14.8310188368833,70.8807949535119,12.4548623300102));
#55028=CARTESIAN_POINT('Ctrl Pts',(14.8440812699463,70.9827214779599,12.3838633423603));
#55029=CARTESIAN_POINT('Ctrl Pts',(14.8521258926325,71.0498271705976,12.345663234386));
#55030=CARTESIAN_POINT('Ctrl Pts',(14.8629319742427,71.1464456942483,12.3017582754833));
#55031=CARTESIAN_POINT('Ctrl Pts',(14.86586109953,71.1733038414498,12.2906486153169));
#55032=CARTESIAN_POINT('Ctrl Pts',(14.8710817197662,71.222312132462,12.2723198003389));
#55033=CARTESIAN_POINT('Ctrl Pts',(14.8733829333636,71.2443233816318,12.2647701767818));
#55034=CARTESIAN_POINT('Ctrl Pts',(14.8785467270058,71.2945589828123,12.249068855161));
#55035=CARTESIAN_POINT('Ctrl Pts',(14.8813966669327,71.3228842416262,12.2412827094571));
#55036=CARTESIAN_POINT('Ctrl Pts',(14.8874712550081,71.3843141124413,12.2266678333283));
#55037=CARTESIAN_POINT('Ctrl Pts',(14.8906853472985,71.4174725291364,12.2201639594458));
#55038=CARTESIAN_POINT('Ctrl Pts',(14.9014132207844,71.5295603224371,12.2027885712705));
#55039=CARTESIAN_POINT('Ctrl Pts',(14.9088048202201,71.6092359614705,12.1980193778373));
#55040=CARTESIAN_POINT('Ctrl Pts',(14.91972421691,71.7240322559499,12.2019472974245));
#55041=CARTESIAN_POINT('Ctrl Pts',(14.9231045297655,71.7591650869083,12.2046156587327));
#55042=CARTESIAN_POINT('Ctrl Pts',(14.9281275428201,71.810144883202,12.2106275581656));
#55043=CARTESIAN_POINT('Ctrl Pts',(14.9297180521815,71.826114158646,12.2128197734387));
#55044=CARTESIAN_POINT('Ctrl Pts',(14.9327074284313,71.8557319432653,12.2174615128714));
#55045=CARTESIAN_POINT('Ctrl Pts',(14.9341022506016,71.8693899663505,12.2198317755868));
#55046=CARTESIAN_POINT('Ctrl Pts',(14.9379401683027,71.906566753415,12.2269122244914));
#55047=CARTESIAN_POINT('Ctrl Pts',(14.9404036066684,71.9299941023716,12.2320657379584));
#55048=CARTESIAN_POINT('Ctrl Pts',(14.9501991470752,72.0217487154213,12.2549916236513));
#55049=CARTESIAN_POINT('Ctrl Pts',(14.9576632891323,72.0886885870838,12.2777844009164));
#55050=CARTESIAN_POINT('Ctrl Pts',(14.971685112274,72.2111849315068,12.331244288908));
#55051=CARTESIAN_POINT('Ctrl Pts',(14.9782370942326,72.2670350487451,12.3607436224752));
#55052=CARTESIAN_POINT('Ctrl Pts',(14.9875940308943,72.3449011490051,12.4096085389612));
#55053=CARTESIAN_POINT('Ctrl Pts',(14.9905009144876,72.3688047158754,12.4257692480362));
#55054=CARTESIAN_POINT('Ctrl Pts',(14.995699177761,72.4109576578052,12.4564109754643));
#55055=CARTESIAN_POINT('Ctrl Pts',(14.9979998490801,72.4293977176263,12.470605686936));
#55056=CARTESIAN_POINT('Ctrl Pts',(15.0031839515583,72.4703774544436,12.5039837220097));
#55057=CARTESIAN_POINT('Ctrl Pts',(15.006054278118,72.4926581163954,12.5234646046496));
#55058=CARTESIAN_POINT('Ctrl Pts',(15.0121857808431,72.5391615644335,12.5670837369629));
#55059=CARTESIAN_POINT('Ctrl Pts',(15.0154359609183,72.563131290677,12.5914573767965));
#55060=CARTESIAN_POINT('Ctrl Pts',(15.0264586787469,72.6414582315259,12.6778132522666));
#55061=CARTESIAN_POINT('Ctrl Pts',(15.0341004678183,72.6907488873929,12.7440964190608));
#55062=CARTESIAN_POINT('Ctrl Pts',(15.0450547094162,72.7500739692957,12.8425797998964));
#55063=CARTESIAN_POINT('Ctrl Pts',(15.048187766418,72.7657976174822,12.8711099278409));
#55064=CARTESIAN_POINT('Ctrl Pts',(15.0529179139282,72.7874603536593,12.9142613990469));
#55065=CARTESIAN_POINT('Ctrl Pts',(15.0544711149184,72.7942527713946,12.928442556352));
#55066=CARTESIAN_POINT('Ctrl Pts',(15.0574416316971,72.8066095283088,12.955520044123));
#55067=CARTESIAN_POINT('Ctrl Pts',(15.0588559326595,72.8122264226868,12.9683893951691));
#55068=CARTESIAN_POINT('Ctrl Pts',(15.0628436036574,72.8273417407841,13.0046495455841));
#55069=CARTESIAN_POINT('Ctrl Pts',(15.0654400750875,72.8363572428287,13.0282332221697));
#55070=CARTESIAN_POINT('Ctrl Pts',(15.0755115401593,72.8683120497401,13.1199278921612));
#55071=CARTESIAN_POINT('Ctrl Pts',(15.0831133857725,72.8861574442324,13.1896704384541));
#55072=CARTESIAN_POINT('Ctrl Pts',(15.0969656521181,72.9079524885354,13.3200120460876));
#55073=CARTESIAN_POINT('Ctrl Pts',(15.1032216474005,72.91365047315,13.3801205914671));
#55074=CARTESIAN_POINT('Ctrl Pts',(15.1122694267702,72.915721987669,13.4690252116037));
#55075=CARTESIAN_POINT('Ctrl Pts',(15.1151524317689,72.9154215180554,13.497650981896));
#55076=CARTESIAN_POINT('Ctrl Pts',(15.1203273983721,72.9131232239384,13.5494949149088));
#55077=CARTESIAN_POINT('Ctrl Pts',(15.122628181847,72.9114535835471,13.5727137465772));
#55078=CARTESIAN_POINT('Ctrl Pts',(15.127837453955,72.9061881208148,13.62557716566));
#55079=CARTESIAN_POINT('Ctrl Pts',(15.1307322902144,72.9021832539147,13.6551678180347));
#55080=CARTESIAN_POINT('Ctrl Pts',(15.1369321502809,72.8912853510357,13.7187362901842));
#55081=CARTESIAN_POINT('Ctrl Pts',(15.1402256459912,72.8840369798038,13.7526284521532));
#55082=CARTESIAN_POINT('Ctrl Pts',(15.1516201001995,72.8540199604457,13.8693997509815));
#55083=CARTESIAN_POINT('Ctrl Pts',(15.159579010404,72.8242413019048,13.9502221895792));
#55084=CARTESIAN_POINT('Ctrl Pts',(15.1707121077332,72.7731131753678,14.0548916325578));
#55085=CARTESIAN_POINT('Ctrl Pts',(15.1736643731797,72.7587042797595,14.0818728029703));
#55086=CARTESIAN_POINT('Ctrl Pts',(15.1781263249164,72.7358797538617,14.121132940331));
#55087=CARTESIAN_POINT('Ctrl Pts',(15.1795961315517,72.7281979672583,14.133828806804));
#55088=CARTESIAN_POINT('Ctrl Pts',(15.1825474325921,72.7124851301447,14.158799263465));
#55089=CARTESIAN_POINT('Ctrl Pts',(15.1840284283488,72.704460310662,14.1710750885831));
#55090=CARTESIAN_POINT('Ctrl Pts',(15.1885138951142,72.6797079287449,14.2075447179073));
#55091=CARTESIAN_POINT('Ctrl Pts',(15.1915511099815,72.6623517964571,14.2312974033249));
#55092=CARTESIAN_POINT('Ctrl Pts',(15.1994980567093,72.6152102830187,14.2913216621672));
#55093=CARTESIAN_POINT('Ctrl Pts',(15.204439160851,72.5842103376323,14.326583910747));
#55094=CARTESIAN_POINT('Ctrl Pts',(15.2175237121263,72.4970117535786,14.4153386370559));
#55095=CARTESIAN_POINT('Ctrl Pts',(15.2256180769774,72.4377334042762,14.4655501307541));
#55096=CARTESIAN_POINT('Ctrl Pts',(15.2364688499461,72.3504598248198,14.5267087662254));
#55097=CARTESIAN_POINT('Ctrl Pts',(15.2393955214991,72.326119135113,14.5425505008356));
#55098=CARTESIAN_POINT('Ctrl Pts',(15.2446136408711,72.2813327949977,14.5695593080877));
#55099=CARTESIAN_POINT('Ctrl Pts',(15.2469147608939,72.2610835513615,14.5810243618296));
#55100=CARTESIAN_POINT('Ctrl Pts',(15.2520806502773,72.2145676982552,14.6056988021584));
#55101=CARTESIAN_POINT('Ctrl Pts',(15.2549327303139,72.1881339944443,14.6185659600403));
#55102=CARTESIAN_POINT('Ctrl Pts',(15.265478793839,72.0879567899197,14.6630973513499));
#55103=CARTESIAN_POINT('Ctrl Pts',(15.2729768750885,72.0117112332123,14.6886697713735));
#55104=CARTESIAN_POINT('Ctrl Pts',(15.2862665339128,71.873981044218,14.7207567250915));
#55105=CARTESIAN_POINT('Ctrl Pts',(15.2920266258047,71.8134912599672,14.7303113450748));
#55106=CARTESIAN_POINT('Ctrl Pts',(15.2997933941884,71.7338225680731,14.7370576237826));
#55107=CARTESIAN_POINT('Ctrl Pts',(15.3016361639581,71.7150550039059,14.7382277455188));
#55108=CARTESIAN_POINT('Ctrl Pts',(15.3044043025565,71.6871607902727,14.7393459544147));
#55109=CARTESIAN_POINT('Ctrl Pts',(15.3053132419976,71.6780485569726,14.7396130026395));
#55110=CARTESIAN_POINT('Ctrl Pts',(15.3070127609763,71.6611088892174,14.7399269598222));
#55111=CARTESIAN_POINT('Ctrl Pts',(15.3078016756847,71.6532830495909,14.7399996448132));
#55112=CARTESIAN_POINT('Ctrl Pts',(15.3085940384764,71.64545743164,14.7399999987014));
#55113=CARTESIAN_POINT('Origin',(19.939,71.6454,13.47));
#55114=CARTESIAN_POINT('',(19.5292399153773,71.6444186650849,15.1743397174806));
#55115=CARTESIAN_POINT('',(19.7889963629056,70.1379689624582,12.6747475226976));
#55116=CARTESIAN_POINT('Ctrl Pts',(19.5292399154299,71.6444186643779,15.1743397174802));
#55117=CARTESIAN_POINT('Ctrl Pts',(19.5334081355681,71.5884378095259,15.1743074844656));
#55118=CARTESIAN_POINT('Ctrl Pts',(19.5375763557064,71.5325354676037,15.1715172641341));
#55119=CARTESIAN_POINT('Ctrl Pts',(19.5417445758447,71.4769114548334,15.1659912870495));
#55120=CARTESIAN_POINT('Ctrl Pts',(19.5463562733338,71.415369330973,15.159877374204));
#55121=CARTESIAN_POINT('Ctrl Pts',(19.550967970823,71.3540405821946,15.1503975106808));
#55122=CARTESIAN_POINT('Ctrl Pts',(19.5555796683121,71.2933205891731,15.137577561636));
#55123=CARTESIAN_POINT('Ctrl Pts',(19.5601909325851,71.2326063000995,15.1247588168786));
#55124=CARTESIAN_POINT('Ctrl Pts',(19.5648021968581,71.1725011599338,15.1086006332566));
#55125=CARTESIAN_POINT('Ctrl Pts',(19.5694134611311,71.1133962734374,15.0891809258151));
#55126=CARTESIAN_POINT('Ctrl Pts',(19.5740128278848,71.0544438834107,15.0698113231451));
#55127=CARTESIAN_POINT('Ctrl Pts',(19.5786121946386,70.9964870838616,15.0471971245032));
#55128=CARTESIAN_POINT('Ctrl Pts',(19.5832115613924,70.9399023287022,15.02146636167));
#55129=CARTESIAN_POINT('Ctrl Pts',(19.587808163908,70.8833515812112,14.99575106313));
#55130=CARTESIAN_POINT('Ctrl Pts',(19.5924047664236,70.8281717016542,14.966923124334));
#55131=CARTESIAN_POINT('Ctrl Pts',(19.5970013689392,70.7747195976396,14.9351588557373));
#55132=CARTESIAN_POINT('Ctrl Pts',(19.6015968666095,70.721280341442,14.9034022220414));
#55133=CARTESIAN_POINT('Ctrl Pts',(19.6061923642797,70.6695684702962,14.868710918185));
#55134=CARTESIAN_POINT('Ctrl Pts',(19.61078786195,70.6199149177897,14.8313064246392));
#55135=CARTESIAN_POINT('Ctrl Pts',(19.6154097076928,70.5699766789452,14.7936874741664));
#55136=CARTESIAN_POINT('Ctrl Pts',(19.6200315534356,70.522120864648,14.7533244120962));
#55137=CARTESIAN_POINT('Ctrl Pts',(19.6246533991784,70.4766514692552,14.7104844648289));
#55138=CARTESIAN_POINT('Ctrl Pts',(19.6292543668237,70.4313874711258,14.6678380369136));
#55139=CARTESIAN_POINT('Ctrl Pts',(19.6338553344691,70.3884886980699,14.622737453413));
#55140=CARTESIAN_POINT('Ctrl Pts',(19.6384563021145,70.3482171986574,14.5754825260949));
#55141=CARTESIAN_POINT('Ctrl Pts',(19.643088586906,70.3076715855085,14.5279059513366));
#55142=CARTESIAN_POINT('Ctrl Pts',(19.6477208716975,70.2697894690637,14.4781460013856));
#55143=CARTESIAN_POINT('Ctrl Pts',(19.652353156489,70.2347948046825,14.4265395018207));
#55144=CARTESIAN_POINT('Ctrl Pts',(19.6569854412805,70.1998001403013,14.3749330022558));
#55145=CARTESIAN_POINT('Ctrl Pts',(19.661617726072,70.1676931439373,14.3214804259295));
#55146=CARTESIAN_POINT('Ctrl Pts',(19.6662500108635,70.1386503546158,14.2665427431938));
#55147=CARTESIAN_POINT('Ctrl Pts',(19.6708443877018,70.1098452347706,14.2120546388416));
#55148=CARTESIAN_POINT('Ctrl Pts',(19.6754387645401,70.0839421319649,14.1558933370675));
#55149=CARTESIAN_POINT('Ctrl Pts',(19.6800331413783,70.0611374155199,14.0984002697456));
#55150=CARTESIAN_POINT('Ctrl Pts',(19.6846198308241,70.0383708563294,14.0410034008401));
#55151=CARTESIAN_POINT('Ctrl Pts',(19.6892065202698,70.0186925768024,13.9822796606064));
#55152=CARTESIAN_POINT('Ctrl Pts',(19.6937932097156,70.0022525532405,13.9225939723503));
#55153=CARTESIAN_POINT('Ctrl Pts',(19.6983756147656,69.9858278861939,13.8629640360935));
#55154=CARTESIAN_POINT('Ctrl Pts',(19.7029580198156,69.9726356143561,13.8023744217564));
#55155=CARTESIAN_POINT('Ctrl Pts',(19.7075404248657,69.9627766285917,13.7412073479659));
#55156=CARTESIAN_POINT('Ctrl Pts',(19.7121202365844,69.9529232223464,13.6800748906018));
#55157=CARTESIAN_POINT('Ctrl Pts',(19.7167000483031,69.9463994422805,13.6183661239773));
#55158=CARTESIAN_POINT('Ctrl Pts',(19.7212798600218,69.9432551338905,13.5564736397827));
#55159=CARTESIAN_POINT('Ctrl Pts',(19.7258587659086,69.9401114474072,13.4945933971816));
#55160=CARTESIAN_POINT('Ctrl Pts',(19.7304376717953,69.9403459308535,13.4325300178702));
#55161=CARTESIAN_POINT('Ctrl Pts',(19.735016577682,69.9439564243733,13.3706793346843));
#55162=CARTESIAN_POINT('Ctrl Pts',(19.7395995429358,69.9475701187275,13.3087738186113));
#55163=CARTESIAN_POINT('Ctrl Pts',(19.7441825081896,69.9545657749991,13.2470818853951));
#55164=CARTESIAN_POINT('Ctrl Pts',(19.7487654734434,69.9648891529298,13.1859962527016));
#55165=CARTESIAN_POINT('Ctrl Pts',(19.7533503268661,69.9752167840633,13.124885452899));
#55166=CARTESIAN_POINT('Ctrl Pts',(19.7579351802887,69.9888747583705,13.0643819498165));
#55167=CARTESIAN_POINT('Ctrl Pts',(19.7625200337113,70.005757866363,13.0048672133656));
#55168=CARTESIAN_POINT('Ctrl Pts',(19.7671134700236,70.0226725796959,12.9452410647561));
#55169=CARTESIAN_POINT('Ctrl Pts',(19.7717069063359,70.0428243259473,12.8866078653173));
#55170=CARTESIAN_POINT('Ctrl Pts',(19.7763003426482,70.0660585204686,12.8293321245516));
#55171=CARTESIAN_POINT('Ctrl Pts',(19.7805323494007,70.0874645575652,12.7765630633974));
#55172=CARTESIAN_POINT('Ctrl Pts',(19.7847643561531,70.1114863591526,12.7249462951846));
#55173=CARTESIAN_POINT('Ctrl Pts',(19.7889963629056,70.1379689624582,12.6747475226976));
#55174=CARTESIAN_POINT('',(19.789,70.1379459883857,14.2652089275579));
#55175=CARTESIAN_POINT('Origin',(19.789,71.6454,13.47));
#55176=CARTESIAN_POINT('',(19.6518850845702,71.6441855388828,15.174605651636));
#55177=CARTESIAN_POINT('Ctrl Pts',(19.789,70.1379459883857,14.2652089275579));
#55178=CARTESIAN_POINT('Ctrl Pts',(19.7474981883271,70.3991888501049,14.7604392830743));
#55179=CARTESIAN_POINT('Ctrl Pts',(19.7017932165172,70.9742539043654,15.1485528849809));
#55180=CARTESIAN_POINT('Ctrl Pts',(19.6560882447072,71.5877183033873,15.1763527703962));
#55181=CARTESIAN_POINT('Ctrl Pts',(19.6518850845702,71.6441845643294,15.1759735251619));
#55182=CARTESIAN_POINT('',(18.858135084626,71.6451886815825,15.1743399868995));
#55183=CARTESIAN_POINT('Ctrl Pts',(19.6518850845702,71.6441857284568,15.1743395674409));
#55184=CARTESIAN_POINT('Ctrl Pts',(19.6472227531282,71.7067602847858,15.1743841492276));
#55185=CARTESIAN_POINT('Ctrl Pts',(19.6425604216862,71.7694858767845,15.1709778041751));
#55186=CARTESIAN_POINT('Ctrl Pts',(19.6378980902442,71.8319411817604,15.1641007122091));
#55187=CARTESIAN_POINT('Ctrl Pts',(19.6333926468792,71.8922948573665,15.1574550353081));
#55188=CARTESIAN_POINT('Ctrl Pts',(19.6288872035141,71.9523955681993,15.1475685326357));
#55189=CARTESIAN_POINT('Ctrl Pts',(19.624381760149,72.0118616368733,15.1344761050553));
#55190=CARTESIAN_POINT('Ctrl Pts',(19.6198801777333,72.0712767459725,15.1213948970588));
#55191=CARTESIAN_POINT('Ctrl Pts',(19.6153785953175,72.1300577754547,15.1051133163245));
#55192=CARTESIAN_POINT('Ctrl Pts',(19.6108770129018,72.1878305538533,15.0857177754318));
#55193=CARTESIAN_POINT('Ctrl Pts',(19.6063775010452,72.2455767589396,15.0663311557609));
#55194=CARTESIAN_POINT('Ctrl Pts',(19.6018779891886,72.3023151312258,15.0438335819748));
#55195=CARTESIAN_POINT('Ctrl Pts',(19.5973784773321,72.3576863001101,15.0183614120338));
#55196=CARTESIAN_POINT('Ctrl Pts',(19.5928792492668,72.4130539766476,14.9928908486628));
#55197=CARTESIAN_POINT('Ctrl Pts',(19.5883800212015,72.4670541418949,14.9644462851191));
#55198=CARTESIAN_POINT('Ctrl Pts',(19.5838807931362,72.5193492133626,14.9332114023828));
#55199=CARTESIAN_POINT('Ctrl Pts',(19.5793772343218,72.5716946216507,14.901946454391));
#55200=CARTESIAN_POINT('Ctrl Pts',(19.5748736755074,72.6223312086906,14.8678861028988));
#55201=CARTESIAN_POINT('Ctrl Pts',(19.570370116693,72.6709491311669,14.831258173589));
#55202=CARTESIAN_POINT('Ctrl Pts',(19.5658639275193,72.7195954495422,14.7946088512839));
#55203=CARTESIAN_POINT('Ctrl Pts',(19.5613577383457,72.766220357122,14.7553893123699));
#55204=CARTESIAN_POINT('Ctrl Pts',(19.556851549172,72.810548448634,14.7138665234846));
#55205=CARTESIAN_POINT('Ctrl Pts',(19.5523379098736,72.8549498281948,14.6722750845837));
#55206=CARTESIAN_POINT('Ctrl Pts',(19.5478242705752,72.8970464603924,14.6283731881336));
#55207=CARTESIAN_POINT('Ctrl Pts',(19.5433106312768,72.9366020707453,14.5824621558072));
#55208=CARTESIAN_POINT('Ctrl Pts',(19.542203464172,72.9463048111941,14.5712004706397));
#55209=CARTESIAN_POINT('Ctrl Pts',(19.5410962970673,72.9558548642394,14.5598180361732));
#55210=CARTESIAN_POINT('Ctrl Pts',(19.5399891299625,72.9652491465984,14.5483195564504));
#55211=CARTESIAN_POINT('Ctrl Pts',(19.5353826477796,73.0043350209182,14.5004789533968));
#55212=CARTESIAN_POINT('Ctrl Pts',(19.5307761655967,73.0408937684296,14.4504158455636));
#55213=CARTESIAN_POINT('Ctrl Pts',(19.5261696834138,73.0746645583352,14.3984275189195));
#55214=CARTESIAN_POINT('Ctrl Pts',(19.5215577672275,73.1084751857084,14.3463778646225));
#55215=CARTESIAN_POINT('Ctrl Pts',(19.5169458510412,73.1394909176284,14.2923988142978));
#55216=CARTESIAN_POINT('Ctrl Pts',(19.512333934855,73.1674899195399,14.2368227386006));
#55217=CARTESIAN_POINT('Ctrl Pts',(19.5077398498217,73.1953806682949,14.1814615379067));
#55218=CARTESIAN_POINT('Ctrl Pts',(19.5031457647884,73.2202777143286,14.1245160771108));
#55219=CARTESIAN_POINT('Ctrl Pts',(19.498551679755,73.2420059035321,14.0663425394908));
#55220=CARTESIAN_POINT('Ctrl Pts',(19.4939603691465,73.2637209708136,14.0082041335893));
#55221=CARTESIAN_POINT('Ctrl Pts',(19.4893690585379,73.2822707998122,13.9488395953978));
#55222=CARTESIAN_POINT('Ctrl Pts',(19.4847777479293,73.2975282063429,13.8886253998578));
#55223=CARTESIAN_POINT('Ctrl Pts',(19.4801875437516,73.3127819360878,13.8284257149559));
#55224=CARTESIAN_POINT('Ctrl Pts',(19.475597339574,73.3247446945025,13.7673772701358));
#55225=CARTESIAN_POINT('Ctrl Pts',(19.4710071353963,73.3333396153203,13.7058700715062));
#55226=CARTESIAN_POINT('Ctrl Pts',(19.4663801820252,73.3420033471093,13.6438704459933));
#55227=CARTESIAN_POINT('Ctrl Pts',(19.4617532286542,73.3472449687181,13.5814052001833));
#55228=CARTESIAN_POINT('Ctrl Pts',(19.4571262752831,73.3490389145714,13.5188803064433));
#55229=CARTESIAN_POINT('Ctrl Pts',(19.4525305464212,73.3508207541694,13.4567773553848));
#55230=CARTESIAN_POINT('Ctrl Pts',(19.4479348175592,73.349201374521,13.3946160704898));
#55231=CARTESIAN_POINT('Ctrl Pts',(19.4433390886972,73.3442081332339,13.3327929955936));
#55232=CARTESIAN_POINT('Ctrl Pts',(19.4386965230716,73.3391640039879,13.2703398589962));
#55233=CARTESIAN_POINT('Ctrl Pts',(19.434053957446,73.330676909655,13.2082323908635));
#55234=CARTESIAN_POINT('Ctrl Pts',(19.4294113918204,73.3188282118031,13.1468702187333));
#55235=CARTESIAN_POINT('Ctrl Pts',(19.4247688261948,73.3069795139512,13.0855080466031));
#55236=CARTESIAN_POINT('Ctrl Pts',(19.4201262605693,73.2917693994114,13.0248916663312));
#55237=CARTESIAN_POINT('Ctrl Pts',(19.4154836949437,73.2733304595571,12.965403869965));
#55238=CARTESIAN_POINT('Ctrl Pts',(19.4108727106458,73.2550169516837,12.9063207428584));
#55239=CARTESIAN_POINT('Ctrl Pts',(19.406261726348,73.2334478747545,12.8481231124961));
#55240=CARTESIAN_POINT('Ctrl Pts',(19.4016507420502,73.2087284876023,12.7911930499391));
#55241=CARTESIAN_POINT('Ctrl Pts',(19.3970393886283,73.184007121584,12.7342584299483));
#55242=CARTESIAN_POINT('Ctrl Pts',(19.3924280352064,73.1561350620157,12.678592074235));
#55243=CARTESIAN_POINT('Ctrl Pts',(19.3878166817845,73.1252677430926,12.6245614755916));
#55244=CARTESIAN_POINT('Ctrl Pts',(19.3832176093261,73.0944826300603,12.5706747713206));
#55245=CARTESIAN_POINT('Ctrl Pts',(19.3786185368676,73.0607184085154,12.5184155797055));
#55246=CARTESIAN_POINT('Ctrl Pts',(19.3740194644092,73.0241765763943,12.4681267605198));
#55247=CARTESIAN_POINT('Ctrl Pts',(19.3694229982887,72.9876554528757,12.4178664404846));
#55248=CARTESIAN_POINT('Ctrl Pts',(19.3648265321682,72.9483601375223,12.3695746861601));
#55249=CARTESIAN_POINT('Ctrl Pts',(19.3602300660477,72.9065354499344,12.3235654346982));
#55250=CARTESIAN_POINT('Ctrl Pts',(19.3556345471125,72.864719381083,12.2775656642783));
#55251=CARTESIAN_POINT('Ctrl Pts',(19.3510390281773,72.8203753150686,12.2338478362991));
#55252=CARTESIAN_POINT('Ctrl Pts',(19.3464435092422,72.7737870453277,12.1926913013932));
#55253=CARTESIAN_POINT('Ctrl Pts',(19.3418214051324,72.7269292614575,12.1512966750592));
#55254=CARTESIAN_POINT('Ctrl Pts',(19.3371993010226,72.6778015952658,12.1124934315799));
#55255=CARTESIAN_POINT('Ctrl Pts',(19.3325771969128,72.6267271955063,12.0765252887261));
#55256=CARTESIAN_POINT('Ctrl Pts',(19.3279758236866,72.5758818726795,12.0407184688029));
#55257=CARTESIAN_POINT('Ctrl Pts',(19.3233744504603,72.5231076989931,12.0077216037023));
#55258=CARTESIAN_POINT('Ctrl Pts',(19.3187730772341,72.4687512366767,11.9777307291702));
#55259=CARTESIAN_POINT('Ctrl Pts',(19.3141406076826,72.4140274304933,11.9475371747109));
#55260=CARTESIAN_POINT('Ctrl Pts',(19.309508138131,72.3577003334321,11.9203906244013));
#55261=CARTESIAN_POINT('Ctrl Pts',(19.3048756685795,72.3001449413085,11.8964422802353));
#55262=CARTESIAN_POINT('Ctrl Pts',(19.300243199028,72.2425895491849,11.8724939360694));
#55263=CARTESIAN_POINT('Ctrl Pts',(19.2956107294764,72.1838063688168,11.8517439127542));
#55264=CARTESIAN_POINT('Ctrl Pts',(19.2909782599249,72.1241843895038,11.8342920969906));
#55265=CARTESIAN_POINT('Ctrl Pts',(19.286378296262,72.064980775686,11.8169627400522));
#55266=CARTESIAN_POINT('Ctrl Pts',(19.281778332599,72.00471595295,11.80281691182));
#55267=CARTESIAN_POINT('Ctrl Pts',(19.2771783689361,71.9437642251172,11.7919792537724));
#55268=CARTESIAN_POINT('Ctrl Pts',(19.2725656379349,71.8826433239197,11.781111515477));
#55269=CARTESIAN_POINT('Ctrl Pts',(19.2679529069336,71.8208321764191,11.7735705373702));
#55270=CARTESIAN_POINT('Ctrl Pts',(19.2633401759324,71.7587241672146,11.7694317218279));
#55271=CARTESIAN_POINT('Ctrl Pts',(19.2587526068373,71.69695494991,11.7653154830386));
#55272=CARTESIAN_POINT('Ctrl Pts',(19.2541650377422,71.63489261025,11.7645644418691));
#55273=CARTESIAN_POINT('Ctrl Pts',(19.2495774686471,71.5729324668579,11.7672013353775));
#55274=CARTESIAN_POINT('Ctrl Pts',(19.2449926537738,71.511009522247,11.7698366457838));
#55275=CARTESIAN_POINT('Ctrl Pts',(19.2404078389006,71.4491891590318,11.7758558357454));
#55276=CARTESIAN_POINT('Ctrl Pts',(19.2358230240273,71.3878667231025,11.7852295566189));
#55277=CARTESIAN_POINT('Ctrl Pts',(19.231239283968,71.3265586629355,11.7946010800197));
#55278=CARTESIAN_POINT('Ctrl Pts',(19.2266555439086,71.2657488004955,11.8073254961146));
#55279=CARTESIAN_POINT('Ctrl Pts',(19.2220718038493,71.2058253451771,11.8233218412703));
#55280=CARTESIAN_POINT('Ctrl Pts',(19.2174385556041,71.1452546669515,11.8394909601915));
#55281=CARTESIAN_POINT('Ctrl Pts',(19.2128053073588,71.0855901798453,11.8590030134026));
#55282=CARTESIAN_POINT('Ctrl Pts',(19.2081720591135,71.0272179277177,11.8817223916743));
#55283=CARTESIAN_POINT('Ctrl Pts',(19.2035826403476,70.969397863879,11.9042268497715));
#55284=CARTESIAN_POINT('Ctrl Pts',(19.1989932215818,70.9128461350012,11.9298779404172));
#55285=CARTESIAN_POINT('Ctrl Pts',(19.1944038028159,70.8579162553476,11.9584960511106));
#55286=CARTESIAN_POINT('Ctrl Pts',(19.1897486398309,70.80219949565,11.9875241211986));
#55287=CARTESIAN_POINT('Ctrl Pts',(19.185093476846,70.7481518940692,12.019604631197));
#55288=CARTESIAN_POINT('Ctrl Pts',(19.180438313861,70.6961127090668,12.0545041593587));
#55289=CARTESIAN_POINT('Ctrl Pts',(19.1757831508761,70.6440735240645,12.0894036875204));
#55290=CARTESIAN_POINT('Ctrl Pts',(19.1711279878911,70.5940431473507,12.1271218584828));
#55291=CARTESIAN_POINT('Ctrl Pts',(19.1664728249062,70.5463246698812,12.1673840725969));
#55292=CARTESIAN_POINT('Ctrl Pts',(19.1618680212956,70.4991224090686,12.2072107316248));
#55293=CARTESIAN_POINT('Ctrl Pts',(19.1572632176851,70.4539945476355,12.2496849530029));
#55294=CARTESIAN_POINT('Ctrl Pts',(19.1526584140745,70.4112518911924,12.2945625150071));
#55295=CARTESIAN_POINT('Ctrl Pts',(19.1480462880667,70.3684412668755,12.3395114397368));
#55296=CARTESIAN_POINT('Ctrl Pts',(19.1434341620589,70.3280238600468,12.3868710604633));
#55297=CARTESIAN_POINT('Ctrl Pts',(19.1388220360511,70.2902789032634,12.4363551631341));
#55298=CARTESIAN_POINT('Ctrl Pts',(19.1342294856661,70.2526941504803,12.4856292363898));
#55299=CARTESIAN_POINT('Ctrl Pts',(19.1296369352811,70.2177595391408,12.5370094069176));
#55300=CARTESIAN_POINT('Ctrl Pts',(19.1250443848961,70.1857124416265,12.590177820506));
#55301=CARTESIAN_POINT('Ctrl Pts',(19.1204545500048,70.1536842929931,12.6433147965536));
#55302=CARTESIAN_POINT('Ctrl Pts',(19.1158647151135,70.1245405333473,12.6982374852746));
#55303=CARTESIAN_POINT('Ctrl Pts',(19.1112748802221,70.0984750930454,12.7545992956089));
#55304=CARTESIAN_POINT('Ctrl Pts',(19.1066860900192,70.0724155854758,12.81094827748));
#55305=CARTESIAN_POINT('Ctrl Pts',(19.1020972998162,70.0494332186248,12.8687352705196));
#55306=CARTESIAN_POINT('Ctrl Pts',(19.0975085096132,70.0296749321915,12.9275911681626));
#55307=CARTESIAN_POINT('Ctrl Pts',(19.0928800829694,70.0097459802631,12.9869554434395));
#55308=CARTESIAN_POINT('Ctrl Pts',(19.0882516563256,69.9930972735942,13.0474066928886));
#55309=CARTESIAN_POINT('Ctrl Pts',(19.0836232296818,69.9798284057046,13.1085500036295));
#55310=CARTESIAN_POINT('Ctrl Pts',(19.0790287453758,69.9666568444012,13.1692449229259));
#55311=CARTESIAN_POINT('Ctrl Pts',(19.0744342610697,69.9568157404246,13.2306212706332));
#55312=CARTESIAN_POINT('Ctrl Pts',(19.0698397767637,69.9503507341686,13.2922844351097));
#55313=CARTESIAN_POINT('Ctrl Pts',(19.065194378951,69.9438140863272,13.3546309163049));
#55314=CARTESIAN_POINT('Ctrl Pts',(19.0605489811383,69.9407288640072,13.4172700805852));
#55315=CARTESIAN_POINT('Ctrl Pts',(19.0559035833256,69.9410881372469,13.4797933691354));
#55316=CARTESIAN_POINT('Ctrl Pts',(19.0512581855128,69.9414474104865,13.5423166576857));
#55317=CARTESIAN_POINT('Ctrl Pts',(19.0466127877001,69.9452510851302,13.6047235462825));
#55318=CARTESIAN_POINT('Ctrl Pts',(19.0419673898874,69.9524386089449,13.666612725928));
#55319=CARTESIAN_POINT('Ctrl Pts',(19.0373625663435,69.9595633548157,13.7279613473019));
#55320=CARTESIAN_POINT('Ctrl Pts',(19.0327577427996,69.9700410980345,13.7890430378238));
#55321=CARTESIAN_POINT('Ctrl Pts',(19.0281529192557,69.9838398718812,13.8494638009692));
#55322=CARTESIAN_POINT('Ctrl Pts',(19.0235407957396,69.9976605207607,13.9099803484349));
#55323=CARTESIAN_POINT('Ctrl Pts',(19.0189286722234,70.0148127251835,13.969833358198));
#55324=CARTESIAN_POINT('Ctrl Pts',(19.0143165487073,70.0352120763954,14.0286319774931));
#55325=CARTESIAN_POINT('Ctrl Pts',(19.0097239409176,70.0555251098499,14.0871817964759));
#55326=CARTESIAN_POINT('Ctrl Pts',(19.005131333128,70.0790577259536,14.1446856402258));
#55327=CARTESIAN_POINT('Ctrl Pts',(19.0005387253383,70.1056760189816,14.2007700718261));
#55328=CARTESIAN_POINT('Ctrl Pts',(18.9959488190682,70.1322786542737,14.2568215127606));
#55329=CARTESIAN_POINT('Ctrl Pts',(18.9913589127981,70.161963149739,14.311454740292));
#55330=CARTESIAN_POINT('Ctrl Pts',(18.986769006528,70.1945476521967,14.3643166667762));
#55331=CARTESIAN_POINT('Ctrl Pts',(18.9821801310537,70.2271248368648,14.4171667215906));
#55332=CARTESIAN_POINT('Ctrl Pts',(18.9775912555794,70.2626004692729,14.4682458339003));
#55333=CARTESIAN_POINT('Ctrl Pts',(18.9730023801051,70.3007479760522,14.517227659152));
#55334=CARTESIAN_POINT('Ctrl Pts',(18.9683740113354,70.339223792188,14.5666310372885));
#55335=CARTESIAN_POINT('Ctrl Pts',(18.9637456425657,70.3804173990726,14.6139004212703));
#55336=CARTESIAN_POINT('Ctrl Pts',(18.959117273796,70.4240545923065,14.6587347183901));
#55337=CARTESIAN_POINT('Ctrl Pts',(18.9545226708685,70.4673734343775,14.7032419309847));
#55338=CARTESIAN_POINT('Ctrl Pts',(18.9499280679409,70.5130999105703,14.7453491627486));
#55339=CARTESIAN_POINT('Ctrl Pts',(18.9453334650134,70.5609302450361,14.7848004358718));
#55340=CARTESIAN_POINT('Ctrl Pts',(18.9406882133226,70.6092878388378,14.82468660146));
#55341=CARTESIAN_POINT('Ctrl Pts',(18.9360429616318,70.6597955412824,14.8618575655445));
#55342=CARTESIAN_POINT('Ctrl Pts',(18.931397709941,70.7121089816365,14.8960935139892));
#55343=CARTESIAN_POINT('Ctrl Pts',(18.9267524582502,70.7644224219906,14.9303294624338));
#55344=CARTESIAN_POINT('Ctrl Pts',(18.9221072065594,70.8185411113404,14.9616301843882));
#55345=CARTESIAN_POINT('Ctrl Pts',(18.9174619548686,70.8740971202776,14.9898245633401));
#55346=CARTESIAN_POINT('Ctrl Pts',(18.912518049015,70.9332249557679,15.0198316252639));
#55347=CARTESIAN_POINT('Ctrl Pts',(18.9075741431615,70.9941931861682,15.046428425153));
#55348=CARTESIAN_POINT('Ctrl Pts',(18.9026302373079,71.0565973538058,15.0694018505162));
#55349=CARTESIAN_POINT('Ctrl Pts',(18.8977597888335,71.1180743098957,15.0920339328875));
#55350=CARTESIAN_POINT('Ctrl Pts',(18.892889340359,71.1809444334017,15.1111493959224));
#55351=CARTESIAN_POINT('Ctrl Pts',(18.8880188918845,71.2447962575595,15.1265903166271));
#55352=CARTESIAN_POINT('Ctrl Pts',(18.8830382573414,71.3100926266119,15.1423805633451));
#55353=CARTESIAN_POINT('Ctrl Pts',(18.8780576227984,71.376415286907,15.1543277305986));
#55354=CARTESIAN_POINT('Ctrl Pts',(18.8730769882553,71.4433035472524,15.1623155318636));
#55355=CARTESIAN_POINT('Ctrl Pts',(18.8680963537122,71.5101918075978,15.1703033331287));
#55356=CARTESIAN_POINT('Ctrl Pts',(18.8631157191691,71.5776452193343,15.1743316122925));
#55357=CARTESIAN_POINT('Ctrl Pts',(18.858135084626,71.6451886815825,15.1743399868995));
#55358=CARTESIAN_POINT('',(18.0643850846152,71.6466158347437,15.1743395663265));
#55359=CARTESIAN_POINT('Ctrl Pts',(18.8581350845702,71.6451886823392,15.1743399868996));
#55360=CARTESIAN_POINT('Ctrl Pts',(18.8533776934734,71.709704691929,15.1743479861089));
#55361=CARTESIAN_POINT('Ctrl Pts',(18.8486203023767,71.774167687991,15.1706883871686));
#55362=CARTESIAN_POINT('Ctrl Pts',(18.8438629112799,71.8381538247881,15.1634050899385));
#55363=CARTESIAN_POINT('Ctrl Pts',(18.8390945725359,71.9022872056611,15.1561050324783));
#55364=CARTESIAN_POINT('Ctrl Pts',(18.8343262337919,71.9659410868059,15.1451646747383));
#55365=CARTESIAN_POINT('Ctrl Pts',(18.8295578950479,72.0286995066004,15.1306794765517));
#55366=CARTESIAN_POINT('Ctrl Pts',(18.8247837352535,72.0915345400639,15.1161765952529));
#55367=CARTESIAN_POINT('Ctrl Pts',(18.8200095754591,72.1534715015155,15.0981203771717));
#55368=CARTESIAN_POINT('Ctrl Pts',(18.8152354156646,72.2141102507751,15.0766559949981));
#55369=CARTESIAN_POINT('Ctrl Pts',(18.8104493894206,72.2748997211437,15.0551382618645));
#55370=CARTESIAN_POINT('Ctrl Pts',(18.8056633631767,72.3343841154749,15.0301956123921));
#55371=CARTESIAN_POINT('Ctrl Pts',(18.8008773369327,72.392183944088,15.0020210757207));
#55372=CARTESIAN_POINT('Ctrl Pts',(18.7982370645717,72.424069956027,14.9864782335663));
#55373=CARTESIAN_POINT('Ctrl Pts',(18.7955967922108,72.4554437540396,14.9699526329256));
#55374=CARTESIAN_POINT('Ctrl Pts',(18.7929565198498,72.4862453494548,14.9524823553419));
#55375=CARTESIAN_POINT('Ctrl Pts',(18.7883522396236,72.5399591930735,14.9220165387032));
#55376=CARTESIAN_POINT('Ctrl Pts',(18.7837479593973,72.5921212668839,14.8885675029417));
#55377=CARTESIAN_POINT('Ctrl Pts',(18.7791436791711,72.6423812110903,14.8523180894182));
#55378=CARTESIAN_POINT('Ctrl Pts',(18.7745314877402,72.6927275133553,14.8160063911266));
#55379=CARTESIAN_POINT('Ctrl Pts',(18.7699192963094,72.7411646753013,14.7768848943094));
#55380=CARTESIAN_POINT('Ctrl Pts',(18.7653071048786,72.7873655229722,14.73518361511));
#55381=CARTESIAN_POINT('Ctrl Pts',(18.7607150744532,72.8333644155519,14.6936646222985));
#55382=CARTESIAN_POINT('Ctrl Pts',(18.7561230440278,72.87714610762,14.6495886741211));
#55383=CARTESIAN_POINT('Ctrl Pts',(18.7515310136024,72.9184188786279,14.6032245012605));
#55384=CARTESIAN_POINT('Ctrl Pts',(18.7469416958328,72.9596672685202,14.5568877171656));
#55385=CARTESIAN_POINT('Ctrl Pts',(18.7423523780633,72.9984093401351,14.5082657672341));
#55386=CARTESIAN_POINT('Ctrl Pts',(18.7377630602938,73.0343907899462,14.4576636173539));
#55387=CARTESIAN_POINT('Ctrl Pts',(18.7331747834526,73.0703640786072,14.4070729448251));
#55388=CARTESIAN_POINT('Ctrl Pts',(18.7285865066114,73.1035776951015,14.3545033773746));
#55389=CARTESIAN_POINT('Ctrl Pts',(18.7239982297702,73.1338193861151,14.3002906519025));
#55390=CARTESIAN_POINT('Ctrl Pts',(18.7193693010253,73.1643290170015,14.2455976043891));
#55391=CARTESIAN_POINT('Ctrl Pts',(18.7147403722804,73.1918135140614,14.189232578808));
#55392=CARTESIAN_POINT('Ctrl Pts',(18.7101114435354,73.2161023138299,14.1315656255653));
#55393=CARTESIAN_POINT('Ctrl Pts',(18.7055174572231,73.2402077645351,14.0743339833283));
#55394=CARTESIAN_POINT('Ctrl Pts',(18.7009234709108,73.2611654804613,14.0158205052203));
#55395=CARTESIAN_POINT('Ctrl Pts',(18.6963294845985,73.2788581046431,13.9564046216635));
#55396=CARTESIAN_POINT('Ctrl Pts',(18.6916830846372,73.2967525872828,13.8963108511804));
#55397=CARTESIAN_POINT('Ctrl Pts',(18.687036684676,73.3113068618472,13.8352944667737));
#55398=CARTESIAN_POINT('Ctrl Pts',(18.6823902847148,73.3224526273905,13.7737586551238));
#55399=CARTESIAN_POINT('Ctrl Pts',(18.6777438847535,73.3335983929338,13.7122228434739));
#55400=CARTESIAN_POINT('Ctrl Pts',(18.6730974847923,73.3413356457848,13.6501681381785));
#55401=CARTESIAN_POINT('Ctrl Pts',(18.6684510848311,73.3456501962626,13.5880004479189));
#55402=CARTESIAN_POINT('Ctrl Pts',(18.6638468640006,73.3499255800758,13.5263971040692));
#55403=CARTESIAN_POINT('Ctrl Pts',(18.6592426431701,73.3508570957658,13.4644393755095));
#55404=CARTESIAN_POINT('Ctrl Pts',(18.6546384223397,73.3484036191377,13.402520308211));
#55405=CARTESIAN_POINT('Ctrl Pts',(18.6500262234844,73.3459458912153,13.3404939498256));
#55406=CARTESIAN_POINT('Ctrl Pts',(18.6454140246291,73.3400913468835,13.2785068938624));
#55407=CARTESIAN_POINT('Ctrl Pts',(18.6408018257738,73.3308509946095,13.2169589354079));
#55408=CARTESIAN_POINT('Ctrl Pts',(18.6362098527738,73.3216511640115,13.1556808829443));
#55409=CARTESIAN_POINT('Ctrl Pts',(18.6316178797738,73.3090952070524,13.0948385923167));
#55410=CARTESIAN_POINT('Ctrl Pts',(18.6270259067737,73.2932459881658,13.0348236737988));
#55411=CARTESIAN_POINT('Ctrl Pts',(18.6224366455156,73.2774061288703,12.974844196466));
#55412=CARTESIAN_POINT('Ctrl Pts',(18.6178473842574,73.2582769938693,12.9156916116504));
#55413=CARTESIAN_POINT('Ctrl Pts',(18.6132581229993,73.23597232155,12.8577463552424));
#55414=CARTESIAN_POINT('Ctrl Pts',(18.6086699016529,73.2136727033977,12.799814229043));
#55415=CARTESIAN_POINT('Ctrl Pts',(18.6040816803066,73.1881991589405,12.7430893610911));
#55416=CARTESIAN_POINT('Ctrl Pts',(18.5994934589603,73.1597143048886,12.6879341321795));
#55417=CARTESIAN_POINT('Ctrl Pts',(18.5948644748646,73.1309763852414,12.6322888923026));
#55418=CARTESIAN_POINT('Ctrl Pts',(18.590235490769,73.0991735938314,12.5782418013657));
#55419=CARTESIAN_POINT('Ctrl Pts',(18.5856065066733,73.0645201952379,12.5261394663045));
#55420=CARTESIAN_POINT('Ctrl Pts',(18.5810125726861,73.030129187993,12.4744316438312));
#55421=CARTESIAN_POINT('Ctrl Pts',(18.5764186386989,72.9929309481254,12.4246396047205));
#55422=CARTESIAN_POINT('Ctrl Pts',(18.5718247047117,72.9531769349122,12.3770707597875));
#55423=CARTESIAN_POINT('Ctrl Pts',(18.5671781955618,72.9129679578885,12.3289575143976));
#55424=CARTESIAN_POINT('Ctrl Pts',(18.5625316864119,72.8701446873665,12.2831190737208));
#55425=CARTESIAN_POINT('Ctrl Pts',(18.557885177262,72.8250055143118,12.2398351060914));
#55426=CARTESIAN_POINT('Ctrl Pts',(18.5532386681121,72.7798663412571,12.196551138462));
#55427=CARTESIAN_POINT('Ctrl Pts',(18.5485921589622,72.7324117085443,12.1558219417343));
#55428=CARTESIAN_POINT('Ctrl Pts',(18.5439456498123,72.6829721695382,12.1178835743178));
#55429=CARTESIAN_POINT('Ctrl Pts',(18.5393415477255,72.6339838479048,12.0802914571052));
#55430=CARTESIAN_POINT('Ctrl Pts',(18.5347374456387,72.5828530488402,12.0452907683919));
#55431=CARTESIAN_POINT('Ctrl Pts',(18.5301333435519,72.5298846624105,12.0131329101251));
#55432=CARTESIAN_POINT('Ctrl Pts',(18.5255211298536,72.4768229550764,11.9809183954144));
#55433=CARTESIAN_POINT('Ctrl Pts',(18.5209089161553,72.4219175562888,11.9515570867998));
#55434=CARTESIAN_POINT('Ctrl Pts',(18.5162967024571,72.3655078129013,11.9252606778493));
#55435=CARTESIAN_POINT('Ctrl Pts',(18.5117048541812,72.309347149094,11.8990803817919));
#55436=CARTESIAN_POINT('Ctrl Pts',(18.5071130059053,72.2516958474173,11.8759382160423));
#55437=CARTESIAN_POINT('Ctrl Pts',(18.5025211576295,72.1929150497117,11.8559981084462));
#55438=CARTESIAN_POINT('Ctrl Pts',(18.4979320229831,72.134168989501,11.83606978479));
#55439=CARTESIAN_POINT('Ctrl Pts',(18.4933428883367,72.0742952364289,11.8193399290415));
#55440=CARTESIAN_POINT('Ctrl Pts',(18.4887537536904,72.0136737223021,11.8059238896428));
#55441=CARTESIAN_POINT('Ctrl Pts',(18.4841656606265,71.9530659672642,11.7925108952435));
#55442=CARTESIAN_POINT('Ctrl Pts',(18.4795775675627,71.8917112831891,11.7824103331851));
#55443=CARTESIAN_POINT('Ctrl Pts',(18.4749894744989,71.830001553527,11.7756868347217));
#55444=CARTESIAN_POINT('Ctrl Pts',(18.4703603695234,71.7677402147445,11.7689032364475));
#55445=CARTESIAN_POINT('Ctrl Pts',(18.465731264548,71.7051179685949,11.7655574681876));
#55446=CARTESIAN_POINT('Ctrl Pts',(18.4611021595725,71.6425421472726,11.7656623960383));
#55447=CARTESIAN_POINT('Ctrl Pts',(18.4565083564861,71.580443533685,11.7657665237017));
#55448=CARTESIAN_POINT('Ctrl Pts',(18.4519145533996,71.5183911493209,11.769268812178));
#55449=CARTESIAN_POINT('Ctrl Pts',(18.4473207503132,71.4567801341243,11.7761294672269));
#55450=CARTESIAN_POINT('Ctrl Pts',(18.4426739943933,71.3944589278792,11.7830692051441));
#55451=CARTESIAN_POINT('Ctrl Pts',(18.4380272384733,71.332589859076,11.7934451581334));
#55452=CARTESIAN_POINT('Ctrl Pts',(18.4333804825534,71.271570963609,11.8071630605646));
#55453=CARTESIAN_POINT('Ctrl Pts',(18.4287337266334,71.2105520681421,11.8208809629957));
#55454=CARTESIAN_POINT('Ctrl Pts',(18.4240869707134,71.1503838391696,11.8379406101307));
#55455=CARTESIAN_POINT('Ctrl Pts',(18.4194402147935,71.0914457198719,11.8581968199784));
#55456=CARTESIAN_POINT('Ctrl Pts',(18.4148360342462,71.0330476143894,11.878267434607));
#55457=CARTESIAN_POINT('Ctrl Pts',(18.4102318536989,70.9756262702442,11.9015555791544));
#55458=CARTESIAN_POINT('Ctrl Pts',(18.4056276731516,70.9195596795308,11.9279459591891));
#55459=CARTESIAN_POINT('Ctrl Pts',(18.4010154692609,70.8633953859784,11.9543823276639));
#55460=CARTESIAN_POINT('Ctrl Pts',(18.3964032653702,70.8085910710518,11.9839316321461));
#55461=CARTESIAN_POINT('Ctrl Pts',(18.3917910614795,70.755510637495,12.0164279315767));
#55462=CARTESIAN_POINT('Ctrl Pts',(18.3871991319811,70.7026635356731,12.0487813833058));
#55463=CARTESIAN_POINT('Ctrl Pts',(18.3826072024828,70.6515256397942,12.0840557332596));
#55464=CARTESIAN_POINT('Ctrl Pts',(18.3780152729844,70.6024330954231,12.1220404785168));
#55465=CARTESIAN_POINT('Ctrl Pts',(18.3734260563137,70.5533695540264,12.1600027830834));
#55466=CARTESIAN_POINT('Ctrl Pts',(18.3688368396431,70.5063493680446,12.2006719975531));
#55467=CARTESIAN_POINT('Ctrl Pts',(18.3642476229724,70.4616785664782,12.2437951217594));
#55468=CARTESIAN_POINT('Ctrl Pts',(18.3596594472243,70.4170178971089,12.2869084648116));
#55469=CARTESIAN_POINT('Ctrl Pts',(18.3550712714763,70.3747059186949,12.3324742602312));
#55470=CARTESIAN_POINT('Ctrl Pts',(18.3504830957282,70.3350129845232,12.3802015299746));
#55471=CARTESIAN_POINT('Ctrl Pts',(18.3458540693988,70.2949666464002,12.4283537369533));
#55472=CARTESIAN_POINT('Ctrl Pts',(18.3412250430693,70.2575865832869,12.4787057181409));
#55473=CARTESIAN_POINT('Ctrl Pts',(18.3365960167399,70.2231085072819,12.5309250587191));
#55474=CARTESIAN_POINT('Ctrl Pts',(18.3320021303128,70.188892161528,12.5827479914142));
#55475=CARTESIAN_POINT('Ctrl Pts',(18.3274082438856,70.1575341048607,12.6364095570815));
#55476=CARTESIAN_POINT('Ctrl Pts',(18.3228143574585,70.1292194430487,12.6915583809155));
#55477=CARTESIAN_POINT('Ctrl Pts',(18.3181677611779,70.1005799012685,12.7473399775601));
#55478=CARTESIAN_POINT('Ctrl Pts',(18.3135211648973,70.075054270936,12.8046427001273));
#55479=CARTESIAN_POINT('Ctrl Pts',(18.3088745686167,70.052783830391,12.8630827305967));
#55480=CARTESIAN_POINT('Ctrl Pts',(18.304227972336,70.030513389846,12.9215227610661));
#55481=CARTESIAN_POINT('Ctrl Pts',(18.2995813760554,70.0114982408165,12.9810995754133));
#55482=CARTESIAN_POINT('Ctrl Pts',(18.2949347797748,69.9958269593481,13.0414167301978));
#55483=CARTESIAN_POINT('Ctrl Pts',(18.2903306132046,69.9802987778814,13.1011831077552));
#55484=CARTESIAN_POINT('Ctrl Pts',(18.2857264466345,69.9679922107812,13.1619126164308));
#55485=CARTESIAN_POINT('Ctrl Pts',(18.2811222800644,69.9590199518388,13.2232264828556));
#55486=CARTESIAN_POINT('Ctrl Pts',(18.2765100744265,69.9500320269564,13.2846474058598));
#55487=CARTESIAN_POINT('Ctrl Pts',(18.2718978687887,69.9443902391824,13.3466542458907));
#55488=CARTESIAN_POINT('Ctrl Pts',(18.2672856631508,69.9421572818739,13.4088519930779));
#55489=CARTESIAN_POINT('Ctrl Pts',(18.2626937476903,69.9399341478698,13.4707761177468));
#55490=CARTESIAN_POINT('Ctrl Pts',(18.2581018322298,69.9410899606479,13.5328889657477));
#55491=CARTESIAN_POINT('Ctrl Pts',(18.2535099167693,69.9456349339227,13.594794053317));
#55492=CARTESIAN_POINT('Ctrl Pts',(18.2489207141178,69.950177222121,13.6566625686368));
#55493=CARTESIAN_POINT('Ctrl Pts',(18.2443315114663,69.9581046628539,13.7183230621107));
#55494=CARTESIAN_POINT('Ctrl Pts',(18.2397423088148,69.969375408636,13.7793806793307));
#55495=CARTESIAN_POINT('Ctrl Pts',(18.2351541470425,69.980643598095,13.8404244480443));
#55496=CARTESIAN_POINT('Ctrl Pts',(18.2305659852702,69.9952534947683,13.9008651135017));
#55497=CARTESIAN_POINT('Ctrl Pts',(18.2259778234979,70.0131118863953,13.9603165811849));
#55498=CARTESIAN_POINT('Ctrl Pts',(18.2213487836027,70.0311293869559,14.0202977303658));
#55499=CARTESIAN_POINT('Ctrl Pts',(18.2167197437076,70.0524534378522,14.079271455703));
#55500=CARTESIAN_POINT('Ctrl Pts',(18.2120907038124,70.0769371474875,14.1368576428956));
#55501=CARTESIAN_POINT('Ctrl Pts',(18.2074968310886,70.1012348525017,14.1940063434048));
#55502=CARTESIAN_POINT('Ctrl Pts',(18.2029029583647,70.1286440947259,14.2497880797131));
#55503=CARTESIAN_POINT('Ctrl Pts',(18.1983090856409,70.1589742257078,14.3038544555975));
#55504=CARTESIAN_POINT('Ctrl Pts',(18.1936624621601,70.1896526330711,14.358541667632));
#55505=CARTESIAN_POINT('Ctrl Pts',(18.1890158386793,70.2233191661855,14.4114734152918));
#55506=CARTESIAN_POINT('Ctrl Pts',(18.1843692151985,70.2597319159975,14.4623199063693));
#55507=CARTESIAN_POINT('Ctrl Pts',(18.1797225917176,70.2961446658095,14.5131663974469));
#55508=CARTESIAN_POINT('Ctrl Pts',(18.1750759682368,70.3353032516732,14.5619272576588));
#55509=CARTESIAN_POINT('Ctrl Pts',(18.170429344756,70.3769261265954,14.6083096538684));
#55510=CARTESIAN_POINT('Ctrl Pts',(18.1658930358871,70.4175608406918,14.6535908943545));
#55511=CARTESIAN_POINT('Ctrl Pts',(18.1613567270183,70.4607151649762,14.6967956968842));
#55512=CARTESIAN_POINT('Ctrl Pts',(18.1568204181494,70.5061456764191,14.7376255053454));
#55513=CARTESIAN_POINT('Ctrl Pts',(18.1522901777964,70.5515154125083,14.7784006931129));
#55514=CARTESIAN_POINT('Ctrl Pts',(18.1477599374433,70.5991549214016,14.8168068308777));
#55515=CARTESIAN_POINT('Ctrl Pts',(18.1432296970902,70.6487820235391,14.8525799957308));
#55516=CARTESIAN_POINT('Ctrl Pts',(18.1387037497788,70.6983620969985,14.8883192604652));
#55517=CARTESIAN_POINT('Ctrl Pts',(18.1341778024674,70.7499256102087,14.9214301901394));
#55518=CARTESIAN_POINT('Ctrl Pts',(18.1296518551559,70.8031568754621,14.9516886834854));
#55519=CARTESIAN_POINT('Ctrl Pts',(18.125128431986,70.8563584533952,14.9819303015311));
#55520=CARTESIAN_POINT('Ctrl Pts',(18.1206050088161,70.9112254852309,15.0093223788357));
#55521=CARTESIAN_POINT('Ctrl Pts',(18.1160815856462,70.9674147263675,15.0336850080299));
#55522=CARTESIAN_POINT('Ctrl Pts',(18.1115565317005,71.023624224741,15.0580564203922));
#55523=CARTESIAN_POINT('Ctrl Pts',(18.1070314777548,71.0811564091793,15.0793959821789));
#55524=CARTESIAN_POINT('Ctrl Pts',(18.1025064238091,71.1396464212039,15.0975712436434));
#55525=CARTESIAN_POINT('Ctrl Pts',(18.0979807351458,71.1981446374715,15.1157490545049));
#55526=CARTESIAN_POINT('Ctrl Pts',(18.0934550464825,71.2576004434866,15.1307615418621));
#55527=CARTESIAN_POINT('Ctrl Pts',(18.0889293578192,71.317634974436,15.1425265090925));
#55528=CARTESIAN_POINT('Ctrl Pts',(18.0843973318221,71.3777535718965,15.1543079508373));
#55529=CARTESIAN_POINT('Ctrl Pts',(18.0798653058251,71.4384519944004,15.1628327089221));
#55530=CARTESIAN_POINT('Ctrl Pts',(18.0753332798281,71.4993436244346,15.1680701901737));
#55531=CARTESIAN_POINT('Ctrl Pts',(18.0716838814238,71.5483764008631,15.1722876540045));
#55532=CARTESIAN_POINT('Ctrl Pts',(18.0680344830195,71.5975342312904,15.1743745799587));
#55533=CARTESIAN_POINT('Ctrl Pts',(18.0643850846152,71.6466158347437,15.1743395663265));
#55534=CARTESIAN_POINT('',(17.2706350845291,71.6439433034762,15.1743393774819));
#55535=CARTESIAN_POINT('Ctrl Pts',(18.0643850845702,71.6466158353495,15.174339566326));
#55536=CARTESIAN_POINT('Ctrl Pts',(18.0582313596258,71.7293787058325,15.1742805252608));
#55537=CARTESIAN_POINT('Ctrl Pts',(18.0520776346815,71.8119254455953,15.168191932043));
#55538=CARTESIAN_POINT('Ctrl Pts',(18.0459239097372,71.8935789255846,15.1561737919016));
#55539=CARTESIAN_POINT('Ctrl Pts',(18.0413197449804,71.9546713660552,15.1471819214845));
#55540=CARTESIAN_POINT('Ctrl Pts',(18.0367155802237,72.0153952534079,15.1348478116356));
#55541=CARTESIAN_POINT('Ctrl Pts',(18.0321114154669,72.0753578439467,15.1192152946261));
#55542=CARTESIAN_POINT('Ctrl Pts',(18.0274992096024,72.1354251582903,15.1035554756498));
#55543=CARTESIAN_POINT('Ctrl Pts',(18.0228870037379,72.1947280011364,15.0845857452346));
#55544=CARTESIAN_POINT('Ctrl Pts',(18.0182747978734,72.2528781616959,15.0624023105555));
#55545=CARTESIAN_POINT('Ctrl Pts',(18.0136828845006,72.3107724768554,15.0403164771498));
#55546=CARTESIAN_POINT('Ctrl Pts',(18.0090909711279,72.3675237460416,15.0150453146395));
#55547=CARTESIAN_POINT('Ctrl Pts',(18.0044990577551,72.4227628540532,14.9867339347223));
#55548=CARTESIAN_POINT('Ctrl Pts',(17.9999098572888,72.4779693267521,14.9584392811928));
#55549=CARTESIAN_POINT('Ctrl Pts',(17.9953206568224,72.5316649595835,14.9271082033252));
#55550=CARTESIAN_POINT('Ctrl Pts',(17.990731456356,72.58350242719,14.8929331227082));
#55551=CARTESIAN_POINT('Ctrl Pts',(17.9861432968626,72.6353281364512,14.8587657940595));
#55552=CARTESIAN_POINT('Ctrl Pts',(17.9815551373692,72.6852960942193,14.821756022743));
#55553=CARTESIAN_POINT('Ctrl Pts',(17.9769669778758,72.7330870603228,14.7821401199591));
#55554=CARTESIAN_POINT('Ctrl Pts',(17.972337935946,72.7813038640928,14.7421712227713));
#55555=CARTESIAN_POINT('Ctrl Pts',(17.9677088940163,72.8273042616491,14.6995498271725));
#55556=CARTESIAN_POINT('Ctrl Pts',(17.9630798520865,72.8707954393377,14.654559349653));
#55557=CARTESIAN_POINT('Ctrl Pts',(17.9584859818468,72.9139561689018,14.6099107120125));
#55558=CARTESIAN_POINT('Ctrl Pts',(17.9538921116071,72.9546453847161,14.5629292956482));
#55559=CARTESIAN_POINT('Ctrl Pts',(17.9492982413675,72.992616537172,14.5139264521844));
#55560=CARTESIAN_POINT('Ctrl Pts',(17.9446516135926,73.0310237629836,14.4643608437529));
#55561=CARTESIAN_POINT('Ctrl Pts',(17.9400049858178,73.0666497805645,14.412727510831));
#55562=CARTESIAN_POINT('Ctrl Pts',(17.935358358043,73.0992851498073,14.3593777638157));
#55563=CARTESIAN_POINT('Ctrl Pts',(17.9307117302681,73.1319205190501,14.3060280168005));
#55564=CARTESIAN_POINT('Ctrl Pts',(17.9260651024933,73.1615650436088,14.2509623521114));
#55565=CARTESIAN_POINT('Ctrl Pts',(17.9214184747185,73.1880587682366,14.1945541804328));
#55566=CARTESIAN_POINT('Ctrl Pts',(17.9168143123683,73.2143103673228,14.1386615217411));
#55567=CARTESIAN_POINT('Ctrl Pts',(17.9122101500181,73.2375723488741,14.0812298510895));
#55568=CARTESIAN_POINT('Ctrl Pts',(17.9076059876679,73.2576643014475,14.0226107652569));
#55569=CARTESIAN_POINT('Ctrl Pts',(17.9029937815025,73.2777913561613,13.9638892675077));
#55570=CARTESIAN_POINT('Ctrl Pts',(17.8983815753372,73.2947370347143,13.903976644647));
#55571=CARTESIAN_POINT('Ctrl Pts',(17.8937693691718,73.3083670882121,13.8432496471843));
#55572=CARTESIAN_POINT('Ctrl Pts',(17.8891774582468,73.3219371649438,13.782789868697));
#55573=CARTESIAN_POINT('Ctrl Pts',(17.8845855473217,73.3322205966582,13.7215233581769));
#55574=CARTESIAN_POINT('Ctrl Pts',(17.8799936363967,73.3391344489828,13.6598379622963));
#55575=CARTESIAN_POINT('Ctrl Pts',(17.8754044383863,73.3460442165829,13.5981890103313));
#55576=CARTESIAN_POINT('Ctrl Pts',(17.8708152403759,73.3495882965235,13.5361221668568));
#55577=CARTESIAN_POINT('Ctrl Pts',(17.8662260423655,73.3497352277371,13.4740332486111));
#55578=CARTESIAN_POINT('Ctrl Pts',(17.861637885332,73.3498821256219,13.4119584141191));
#55579=CARTESIAN_POINT('Ctrl Pts',(17.8570497282986,73.3466334037854,13.3498620217563));
#55580=CARTESIAN_POINT('Ctrl Pts',(17.8524615712652,73.3400097008886,13.2881407212866));
#55581=CARTESIAN_POINT('Ctrl Pts',(17.8478325269681,73.3333269710045,13.2258693927622));
#55582=CARTESIAN_POINT('Ctrl Pts',(17.8432034826709,73.3232088298502,13.1639803994117));
#55583=CARTESIAN_POINT('Ctrl Pts',(17.8385744383738,73.3097297803731,13.1028743842182));
#55584=CARTESIAN_POINT('Ctrl Pts',(17.8339805705749,73.2963531593303,13.0422327187901));
#55585=CARTESIAN_POINT('Ctrl Pts',(17.8293867027759,73.2796667272973,12.9823626523723));
#55586=CARTESIAN_POINT('Ctrl Pts',(17.824792834977,73.2597938292486,12.9236416929487));
#55587=CARTESIAN_POINT('Ctrl Pts',(17.8201462024308,73.2396926729023,12.8642462699315));
#55588=CARTESIAN_POINT('Ctrl Pts',(17.8154995698846,73.2163315668755,12.8060270196675));
#55589=CARTESIAN_POINT('Ctrl Pts',(17.8108529373383,73.1898876650216,12.7493525909322));
#55590=CARTESIAN_POINT('Ctrl Pts',(17.8062063047921,73.1634437631677,12.692678162197));
#55591=CARTESIAN_POINT('Ctrl Pts',(17.8015596722459,73.1339173708365,12.637548992884));
#55592=CARTESIAN_POINT('Ctrl Pts',(17.7969130396997,73.1015313997032,12.5843046898631));
#55593=CARTESIAN_POINT('Ctrl Pts',(17.7923088783088,73.0694414428552,12.5315470504733));
#55594=CARTESIAN_POINT('Ctrl Pts',(17.787704716918,73.0344171462522,12.4804313641601));
#55595=CARTESIAN_POINT('Ctrl Pts',(17.7831005555272,72.9966519366625,12.4313022387308));
#55596=CARTESIAN_POINT('Ctrl Pts',(17.7784883492419,72.9588207395676,12.3820872695193));
#55597=CARTESIAN_POINT('Ctrl Pts',(17.7738761429566,72.9182392675481,12.3348662716024));
#55598=CARTESIAN_POINT('Ctrl Pts',(17.7692639366714,72.8751474151999,12.2899592674788));
#55599=CARTESIAN_POINT('Ctrl Pts',(17.7646720267685,72.8322451919921,12.245249880216));
#55600=CARTESIAN_POINT('Ctrl Pts',(17.7600801168656,72.7868549688105,12.2028345500411));
#55601=CARTESIAN_POINT('Ctrl Pts',(17.7554882069628,72.7392542355005,12.1629966537619));
#55602=CARTESIAN_POINT('Ctrl Pts',(17.7508990099952,72.6916816250661,12.123182294015));
#55603=CARTESIAN_POINT('Ctrl Pts',(17.7463098130277,72.6419014827485,12.0859426730579));
#55604=CARTESIAN_POINT('Ctrl Pts',(17.7417206160601,72.5902263756589,12.0515226630435));
#55605=CARTESIAN_POINT('Ctrl Pts',(17.7371324600885,72.538562990353,12.0171104607326));
#55606=CARTESIAN_POINT('Ctrl Pts',(17.7325443041168,72.4850059157838,11.9855168803209));
#55607=CARTESIAN_POINT('Ctrl Pts',(17.7279561481451,72.4298971930433,11.956943824669));
#55608=CARTESIAN_POINT('Ctrl Pts',(17.7233271028564,72.3742973453172,11.928116127994));
#55609=CARTESIAN_POINT('Ctrl Pts',(17.7186980575677,72.3171185046177,11.9023633335533));
#55610=CARTESIAN_POINT('Ctrl Pts',(17.7140690122791,72.2587357955364,11.8798446498805));
#55611=CARTESIAN_POINT('Ctrl Pts',(17.7094751455761,72.2007967678215,11.8574970977036));
#55612=CARTESIAN_POINT('Ctrl Pts',(17.7048812788732,72.1416726131983,11.8383347737319));
#55613=CARTESIAN_POINT('Ctrl Pts',(17.7002874121703,72.0817461508561,11.8224633927487));
#55614=CARTESIAN_POINT('Ctrl Pts',(17.6956407775887,72.0211313376109,11.8064097036665));
#55615=CARTESIAN_POINT('Ctrl Pts',(17.6909941430072,71.9596961851791,11.7937231678153));
#55616=CARTESIAN_POINT('Ctrl Pts',(17.6863475084256,71.8978458523827,11.7844597521225));
#55617=CARTESIAN_POINT('Ctrl Pts',(17.681700873844,71.8359955195862,11.7751963364298));
#55618=CARTESIAN_POINT('Ctrl Pts',(17.6770542392624,71.7737305401214,11.7693560282505));
#55619=CARTESIAN_POINT('Ctrl Pts',(17.6724076046809,71.711457140305,11.766940608841));
#55620=CARTESIAN_POINT('Ctrl Pts',(17.6678034421943,71.6497529442226,11.7645472673292));
#55621=CARTESIAN_POINT('Ctrl Pts',(17.6631992797078,71.5877965422259,11.7655069489137));
#55622=CARTESIAN_POINT('Ctrl Pts',(17.6585951172212,71.5259820415606,11.7698487753137));
#55623=CARTESIAN_POINT('Ctrl Pts',(17.6539829110729,71.4640595484134,11.7741981870636));
#55624=CARTESIAN_POINT('Ctrl Pts',(17.6493707049246,71.4022799622413,11.7819416392346));
#55625=CARTESIAN_POINT('Ctrl Pts',(17.6447584987763,71.3410425645745,11.7930559379928));
#55626=CARTESIAN_POINT('Ctrl Pts',(17.6401665877339,71.2800746300298,11.8041213304657));
#55627=CARTESIAN_POINT('Ctrl Pts',(17.6355746766914,71.2196446281494,11.8185279025853));
#55628=CARTESIAN_POINT('Ctrl Pts',(17.630982765649,71.1601420609145,11.8362008788855));
#55629=CARTESIAN_POINT('Ctrl Pts',(17.6263935675287,71.1006746480699,11.85386341391));
#55630=CARTESIAN_POINT('Ctrl Pts',(17.6218043694085,71.042134068444,11.8747883817577));
#55631=CARTESIAN_POINT('Ctrl Pts',(17.6172151712882,70.9848971036271,11.8988504974118));
#55632=CARTESIAN_POINT('Ctrl Pts',(17.6126270141526,70.9276731220817,11.9229071549676));
#55633=CARTESIAN_POINT('Ctrl Pts',(17.608038857017,70.871752635484,11.9500993507606));
#55634=CARTESIAN_POINT('Ctrl Pts',(17.6034506998815,70.8174928881701,11.9802534947913));
#55635=CARTESIAN_POINT('Ctrl Pts',(17.5988216556965,70.7627496088187,12.0106763554199));
#55636=CARTESIAN_POINT('Ctrl Pts',(17.5941926115116,70.7096972901596,12.0441139932849));
#55637=CARTESIAN_POINT('Ctrl Pts',(17.5895635673266,70.6586758618685,12.0803416567988));
#55638=CARTESIAN_POINT('Ctrl Pts',(17.5849696994459,70.6080421475871,12.1162940247525));
#55639=CARTESIAN_POINT('Ctrl Pts',(17.5803758315651,70.5594089306551,12.1549937960996));
#55640=CARTESIAN_POINT('Ctrl Pts',(17.5757819636844,70.513075800205,12.1961802552329));
#55641=CARTESIAN_POINT('Ctrl Pts',(17.5711353313473,70.4662104945812,12.2378397756686));
#55642=CARTESIAN_POINT('Ctrl Pts',(17.5664886990103,70.4216988390947,12.2820431089427));
#55643=CARTESIAN_POINT('Ctrl Pts',(17.5618420666732,70.3798112935905,12.328483437786));
#55644=CARTESIAN_POINT('Ctrl Pts',(17.5571954343362,70.3379237480864,12.3749237666293));
#55645=CARTESIAN_POINT('Ctrl Pts',(17.5525488019991,70.2986605968331,12.4236006391787));
#55646=CARTESIAN_POINT('Ctrl Pts',(17.5479021696621,70.2622477212206,12.474176416574));
#55647=CARTESIAN_POINT('Ctrl Pts',(17.5432980075383,70.2261676592415,12.5242899314329));
#55648=CARTESIAN_POINT('Ctrl Pts',(17.5386938454145,70.19274330371,12.5764658699009));
#55649=CARTESIAN_POINT('Ctrl Pts',(17.5340896832906,70.1622166324098,12.6303917975009));
#55650=CARTESIAN_POINT('Ctrl Pts',(17.529477477097,70.1316366270462,12.6844119407072));
#55651=CARTESIAN_POINT('Ctrl Pts',(17.5248652709034,70.1039647779175,12.7401878061276));
#55652=CARTESIAN_POINT('Ctrl Pts',(17.5202530647097,70.079402311737,12.7973737472007));
#55653=CARTESIAN_POINT('Ctrl Pts',(17.5156611540387,70.0549479300753,12.8543080476249));
#55654=CARTESIAN_POINT('Ctrl Pts',(17.5110692433677,70.033575850036,12.9126395832101));
#55655=CARTESIAN_POINT('Ctrl Pts',(17.5064773326966,70.01543889853,12.9720023661757));
#55656=CARTESIAN_POINT('Ctrl Pts',(17.5018881349499,69.9973126624277,13.0313300773053));
#55657=CARTESIAN_POINT('Ctrl Pts',(17.4972989372032,69.9824179121745,13.0916873434003));
#55658=CARTESIAN_POINT('Ctrl Pts',(17.4927097394565,69.9708583441007,13.1526908790182));
#55659=CARTESIAN_POINT('Ctrl Pts',(17.488121582696,69.9593013981304,13.2136805769583));
#55660=CARTESIAN_POINT('Ctrl Pts',(17.4835334259355,69.9510782264169,13.2753157552192));
#55661=CARTESIAN_POINT('Ctrl Pts',(17.478945269175,69.9462414668071,13.3372027309104));
#55662=CARTESIAN_POINT('Ctrl Pts',(17.4743162246307,69.9413616039661,13.3996412181158));
#55663=CARTESIAN_POINT('Ctrl Pts',(17.4696871800864,69.9399288858088,13.4623354931853));
#55664=CARTESIAN_POINT('Ctrl Pts',(17.4650581355421,69.9419437382228,13.5248780449002));
#55665=CARTESIAN_POINT('Ctrl Pts',(17.4604642680357,69.9439432793692,13.5869453232204));
#55666=CARTESIAN_POINT('Ctrl Pts',(17.4558704005294,69.9493380718814,13.6488626690757));
#55667=CARTESIAN_POINT('Ctrl Pts',(17.451276533023,69.9580762787708,13.7102363323419));
#55668=CARTESIAN_POINT('Ctrl Pts',(17.4466298999597,69.9669148534553,13.7723149387781));
#55669=CARTESIAN_POINT('Ctrl Pts',(17.4419832668965,69.979174050854,13.8338367681197));
#55670=CARTESIAN_POINT('Ctrl Pts',(17.4373366338332,69.9947475134842,13.8944068853816));
#55671=CARTESIAN_POINT('Ctrl Pts',(17.4326900007699,70.0103209761145,13.9549770026436));
#55672=CARTESIAN_POINT('Ctrl Pts',(17.4280433677066,70.0292084843387,14.0145949212571));
#55673=CARTESIAN_POINT('Ctrl Pts',(17.4233967346434,70.0512533634033,14.0728858404604));
#55674=CARTESIAN_POINT('Ctrl Pts',(17.4187925725859,70.0730967485747,14.1306439708823));
#55675=CARTESIAN_POINT('Ctrl Pts',(17.4141884105284,70.0981263312731,14.1873276189205));
#55676=CARTESIAN_POINT('Ctrl Pts',(17.4095842484709,70.1262153383897,14.2425624890765));
#55677=CARTESIAN_POINT('Ctrl Pts',(17.404972042269,70.1543534211097,14.2978938626284));
#55678=CARTESIAN_POINT('Ctrl Pts',(17.4003598360671,70.1855614920188,14.3517708958831));
#55679=CARTESIAN_POINT('Ctrl Pts',(17.3957476298651,70.2196625823213,14.4038349165837));
#55680=CARTESIAN_POINT('Ctrl Pts',(17.3911557192663,70.2536136138097,14.4556698341931));
#55681=CARTESIAN_POINT('Ctrl Pts',(17.3865638086674,70.2904320014151,14.5057072208433));
#55682=CARTESIAN_POINT('Ctrl Pts',(17.3819718980685,70.329897084498,14.5536175131963));
#55683=CARTESIAN_POINT('Ctrl Pts',(17.377382700396,70.3693388513904,14.6014994998822));
#55684=CARTESIAN_POINT('Ctrl Pts',(17.3727935027234,70.411423890793,14.6472564938737));
#55685=CARTESIAN_POINT('Ctrl Pts',(17.3682043050508,70.4558899835954,14.6905903311403));
#55686=CARTESIAN_POINT('Ctrl Pts',(17.3636161483663,70.5003459899565,14.7339143388002));
#55687=CARTESIAN_POINT('Ctrl Pts',(17.3590279916819,70.547181614122,14.7748159274075));
#55688=CARTESIAN_POINT('Ctrl Pts',(17.3544398349974,70.5960977654515,14.8130337509429));
#55689=CARTESIAN_POINT('Ctrl Pts',(17.349810790383,70.6454498391579,14.8515921573741));
#55690=CARTESIAN_POINT('Ctrl Pts',(17.3451817457686,70.6969193148219,14.8874183771893));
#55691=CARTESIAN_POINT('Ctrl Pts',(17.3405527011542,70.7501667331433,14.9202869486805));
#55692=CARTESIAN_POINT('Ctrl Pts',(17.3359588337275,70.8030095119357,14.9529057442445));
#55693=CARTESIAN_POINT('Ctrl Pts',(17.3313649663009,70.8576028253208,14.9826114933668));
#55694=CARTESIAN_POINT('Ctrl Pts',(17.3267710988743,70.9135898153586,15.0092299013647));
#55695=CARTESIAN_POINT('Ctrl Pts',(17.322124465666,70.9702198795248,15.0361540519916));
#55696=CARTESIAN_POINT('Ctrl Pts',(17.3174778324577,71.0282753545279,15.0599192682865));
#55697=CARTESIAN_POINT('Ctrl Pts',(17.3128311992494,71.087368277907,15.0803960484111));
#55698=CARTESIAN_POINT('Ctrl Pts',(17.3081845660411,71.1464612012861,15.1008728285356));
#55699=CARTESIAN_POINT('Ctrl Pts',(17.3035379328328,71.2065910461191,15.1180610867985));
#55700=CARTESIAN_POINT('Ctrl Pts',(17.2988912996246,71.2673588385453,15.1318843870276));
#55701=CARTESIAN_POINT('Ctrl Pts',(17.2927452767469,71.3477353661799,15.1501682316186));
#55702=CARTESIAN_POINT('Ctrl Pts',(17.2865992538693,71.429481789506,15.1626267077974));
#55703=CARTESIAN_POINT('Ctrl Pts',(17.2804532309918,71.5118776892291,15.1691017121192));
#55704=CARTESIAN_POINT('Ctrl Pts',(17.2771805155179,71.5557529466724,15.1725496079795));
#55705=CARTESIAN_POINT('Ctrl Pts',(17.273907800044,71.5998120318739,15.1743016585303));
#55706=CARTESIAN_POINT('Ctrl Pts',(17.2706350845702,71.6439433029223,15.1743393774814));
#55707=CARTESIAN_POINT('',(16.4768850845224,71.6462429261512,15.1743397915543));
#55708=CARTESIAN_POINT('Ctrl Pts',(17.2706350845291,71.6439433034762,15.1743393774819));
#55709=CARTESIAN_POINT('Ctrl Pts',(17.2661002318933,71.7050939939149,15.1743916428929));
#55710=CARTESIAN_POINT('Ctrl Pts',(17.2615653792575,71.7663362412798,15.1711485740932));
#55711=CARTESIAN_POINT('Ctrl Pts',(17.2570305266217,71.8272822897832,15.1646072312672));
#55712=CARTESIAN_POINT('Ctrl Pts',(17.2524990686935,71.8881827151916,15.1580707851707));
#55713=CARTESIAN_POINT('Ctrl Pts',(17.2479676107653,71.9487868638439,15.1482410117791));
#55714=CARTESIAN_POINT('Ctrl Pts',(17.2434361528371,72.0087094547258,15.1351669813286));
#55715=CARTESIAN_POINT('Ctrl Pts',(17.2389063309392,72.0686104112505,15.1220976711053));
#55716=CARTESIAN_POINT('Ctrl Pts',(17.2343765090414,72.127829788608,15.1057865376919));
#55717=CARTESIAN_POINT('Ctrl Pts',(17.2298466871436,72.1859920963689,15.0863338210108));
#55718=CARTESIAN_POINT('Ctrl Pts',(17.2252249519321,72.2453345587928,15.066486394849));
#55719=CARTESIAN_POINT('Ctrl Pts',(17.2206032167206,72.3035760300047,15.0433686108237));
#55720=CARTESIAN_POINT('Ctrl Pts',(17.2159814815091,72.360335913905,15.0171397721631));
#55721=CARTESIAN_POINT('Ctrl Pts',(17.2114468974667,72.4160254876279,14.9914055256516));
#55722=CARTESIAN_POINT('Ctrl Pts',(17.2069123134242,72.4702884285972,14.9626768547615));
#55723=CARTESIAN_POINT('Ctrl Pts',(17.2023777293817,72.5227897819664,14.9311509183178));
#55724=CARTESIAN_POINT('Ctrl Pts',(17.1977124185857,72.5768046879385,14.8987161260046));
#55725=CARTESIAN_POINT('Ctrl Pts',(17.1930471077898,72.6289543599915,14.8633205988426));
#55726=CARTESIAN_POINT('Ctrl Pts',(17.1883817969938,72.6789081830433,14.8252253211856));
#55727=CARTESIAN_POINT('Ctrl Pts',(17.1837164861978,72.7288620060951,14.7871300435286));
#55728=CARTESIAN_POINT('Ctrl Pts',(17.1790511754018,72.7766195769644,14.7463354566648));
#55729=CARTESIAN_POINT('Ctrl Pts',(17.1743858646058,72.8218914468588,14.7031434268032));
#55730=CARTESIAN_POINT('Ctrl Pts',(17.1697817024763,72.866569934106,14.6605175189304));
#55731=CARTESIAN_POINT('Ctrl Pts',(17.1651775403467,72.9090171636797,14.6153760878356));
#55732=CARTESIAN_POINT('Ctrl Pts',(17.1605733782172,72.9489378409919,14.5679817542665));
#55733=CARTESIAN_POINT('Ctrl Pts',(17.1559611720242,72.9889282648613,14.5205046167016));
#55734=CARTESIAN_POINT('Ctrl Pts',(17.1513489658313,73.026382897014,14.4707670160188));
#55735=CARTESIAN_POINT('Ctrl Pts',(17.1467367596384,73.0610403932004,14.4190717110626));
#55736=CARTESIAN_POINT('Ctrl Pts',(17.1421448489636,73.0955453827958,14.3676038857457));
#55737=CARTESIAN_POINT('Ctrl Pts',(17.1375529382889,73.1272774953741,14.314195956707));
#55738=CARTESIAN_POINT('Ctrl Pts',(17.1329610276141,73.1560192217013,14.2591795756521));
#55739=CARTESIAN_POINT('Ctrl Pts',(17.1283718298645,73.1847439672648,14.2041956985659));
#55740=CARTESIAN_POINT('Ctrl Pts',(17.1237826321148,73.2104815960163,14.1476057027431));
#55741=CARTESIAN_POINT('Ctrl Pts',(17.1191934343652,73.2330597116227,14.0897672754269));
#55742=CARTESIAN_POINT('Ctrl Pts',(17.1146052776025,73.2556327057403,14.0319419678443));
#55743=CARTESIAN_POINT('Ctrl Pts',(17.1100171208399,73.2750474255411,13.9728692633669));
#55744=CARTESIAN_POINT('Ctrl Pts',(17.1054289640772,73.2911797512475,13.9129264566309));
#55745=CARTESIAN_POINT('Ctrl Pts',(17.1007999195364,73.3074558416485,13.8524494640956));
#55746=CARTESIAN_POINT('Ctrl Pts',(17.0961708749955,73.320390574276,13.7910872811148));
#55747=CARTESIAN_POINT('Ctrl Pts',(17.0915418304546,73.3299086089493,13.7292403941818));
#55748=CARTESIAN_POINT('Ctrl Pts',(17.0869479629481,73.3393543141755,13.6678634940993));
#55749=CARTESIAN_POINT('Ctrl Pts',(17.0823540954416,73.3454350780737,13.6060097486663));
#55750=CARTESIAN_POINT('Ctrl Pts',(17.0777602279351,73.3481294624658,13.5440757264631));
#55751=CARTESIAN_POINT('Ctrl Pts',(17.073113594877,73.3508547947852,13.4814303248322));
#55752=CARTESIAN_POINT('Ctrl Pts',(17.068466961819,73.350115447916,13.4187033228594));
#55753=CARTESIAN_POINT('Ctrl Pts',(17.063820328761,73.34594335698,13.3563024774627));
#55754=CARTESIAN_POINT('Ctrl Pts',(17.059173695703,73.3417712660441,13.2939016320661));
#55755=CARTESIAN_POINT('Ctrl Pts',(17.054527062645,73.3341665574789,13.231827461901));
#55756=CARTESIAN_POINT('Ctrl Pts',(17.049880429587,73.323214327678,13.1704771837765));
#55757=CARTESIAN_POINT('Ctrl Pts',(17.0452762674587,73.3123622029157,13.109687656483));
#55758=CARTESIAN_POINT('Ctrl Pts',(17.0406721053303,73.2981806471449,13.049368508845));
#55759=CARTESIAN_POINT('Ctrl Pts',(17.036067943202,73.2807254577291,12.9899109635671));
#55760=CARTESIAN_POINT('Ctrl Pts',(17.0314557370089,73.2632397718473,12.9303495382931));
#55761=CARTESIAN_POINT('Ctrl Pts',(17.0268435308159,73.2424690460747,12.8716532407826));
#55762=CARTESIAN_POINT('Ctrl Pts',(17.0222313246228,73.2185212901781,12.8142071653422));
#55763=CARTESIAN_POINT('Ctrl Pts',(17.0176394139498,73.1946789138198,12.7570138752125));
#55764=CARTESIAN_POINT('Ctrl Pts',(17.0130475032767,73.1676875793589,12.7010603077331));
#55765=CARTESIAN_POINT('Ctrl Pts',(17.0084555926037,73.1377035953588,12.6467109773116));
#55766=CARTESIAN_POINT('Ctrl Pts',(17.003866394856,73.1077373260562,12.592393756764));
#55767=CARTESIAN_POINT('Ctrl Pts',(16.9992771971082,73.0747821582154,12.5396793368136));
#55768=CARTESIAN_POINT('Ctrl Pts',(16.9946879993605,73.0390410232761,12.4889090083779));
#55769=CARTESIAN_POINT('Ctrl Pts',(16.9900998425999,73.0033079956498,12.438150196391));
#55770=CARTESIAN_POINT('Ctrl Pts',(16.9855116858393,72.9647905476703,12.389335014758));
#55771=CARTESIAN_POINT('Ctrl Pts',(16.9809235290787,72.9237346228418,12.3427753428691));
#55772=CARTESIAN_POINT('Ctrl Pts',(16.9762944845362,72.8823128243542,12.2958007501718));
#55773=CARTESIAN_POINT('Ctrl Pts',(16.9716654399937,72.8383074005824,12.2511224837385));
#55774=CARTESIAN_POINT('Ctrl Pts',(16.9670363954511,72.7920105729229,12.2090245721421));
#55775=CARTESIAN_POINT('Ctrl Pts',(16.9624425279471,72.746065564148,12.1672465710244));
#55776=CARTESIAN_POINT('Ctrl Pts',(16.957848660443,72.6978642923282,12.1280101223236));
#55777=CARTESIAN_POINT('Ctrl Pts',(16.9532547929389,72.6477254880847,12.0915521585726));
#55778=CARTESIAN_POINT('Ctrl Pts',(16.9486081598772,72.5970107852183,12.0546754355107));
#55779=CARTESIAN_POINT('Ctrl Pts',(16.9439615268154,72.5443141943564,12.0206417355799));
#55780=CARTESIAN_POINT('Ctrl Pts',(16.9393148937536,72.4899932556133,11.9896496805916));
#55781=CARTESIAN_POINT('Ctrl Pts',(16.9346682606918,72.4356723168703,11.9586576256034));
#55782=CARTESIAN_POINT('Ctrl Pts',(16.9300216276301,72.3797275324318,11.9307073966637));
#55783=CARTESIAN_POINT('Ctrl Pts',(16.9253749945683,72.3225370223109,11.9059474789458));
#55784=CARTESIAN_POINT('Ctrl Pts',(16.9207708324282,72.265869242013,11.8814138705821));
#55785=CARTESIAN_POINT('Ctrl Pts',(16.9161666702881,72.2077544052792,11.8599154550731));
#55786=CARTESIAN_POINT('Ctrl Pts',(16.9115625081481,72.1485494509366,11.8416218296654));
#55787=CARTESIAN_POINT('Ctrl Pts',(16.9069503019565,72.0892410580769,11.8232962429885));
#55788=CARTESIAN_POINT('Ctrl Pts',(16.9023380957649,72.0288391855924,11.8081869018611));
#55789=CARTESIAN_POINT('Ctrl Pts',(16.8977258895733,71.9677245055836,11.796416494853));
#55790=CARTESIAN_POINT('Ctrl Pts',(16.8931339788878,71.9068787540043,11.7846978822266));
#55791=CARTESIAN_POINT('Ctrl Pts',(16.8885420682024,71.8453269495663,11.7762890035574));
#55792=CARTESIAN_POINT('Ctrl Pts',(16.883950157517,71.7834592892696,11.7712609181377));
#55793=CARTESIAN_POINT('Ctrl Pts',(16.8793609597567,71.7216281807133,11.7662358033374));
#55794=CARTESIAN_POINT('Ctrl Pts',(16.8747717619964,71.6594820909183,11.7645875615234));
#55795=CARTESIAN_POINT('Ctrl Pts',(16.8701825642361,71.5974176123591,11.766335559426));
#55796=CARTESIAN_POINT('Ctrl Pts',(16.8655944074627,71.5353672121461,11.768083160823));
#55797=CARTESIAN_POINT('Ctrl Pts',(16.8610062506894,71.4733988931653,11.7732254578535));
#55798=CARTESIAN_POINT('Ctrl Pts',(16.8564180939161,71.4119084905315,11.7817297163647));
#55799=CARTESIAN_POINT('Ctrl Pts',(16.8517890493855,71.3498701108388,11.7903097613135));
#55800=CARTESIAN_POINT('Ctrl Pts',(16.847160004855,71.2883187317408,11.8023119494799));
#55801=CARTESIAN_POINT('Ctrl Pts',(16.8425309603244,71.2276525359906,11.8176495856164));
#55802=CARTESIAN_POINT('Ctrl Pts',(16.8379370928073,71.1674473545104,11.8328706680603));
#55803=CARTESIAN_POINT('Ctrl Pts',(16.8333432252902,71.1081144229225,11.8513764714748));
#55804=CARTESIAN_POINT('Ctrl Pts',(16.8287493577731,71.0500273090466,11.8730321874042));
#55805=CARTESIAN_POINT('Ctrl Pts',(16.8241027247359,70.9912730020554,11.8949366425739));
#55806=CARTESIAN_POINT('Ctrl Pts',(16.8194560916986,70.9337938089614,11.920063634761));
#55807=CARTESIAN_POINT('Ctrl Pts',(16.8148094586613,70.8779528005222,11.9482248419646));
#55808=CARTESIAN_POINT('Ctrl Pts',(16.810162825624,70.8221117920829,11.9763860491682));
#55809=CARTESIAN_POINT('Ctrl Pts',(16.8055161925867,70.7679093966695,12.0075811528165));
#55810=CARTESIAN_POINT('Ctrl Pts',(16.8008695595495,70.7156782601852,12.0415769806826));
#55811=CARTESIAN_POINT('Ctrl Pts',(16.7962653974163,70.6639245239118,12.0752620817202));
#55812=CARTESIAN_POINT('Ctrl Pts',(16.7916612352832,70.613901528645,12.1118300465224));
#55813=CARTESIAN_POINT('Ctrl Pts',(16.7870570731501,70.5659478186091,12.1510770213199));
#55814=CARTESIAN_POINT('Ctrl Pts',(16.7824448669576,70.5179103273163,12.1903925655956));
#55815=CARTESIAN_POINT('Ctrl Pts',(16.7778326607652,70.471949813175,12.2323962503146));
#55816=CARTESIAN_POINT('Ctrl Pts',(16.7732204545727,70.4283788282358,12.2768385259833));
#55817=CARTESIAN_POINT('Ctrl Pts',(16.7686285438945,70.3849995727013,12.3210852382268));
#55818=CARTESIAN_POINT('Ctrl Pts',(16.7640366332163,70.3439892368291,12.3677487808467));
#55819=CARTESIAN_POINT('Ctrl Pts',(16.7594447225381,70.3056225968613,12.4165431448612));
#55820=CARTESIAN_POINT('Ctrl Pts',(16.7548555247851,70.2672786241075,12.4653086809071));
#55821=CARTESIAN_POINT('Ctrl Pts',(16.7502663270321,70.2315755625268,12.5162021437496));
#55822=CARTESIAN_POINT('Ctrl Pts',(16.745677129279,70.1987486311264,12.5689036385956));
#55823=CARTESIAN_POINT('Ctrl Pts',(16.741088972513,70.1659291459973,12.6215931789393));
#55824=CARTESIAN_POINT('Ctrl Pts',(16.7365008157471,70.1359847635496,12.6760895065633));
#55825=CARTESIAN_POINT('Ctrl Pts',(16.7319126589811,70.1091068540045,12.7320445777913));
#55826=CARTESIAN_POINT('Ctrl Pts',(16.7272836144436,70.0819894195517,12.7884982976678));
#55827=CARTESIAN_POINT('Ctrl Pts',(16.722654569906,70.0579936425927,12.8464364326991));
#55828=CARTESIAN_POINT('Ctrl Pts',(16.7180255253685,70.0372672091046,12.905479174479));
#55829=CARTESIAN_POINT('Ctrl Pts',(16.7134316578588,70.0166982798967,12.9640732387497));
#55830=CARTESIAN_POINT('Ctrl Pts',(16.7088377903492,69.9993492646001,13.0237546695944));
#55831=CARTESIAN_POINT('Ctrl Pts',(16.7042439228395,69.9853141456875,13.0841375997697));
#55832=CARTESIAN_POINT('Ctrl Pts',(16.699597289788,69.9711178182393,13.1452140932704));
#55833=CARTESIAN_POINT('Ctrl Pts',(16.6949506567366,69.960312108809,13.2070077826231));
#55834=CARTESIAN_POINT('Ctrl Pts',(16.6903040236851,69.9529405933612,13.2691119902036));
#55835=CARTESIAN_POINT('Ctrl Pts',(16.6856573906336,69.9455690779134,13.3312161977841));
#55836=CARTESIAN_POINT('Ctrl Pts',(16.6810107575821,69.9416317275215,13.3936303905322));
#55837=CARTESIAN_POINT('Ctrl Pts',(16.6763641245307,69.9411179252497,13.455948477487));
#55838=CARTESIAN_POINT('Ctrl Pts',(16.6717599623902,69.9406088192064,13.5176969679418));
#55839=CARTESIAN_POINT('Ctrl Pts',(16.6671558002497,69.9434588708166,13.5795952177));
#55840=CARTESIAN_POINT('Ctrl Pts',(16.6625516381092,69.9496851607163,13.6412484143963));
#55841=CARTESIAN_POINT('Ctrl Pts',(16.6579394319176,69.9559223287286,13.703009326991));
#55842=CARTESIAN_POINT('Ctrl Pts',(16.653327225726,69.9655475949764,13.7645238182712));
#55843=CARTESIAN_POINT('Ctrl Pts',(16.6487150195345,69.9785255909888,13.8253935004803));
#55844=CARTESIAN_POINT('Ctrl Pts',(16.6441231088489,69.9914464787575,13.885995332349));
#55845=CARTESIAN_POINT('Ctrl Pts',(16.6395311981633,70.0076905724707,13.9459575145064));
#55846=CARTESIAN_POINT('Ctrl Pts',(16.6349392874778,70.0271712445152,14.0048930084812));
#55847=CARTESIAN_POINT('Ctrl Pts',(16.6303500897174,70.0466404072753,14.0637936830536));
#55848=CARTESIAN_POINT('Ctrl Pts',(16.625760891957,70.0693421972098,14.121668391791));
#55849=CARTESIAN_POINT('Ctrl Pts',(16.6211716941966,70.0951398888881,14.1781443521594));
#55850=CARTESIAN_POINT('Ctrl Pts',(16.6165835374232,70.1209317287671,14.2346075018473));
#55851=CARTESIAN_POINT('Ctrl Pts',(16.6119953806499,70.1498178652253,14.2896720720946));
#55852=CARTESIAN_POINT('Ctrl Pts',(16.6074072238766,70.1816138865965,14.3429862827142));
#55853=CARTESIAN_POINT('Ctrl Pts',(16.6027781793462,70.2136932609703,14.3967756075465));
#55854=CARTESIAN_POINT('Ctrl Pts',(16.5981491348158,70.2487344032401,14.448782752615));
#55855=CARTESIAN_POINT('Ctrl Pts',(16.5935200902854,70.2865022922881,14.498674805551));
#55856=CARTESIAN_POINT('Ctrl Pts',(16.5889262227686,70.3239831757702,14.5481877190316));
#55857=CARTESIAN_POINT('Ctrl Pts',(16.5843323552518,70.3641491303437,14.5956172206556));
#55858=CARTESIAN_POINT('Ctrl Pts',(16.5797384877349,70.4067304188606,14.6406718175304));
#55859=CARTESIAN_POINT('Ctrl Pts',(16.5750918546977,70.4498007993759,14.6862439150163));
#55860=CARTESIAN_POINT('Ctrl Pts',(16.5704452216606,70.4953419787245,14.7293858245651));
#55861=CARTESIAN_POINT('Ctrl Pts',(16.5657985886234,70.5430390283343,14.7698365757849));
#55862=CARTESIAN_POINT('Ctrl Pts',(16.5611519555862,70.5907360779441,14.8102873270047));
#55863=CARTESIAN_POINT('Ctrl Pts',(16.5565053225491,70.6405885374863,14.848046649549));
#55864=CARTESIAN_POINT('Ctrl Pts',(16.5518586895119,70.6922520315995,14.8828990713898));
#55865=CARTESIAN_POINT('Ctrl Pts',(16.5471911926695,70.7441474995034,14.9179079837766));
#55866=CARTESIAN_POINT('Ctrl Pts',(16.5425236958271,70.7980717651909,14.9501199881615));
#55867=CARTESIAN_POINT('Ctrl Pts',(16.5378561989847,70.8536966037079,14.9792980381288));
#55868=CARTESIAN_POINT('Ctrl Pts',(16.5331963030289,70.9092308587477,15.0084285724666));
#55869=CARTESIAN_POINT('Ctrl Pts',(16.5285364070732,70.9664597606,15.0345347338153));
#55870=CARTESIAN_POINT('Ctrl Pts',(16.5238765111174,71.02502660324,15.0574229695303));
#55871=CARTESIAN_POINT('Ctrl Pts',(16.5192236139525,71.0835054831689,15.0802768289468));
#55872=CARTESIAN_POINT('Ctrl Pts',(16.5145707167876,71.1433178571596,15.0999221917026));
#55873=CARTESIAN_POINT('Ctrl Pts',(16.5099178196227,71.204084775008,15.11621253421));
#55874=CARTESIAN_POINT('Ctrl Pts',(16.505269008793,71.2647983252484,15.1324885699756));
#55875=CARTESIAN_POINT('Ctrl Pts',(16.5006201979632,71.3264642846154,15.1454153088827));
#55876=CARTESIAN_POINT('Ctrl Pts',(16.4959713871335,71.3886875454887,15.1548957093241));
#55877=CARTESIAN_POINT('Ctrl Pts',(16.4913250410842,71.4508778158432,15.164371083296));
#55878=CARTESIAN_POINT('Ctrl Pts',(16.486678695035,71.5136243185004,15.1704036737768));
#55879=CARTESIAN_POINT('Ctrl Pts',(16.4820323489858,71.5765224629929,15.1729476564169));
#55880=CARTESIAN_POINT('Ctrl Pts',(16.4803165941806,71.5997488418521,15.1738870721197));
#55881=CARTESIAN_POINT('Ctrl Pts',(16.4786008393754,71.6229958356541,15.1743512890066));
#55882=CARTESIAN_POINT('Ctrl Pts',(16.4768850845702,71.646242925503,15.1743397915547));
#55883=CARTESIAN_POINT('',(15.6831350846103,71.6456222717028,15.1743399855062));
#55884=CARTESIAN_POINT('Ctrl Pts',(16.4768850845224,71.6462429261512,15.1743397915543));
#55885=CARTESIAN_POINT('Ctrl Pts',(16.4718160335965,71.7149244661725,15.1743058232891));
#55886=CARTESIAN_POINT('Ctrl Pts',(16.4667469826707,71.7834665079012,15.1701160948275));
#55887=CARTESIAN_POINT('Ctrl Pts',(16.4616779317449,71.8513919293067,15.1618457851295));
#55888=CARTESIAN_POINT('Ctrl Pts',(16.456590169375,71.9195680845766,15.1535449471452));
#55889=CARTESIAN_POINT('Ctrl Pts',(16.451502407005,71.9871227640871,15.141133486262));
#55890=CARTESIAN_POINT('Ctrl Pts',(16.4464146446351,72.0535901041082,15.1247373430572));
#55891=CARTESIAN_POINT('Ctrl Pts',(16.4413033881495,72.1203643750079,15.1082654862368));
#55892=CARTESIAN_POINT('Ctrl Pts',(16.4361921316639,72.1860409566487,15.0877722091777));
#55893=CARTESIAN_POINT('Ctrl Pts',(16.4310808751783,72.2501685556704,15.0634333464793));
#55894=CARTESIAN_POINT('Ctrl Pts',(16.4298383349499,72.2657578969132,15.0575165985915));
#55895=CARTESIAN_POINT('Ctrl Pts',(16.4285957947215,72.2812558061786,15.0513728042411));
#55896=CARTESIAN_POINT('Ctrl Pts',(16.4273532544931,72.2966560156161,15.0450049008571));
#55897=CARTESIAN_POINT('Ctrl Pts',(16.422749092363,72.3537206155941,15.0214089971274));
#55898=CARTESIAN_POINT('Ctrl Pts',(16.4181449302328,72.4096139955579,14.9946611715146));
#55899=CARTESIAN_POINT('Ctrl Pts',(16.4135407681026,72.4639659032766,14.9648995610384));
#55900=CARTESIAN_POINT('Ctrl Pts',(16.4089285619098,72.5184127707601,14.9350859532057));
#55901=CARTESIAN_POINT('Ctrl Pts',(16.4043163557169,72.5713122838385,14.9022481715234));
#55902=CARTESIAN_POINT('Ctrl Pts',(16.3997041495241,72.6223113381645,14.8665740485079));
#55903=CARTESIAN_POINT('Ctrl Pts',(16.3951122388491,72.6730859766308,14.8310569056382));
#55904=CARTESIAN_POINT('Ctrl Pts',(16.3905203281741,72.7219764138639,14.7927286001777));
#55905=CARTESIAN_POINT('Ctrl Pts',(16.3859284174991,72.7686599742686,14.7518197477828));
#55906=CARTESIAN_POINT('Ctrl Pts',(16.3813392197493,72.8153159537777,14.7109350645553));
#55907=CARTESIAN_POINT('Ctrl Pts',(16.3767500219996,72.8597672615453,14.6674731916271));
#55908=CARTESIAN_POINT('Ctrl Pts',(16.3721608242498,72.9017238749623,14.6217053255063));
#55909=CARTESIAN_POINT('Ctrl Pts',(16.3675726674872,72.9436709711833,14.5759478411042));
#55910=CARTESIAN_POINT('Ctrl Pts',(16.3629845107246,72.9831241541936,14.5278857759225));
#55911=CARTESIAN_POINT('Ctrl Pts',(16.358396353962,73.0198313275112,14.4778260571924));
#55912=CARTESIAN_POINT('Ctrl Pts',(16.3537673094213,73.056865620156,14.427320226707));
#55913=CARTESIAN_POINT('Ctrl Pts',(16.3491382648807,73.0911043789371,14.3747813629434));
#55914=CARTESIAN_POINT('Ctrl Pts',(16.3445092203401,73.1223326069817,14.3205556478174));
#55915=CARTESIAN_POINT('Ctrl Pts',(16.3399153528339,73.1533235254813,14.2667420047362));
#55916=CARTESIAN_POINT('Ctrl Pts',(16.3353214853277,73.1813493306058,14.2112675442954));
#55917=CARTESIAN_POINT('Ctrl Pts',(16.3307276178215,73.2062466996329,14.1544942774377));
#55918=CARTESIAN_POINT('Ctrl Pts',(16.3260809847637,73.2314300419517,14.0970689080232));
#55919=CARTESIAN_POINT('Ctrl Pts',(16.3214343517058,73.2534124201494,14.0383151978398));
#55920=CARTESIAN_POINT('Ctrl Pts',(16.316787718648,73.2720762327638,13.9786248807927));
#55921=CARTESIAN_POINT('Ctrl Pts',(16.3121410855901,73.2907400453782,13.9189345637456));
#55922=CARTESIAN_POINT('Ctrl Pts',(16.3074944525322,73.3060852228388,13.8583081691265));
#55923=CARTESIAN_POINT('Ctrl Pts',(16.3028478194744,73.3180475406727,13.7971468176242));
#55924=CARTESIAN_POINT('Ctrl Pts',(16.2982436572919,73.3299005212503,13.7365444894195));
#55925=CARTESIAN_POINT('Ctrl Pts',(16.2936394951094,73.3384791376836,13.6751773685297));
#55926=CARTESIAN_POINT('Ctrl Pts',(16.2890353329268,73.3436940136494,13.6134303970669));
#55927=CARTESIAN_POINT('Ctrl Pts',(16.2844231267405,73.3489180006065,13.5515755465041));
#55928=CARTESIAN_POINT('Ctrl Pts',(16.2798109205542,73.3507663378284,13.4893400098367));
#55929=CARTESIAN_POINT('Ctrl Pts',(16.2751987143679,73.3492005467128,13.427121886456));
#55930=CARTESIAN_POINT('Ctrl Pts',(16.2706068036402,73.3476416456727,13.365177546443));
#55931=CARTESIAN_POINT('Ctrl Pts',(16.2660148929124,73.342698585339,13.303250976302));
#55932=CARTESIAN_POINT('Ctrl Pts',(16.2614229821846,73.3343853590719,13.2417385436812));
#55933=CARTESIAN_POINT('Ctrl Pts',(16.256833784382,73.326077044303,13.180262452932));
#55934=CARTESIAN_POINT('Ctrl Pts',(16.2522445865795,73.3144025802111,13.1192005160946));
#55935=CARTESIAN_POINT('Ctrl Pts',(16.2476553887769,73.2994278249831,13.0589442984442));
#55936=CARTESIAN_POINT('Ctrl Pts',(16.2430672319615,73.2844564665425,12.9987017489675));
#55937=CARTESIAN_POINT('Ctrl Pts',(16.2384790751462,73.2661864258267,12.9392650477409));
#55938=CARTESIAN_POINT('Ctrl Pts',(16.2338909183309,73.2447342957133,12.8810138828842));
#55939=CARTESIAN_POINT('Ctrl Pts',(16.2292618738412,73.2230909934706,12.8222436087753));
#55940=CARTESIAN_POINT('Ctrl Pts',(16.2246328293516,73.198208753179,12.7646806099599));
#55941=CARTESIAN_POINT('Ctrl Pts',(16.220003784862,73.1702573833474,12.708695332964));
#55942=CARTESIAN_POINT('Ctrl Pts',(16.2154099173039,73.1425184209413,12.6531354980347));
#55943=CARTESIAN_POINT('Ctrl Pts',(16.2108160497458,73.1117571186373,12.5991299068633));
#55944=CARTESIAN_POINT('Ctrl Pts',(16.2062221821877,73.0781850242481,12.547014675149));
#55945=CARTESIAN_POINT('Ctrl Pts',(16.2015755492324,73.0442273190691,12.494300845223));
#55946=CARTESIAN_POINT('Ctrl Pts',(16.196928916277,73.0073941386226,12.4435215181809));
#55947=CARTESIAN_POINT('Ctrl Pts',(16.1922822833217,72.9679470634001,12.394991115994));
#55948=CARTESIAN_POINT('Ctrl Pts',(16.1876356503663,72.9284999881775,12.3464607138071));
#55949=CARTESIAN_POINT('Ctrl Pts',(16.1829890174109,72.8864394209574,12.3001795868457));
#55950=CARTESIAN_POINT('Ctrl Pts',(16.1783423844556,72.8420642520106,12.2564228481221));
#55951=CARTESIAN_POINT('Ctrl Pts',(16.1737382224058,72.7980946786054,12.2130660523975));
#55952=CARTESIAN_POINT('Ctrl Pts',(16.169134060356,72.7516788484522,12.1720162449868));
#55953=CARTESIAN_POINT('Ctrl Pts',(16.1645298983063,72.7030882719126,12.1335605681294));
#55954=CARTESIAN_POINT('Ctrl Pts',(16.1599176921034,72.654412800438,12.0950377035082));
#55955=CARTESIAN_POINT('Ctrl Pts',(16.1553054859005,72.6035553073447,12.0591184354327));
#55956=CARTESIAN_POINT('Ctrl Pts',(16.1506932796976,72.5508263862995,12.0260547466775));
#55957=CARTESIAN_POINT('Ctrl Pts',(16.1461013691019,72.4983294942275,11.9931365517727));
#55958=CARTESIAN_POINT('Ctrl Pts',(16.1415094585062,72.4439780262819,11.963049151286));
#55959=CARTESIAN_POINT('Ctrl Pts',(16.1369175479105,72.3881101177355,11.9359998316124));
#55960=CARTESIAN_POINT('Ctrl Pts',(16.1323283502394,72.3322752162393,11.9089664928171));
#55961=CARTESIAN_POINT('Ctrl Pts',(16.1277391525683,72.2749261065563,11.8849678957112));
#55962=CARTESIAN_POINT('Ctrl Pts',(16.1231499548973,72.2164255705906,11.8641654402362));
#55963=CARTESIAN_POINT('Ctrl Pts',(16.1185617982125,72.1579383045395,11.8433677034669));
#55964=CARTESIAN_POINT('Ctrl Pts',(16.1139736415278,72.0983006085148,11.8257648385037));
#55965=CARTESIAN_POINT('Ctrl Pts',(16.1093854848431,72.0378933893514,11.8114693928313));
#55966=CARTESIAN_POINT('Ctrl Pts',(16.104756440226,71.9769478436947,11.7970465515058));
#55967=CARTESIAN_POINT('Ctrl Pts',(16.1001273956088,71.9152194931725,11.7859905263778));
#55968=CARTESIAN_POINT('Ctrl Pts',(16.0954983509916,71.8531109370326,11.7783644002809));
#55969=CARTESIAN_POINT('Ctrl Pts',(16.0909044835606,71.7914743582494,11.770796226889));
#55970=CARTESIAN_POINT('Ctrl Pts',(16.0863106161296,71.729463849279,11.7666059799524));
#55971=CARTESIAN_POINT('Ctrl Pts',(16.0817167486986,71.667476448231,11.7658029849711));
#55972=CARTESIAN_POINT('Ctrl Pts',(16.0770701154883,71.6047770515562,11.7649907666814));
#55973=CARTESIAN_POINT('Ctrl Pts',(16.072423482278,71.5421018294417,11.7676441042901));
#55974=CARTESIAN_POINT('Ctrl Pts',(16.0677768490677,71.4798573743076,11.7737186333987));
#55975=CARTESIAN_POINT('Ctrl Pts',(16.0631302158574,71.4176129191735,11.7797931625072));
#55976=CARTESIAN_POINT('Ctrl Pts',(16.0584835826472,71.355799745575,11.7892887409084));
#55977=CARTESIAN_POINT('Ctrl Pts',(16.0538369494369,71.2948122883247,11.8021081893533));
#55978=CARTESIAN_POINT('Ctrl Pts',(16.0492327873053,71.2343822676048,11.8148104656913));
#55979=CARTESIAN_POINT('Ctrl Pts',(16.0446286251737,71.1745240167357,11.8308262668942));
#55980=CARTESIAN_POINT('Ctrl Pts',(16.0400244630421,71.115626873338,11.8500878820545));
#55981=CARTESIAN_POINT('Ctrl Pts',(16.0354122568494,71.0566268290858,11.8693831497239));
#55982=CARTESIAN_POINT('Ctrl Pts',(16.0308000506567,70.9985917641664,11.8919355246881));
#55983=CARTESIAN_POINT('Ctrl Pts',(16.0261878444641,70.9419032972114,11.9176252949866));
#55984=CARTESIAN_POINT('Ctrl Pts',(16.0215959337898,70.8854642817718,11.9432020202077));
#55985=CARTESIAN_POINT('Ctrl Pts',(16.0170040231156,70.830360513052,11.9718884022468));
#55986=CARTESIAN_POINT('Ctrl Pts',(16.0124121124413,70.776951565364,12.0035170809115));
#55987=CARTESIAN_POINT('Ctrl Pts',(16.0078229146931,70.7235741719756,12.0351270731792));
#55988=CARTESIAN_POINT('Ctrl Pts',(16.0032337169449,70.6718900493519,12.0696756566565));
#55989=CARTESIAN_POINT('Ctrl Pts',(15.9986445191967,70.6222341362716,12.1069495787386));
#55990=CARTESIAN_POINT('Ctrl Pts',(15.9940563624364,70.5725894868608,12.1442150458127));
#55991=CARTESIAN_POINT('Ctrl Pts',(15.9894682056761,70.5249725388424,12.1842043195397));
#55992=CARTESIAN_POINT('Ctrl Pts',(15.9848800489158,70.4796875205036,12.2266620528809));
#55993=CARTESIAN_POINT('Ctrl Pts',(15.9802510043744,70.4339989405564,12.26949815222));
#55994=CARTESIAN_POINT('Ctrl Pts',(15.9756219598329,70.390684465659,12.3148465929179));
#55995=CARTESIAN_POINT('Ctrl Pts',(15.9709929152914,70.3500190739218,12.3624066215651));
#55996=CARTESIAN_POINT('Ctrl Pts',(15.9663990477895,70.3096627066671,12.4096052319987));
#55997=CARTESIAN_POINT('Ctrl Pts',(15.9618051802875,70.2719155657789,12.4589814900987));
#55998=CARTESIAN_POINT('Ctrl Pts',(15.9572113127856,70.2370047462432,12.51020958288));
#55999=CARTESIAN_POINT('Ctrl Pts',(15.9525646797243,70.2016929380158,12.5620260859644));
#56000=CARTESIAN_POINT('Ctrl Pts',(15.9479180466631,70.1692833129285,12.6157367890329));
#56001=CARTESIAN_POINT('Ctrl Pts',(15.9432714136018,70.1399634886832,12.6709782568701));
#56002=CARTESIAN_POINT('Ctrl Pts',(15.9386247805406,70.1106436644379,12.7262197247073));
#56003=CARTESIAN_POINT('Ctrl Pts',(15.9339781474793,70.0844138067301,12.7829914498343));
#56004=CARTESIAN_POINT('Ctrl Pts',(15.9293315144181,70.061410791909,12.8409109568184));
#56005=CARTESIAN_POINT('Ctrl Pts',(15.924727351917,70.0386180262967,12.8983010753455));
#56006=CARTESIAN_POINT('Ctrl Pts',(15.9201231894159,70.0189032023114,12.9570449467636));
#56007=CARTESIAN_POINT('Ctrl Pts',(15.9155190269148,70.0024249449438,13.0167806225864));
#56008=CARTESIAN_POINT('Ctrl Pts',(15.9109068207683,69.9859178994396,13.0766206588861));
#56009=CARTESIAN_POINT('Ctrl Pts',(15.9062946146218,69.9726589726973,13.1374555102616));
#56010=CARTESIAN_POINT('Ctrl Pts',(15.9016824084754,69.9627591785472,13.1989009376986));
#56011=CARTESIAN_POINT('Ctrl Pts',(15.8970904974269,69.9529029464771,13.2600759867233));
#56012=CARTESIAN_POINT('Ctrl Pts',(15.8924985863785,69.9463764548892,13.321855751545));
#56013=CARTESIAN_POINT('Ctrl Pts',(15.8879066753301,69.9432388217305,13.3838480482384));
#56014=CARTESIAN_POINT('Ctrl Pts',(15.883317477207,69.9401030423022,13.4458037195546));
#56015=CARTESIAN_POINT('Ctrl Pts',(15.878728279084,69.9403521761729,13.5079711681707));
#56016=CARTESIAN_POINT('Ctrl Pts',(15.8741390809609,69.9439934776256,13.5699533952491));
#56017=CARTESIAN_POINT('Ctrl Pts',(15.8695509238258,69.9476339531059,13.6319215626273));
#56018=CARTESIAN_POINT('Ctrl Pts',(15.8649627666906,69.9546650384593,13.6937040858136));
#56019=CARTESIAN_POINT('Ctrl Pts',(15.8603746095555,69.9650419344671,13.75490631302));
#56020=CARTESIAN_POINT('Ctrl Pts',(15.8557455653758,69.9755113034651,13.8166539396354));
#56021=CARTESIAN_POINT('Ctrl Pts',(15.8511165211961,69.9893863585377,13.8778103537777));
#56022=CARTESIAN_POINT('Ctrl Pts',(15.8464874770164,70.00656829291,13.9379802041074));
#56023=CARTESIAN_POINT('Ctrl Pts',(15.8418936091439,70.0236196610188,13.9976928211387));
#56024=CARTESIAN_POINT('Ctrl Pts',(15.8372997412715,70.0439276007735,14.0564333496011));
#56025=CARTESIAN_POINT('Ctrl Pts',(15.832705873399,70.0673459657709,14.1138325097829));
#56026=CARTESIAN_POINT('Ctrl Pts',(15.8280592410657,70.0910333105118,14.1718909479024));
#56027=CARTESIAN_POINT('Ctrl Pts',(15.8234126087324,70.1179027756458,14.2285765194346));
#56028=CARTESIAN_POINT('Ctrl Pts',(15.8187659763991,70.147755046646,14.2835320702303));
#56029=CARTESIAN_POINT('Ctrl Pts',(15.8141193440658,70.1776073176461,14.3384876210261));
#56030=CARTESIAN_POINT('Ctrl Pts',(15.8094727117326,70.2104420630163,14.3917127326367));
#56031=CARTESIAN_POINT('Ctrl Pts',(15.8048260793993,70.2460160674514,14.4428820303227));
#56032=CARTESIAN_POINT('Ctrl Pts',(15.8002390201906,70.2811339878999,14.4933953012933));
#56033=CARTESIAN_POINT('Ctrl Pts',(15.7956519609819,70.3190625536555,14.5421082849052));
#56034=CARTESIAN_POINT('Ctrl Pts',(15.7910649017732,70.359590125684,14.5886902174917));
#56035=CARTESIAN_POINT('Ctrl Pts',(15.7864856588548,70.4000486392479,14.6351927750605));
#56036=CARTESIAN_POINT('Ctrl Pts',(15.7819064159364,70.4430970338756,14.6795711079166));
#56037=CARTESIAN_POINT('Ctrl Pts',(15.777327173018,70.4884814205779,14.7215247645125));
#56038=CARTESIAN_POINT('Ctrl Pts',(15.77275228342,70.5338226619869,14.7634385372859));
#56039=CARTESIAN_POINT('Ctrl Pts',(15.7681773938221,70.5814951205441,14.8029318564857));
#56040=CARTESIAN_POINT('Ctrl Pts',(15.7636025042241,70.6312069215191,14.8397398421458));
#56041=CARTESIAN_POINT('Ctrl Pts',(15.7590302639737,70.6808899340752,14.8765265120681));
#56042=CARTESIAN_POINT('Ctrl Pts',(15.7544580237233,70.7326095370287,14.9106306281275));
#56043=CARTESIAN_POINT('Ctrl Pts',(15.7498857834729,70.7860411279776,14.9418278311937));
#56044=CARTESIAN_POINT('Ctrl Pts',(15.7453144922606,70.8394616283865,14.9730185588055));
#56045=CARTESIAN_POINT('Ctrl Pts',(15.7407432010483,70.8945929695165,15.001303313918));
#56046=CARTESIAN_POINT('Ctrl Pts',(15.736171909836,70.9510837312444,15.0265024107085));
#56047=CARTESIAN_POINT('Ctrl Pts',(15.7315966771968,71.007623200043,15.0517232344885));
#56048=CARTESIAN_POINT('Ctrl Pts',(15.7270214445576,71.0655239636073,15.0738528742927));
#56049=CARTESIAN_POINT('Ctrl Pts',(15.7224462119185,71.1244134392268,15.092759328765));
#56050=CARTESIAN_POINT('Ctrl Pts',(15.717869102674,71.1833270693129,15.1116735380239));
#56051=CARTESIAN_POINT('Ctrl Pts',(15.7132919934295,71.2432297242223,15.1273617962317));
#56052=CARTESIAN_POINT('Ctrl Pts',(15.708714884185,71.3037353937151,15.1397425347676));
#56053=CARTESIAN_POINT('Ctrl Pts',(15.7041294199245,71.364351509739,15.1521458729977));
#56054=CARTESIAN_POINT('Ctrl Pts',(15.699543955664,71.4255723322453,15.161229552918));
#56055=CARTESIAN_POINT('Ctrl Pts',(15.6949584914034,71.4870043162473,15.1669636539916));
#56056=CARTESIAN_POINT('Ctrl Pts',(15.6910173558057,71.5398041561834,15.1718920251615));
#56057=CARTESIAN_POINT('Ctrl Pts',(15.687076220208,71.5927597118406,15.1743468795833));
#56058=CARTESIAN_POINT('Ctrl Pts',(15.6831350846103,71.6456222717028,15.1743399855062));
#56059=CARTESIAN_POINT('',(14.8893850846217,71.6442647494568,15.1743396219082));
#56060=CARTESIAN_POINT('Ctrl Pts',(15.6831350845702,71.6456222722405,15.1743399855061));
#56061=CARTESIAN_POINT('Ctrl Pts',(15.6821969378403,71.658205660058,15.1743383444381));
#56062=CARTESIAN_POINT('Ctrl Pts',(15.6812587911104,71.6707879882523,15.1741973479661));
#56063=CARTESIAN_POINT('Ctrl Pts',(15.6803206443805,71.683367201171,15.1739170540948));
#56064=CARTESIAN_POINT('Ctrl Pts',(15.6757164819436,71.7451024689719,15.1725414499677));
#56065=CARTESIAN_POINT('Ctrl Pts',(15.6711123195067,71.8068849098217,15.167803682167));
#56066=CARTESIAN_POINT('Ctrl Pts',(15.6665081570698,71.8683193739522,15.1596987270862));
#56067=CARTESIAN_POINT('Ctrl Pts',(15.6618959509153,71.9298611673719,15.1515796122161));
#56068=CARTESIAN_POINT('Ctrl Pts',(15.6572837447608,71.9910532545598,15.1400814978904));
#56069=CARTESIAN_POINT('Ctrl Pts',(15.6526715386063,72.0514985127723,15.125251894282));
#56070=CARTESIAN_POINT('Ctrl Pts',(15.6480796276455,72.1116777923658,15.1104875457094));
#56071=CARTESIAN_POINT('Ctrl Pts',(15.6434877166847,72.1711163008623,15.0924210600151));
#56072=CARTESIAN_POINT('Ctrl Pts',(15.6388958057239,72.2294298237826,15.0711508362838));
#56073=CARTESIAN_POINT('Ctrl Pts',(15.6343066076969,72.2877088946567,15.0498931791528));
#56074=CARTESIAN_POINT('Ctrl Pts',(15.6297174096699,72.3448638225535,15.0254357112682));
#56075=CARTESIAN_POINT('Ctrl Pts',(15.6251282116429,72.4005261711974,14.9979264711277));
#56076=CARTESIAN_POINT('Ctrl Pts',(15.6205400546121,72.4561758936071,14.970423471078));
#56077=CARTESIAN_POINT('Ctrl Pts',(15.6159518975812,72.5103332546068,14.9398702980457));
#56078=CARTESIAN_POINT('Ctrl Pts',(15.6113637405504,72.5626522657928,14.9064620135938));
#56079=CARTESIAN_POINT('Ctrl Pts',(15.6067346962846,72.6154375164042,14.8727560121364));
#56080=CARTESIAN_POINT('Ctrl Pts',(15.6021056520189,72.6663510289185,14.8361440122005));
#56081=CARTESIAN_POINT('Ctrl Pts',(15.5974766077532,72.7150672185874,14.796871085328));
#56082=CARTESIAN_POINT('Ctrl Pts',(15.5928827400036,72.7634132096295,14.7578965968945));
#56083=CARTESIAN_POINT('Ctrl Pts',(15.588288872254,72.809594814753,14.7163018703938));
#56084=CARTESIAN_POINT('Ctrl Pts',(15.5836950045044,72.8533289087601,14.6723654132508));
#56085=CARTESIAN_POINT('Ctrl Pts',(15.5790483719806,72.8975653288505,14.6279243056986));
#56086=CARTESIAN_POINT('Ctrl Pts',(15.5744017394569,72.9392972884855,14.5810877163756));
#56087=CARTESIAN_POINT('Ctrl Pts',(15.5697551069331,72.9782735500341,14.5321783914294));
#56088=CARTESIAN_POINT('Ctrl Pts',(15.5651084744093,73.0172498115826,14.4832690664832));
#56089=CARTESIAN_POINT('Ctrl Pts',(15.5604618418855,73.053470118873,14.4322874742781));
#56090=CARTESIAN_POINT('Ctrl Pts',(15.5558152093618,73.0867296100807,14.3795844054868));
#56091=CARTESIAN_POINT('Ctrl Pts',(15.5512110445284,73.1196851276543,14.3273630140382));
#56092=CARTESIAN_POINT('Ctrl Pts',(15.546606879695,73.1498640561934,14.2732450603545));
#56093=CARTESIAN_POINT('Ctrl Pts',(15.5420027148615,73.1770439298689,14.2175571601528));
#56094=CARTESIAN_POINT('Ctrl Pts',(15.5373905090066,73.2042712722944,14.1617720028761));
#56095=CARTESIAN_POINT('Ctrl Pts',(15.5327783031517,73.228488761569,14.1044118176455));
#56096=CARTESIAN_POINT('Ctrl Pts',(15.5281660972967,73.2495166336152,14.045833883476));
#56097=CARTESIAN_POINT('Ctrl Pts',(15.5235741838923,73.2704519887471,13.9875136762749));
#56098=CARTESIAN_POINT('Ctrl Pts',(15.518982270488,73.2882255366742,13.9279868828877));
#56099=CARTESIAN_POINT('Ctrl Pts',(15.5143903570836,73.3027070635906,13.8676281335276));
#56100=CARTESIAN_POINT('Ctrl Pts',(15.5098011566025,73.3171800347551,13.807305044391));
#56101=CARTESIAN_POINT('Ctrl Pts',(15.5052119561214,73.3283647240605,13.7461514663075));
#56102=CARTESIAN_POINT('Ctrl Pts',(15.5006227556404,73.336181012075,13.6845562975226));
#56103=CARTESIAN_POINT('Ctrl Pts',(15.4960345961492,73.3439955270841,13.6229751006593));
#56104=CARTESIAN_POINT('Ctrl Pts',(15.4914464366581,73.3484430942568,13.5609530149312));
#56105=CARTESIAN_POINT('Ctrl Pts',(15.486858277167,73.34949519187,13.4988862016455));
#56106=CARTESIAN_POINT('Ctrl Pts',(15.482229235265,73.3505566641109,13.4362663472186));
#56107=CARTESIAN_POINT('Ctrl Pts',(15.477600193363,73.3481618118956,13.3736014875569));
#56108=CARTESIAN_POINT('Ctrl Pts',(15.472971151461,73.3423350717331,13.3112983997492));
#56109=CARTESIAN_POINT('Ctrl Pts',(15.4683772812649,73.3365526034514,13.2494686941073));
#56110=CARTESIAN_POINT('Ctrl Pts',(15.4637834110687,73.3273903518195,13.1879957816731));
#56111=CARTESIAN_POINT('Ctrl Pts',(15.4591895408726,73.3149240793806,13.127269517013));
#56112=CARTESIAN_POINT('Ctrl Pts',(15.4545429131177,73.3023146400532,13.0658458513937));
#56113=CARTESIAN_POINT('Ctrl Pts',(15.4498962853628,73.2863249258895,13.0051866114072));
#56114=CARTESIAN_POINT('Ctrl Pts',(15.4452496576078,73.2670851899437,12.9456795061059));
#56115=CARTESIAN_POINT('Ctrl Pts',(15.4406030298529,73.2478454539978,12.8861724008046));
#56116=CARTESIAN_POINT('Ctrl Pts',(15.4359564020979,73.2253559451803,12.8278179024466));
#56117=CARTESIAN_POINT('Ctrl Pts',(15.431309774343,73.1997959114136,12.7709805537892));
#56118=CARTESIAN_POINT('Ctrl Pts',(15.426705619554,73.1744695116935,12.7146627326055));
#56119=CARTESIAN_POINT('Ctrl Pts',(15.4221014647651,73.1460284107687,12.6596117718381));
#56120=CARTESIAN_POINT('Ctrl Pts',(15.4174973099762,73.1146219799088,12.6061935347818));
#56121=CARTESIAN_POINT('Ctrl Pts',(15.4128851028657,73.0831606215557,12.5526818732333));
#56122=CARTESIAN_POINT('Ctrl Pts',(15.4082728957552,73.0487237179752,12.5008091377367));
#56123=CARTESIAN_POINT('Ctrl Pts',(15.4036606886447,73.0115097905952,12.4509225369778));
#56124=CARTESIAN_POINT('Ctrl Pts',(15.3990687852806,72.9744596854649,12.4012555458042));
#56125=CARTESIAN_POINT('Ctrl Pts',(15.3944768819165,72.9346572372938,12.353557663944));
#56126=CARTESIAN_POINT('Ctrl Pts',(15.3898849785524,72.8923428010913,12.3081443779856));
#56127=CARTESIAN_POINT('Ctrl Pts',(15.3852957880814,72.8500533642259,12.2627579221624));
#56128=CARTESIAN_POINT('Ctrl Pts',(15.3807065976103,72.8052552276664,12.2196537557614));
#56129=CARTESIAN_POINT('Ctrl Pts',(15.3761174071393,72.758228311868,12.1791134891459));
#56130=CARTESIAN_POINT('Ctrl Pts',(15.3715292576111,72.7112120629463,12.1385824180735));
#56131=CARTESIAN_POINT('Ctrl Pts',(15.3669411080828,72.6619684226592,12.1006144229581));
#56132=CARTESIAN_POINT('Ctrl Pts',(15.3623529585546,72.6108118680941,12.0654521152545));
#56133=CARTESIAN_POINT('Ctrl Pts',(15.357723906952,72.5591992671029,12.0299763453778));
#56134=CARTESIAN_POINT('Ctrl Pts',(15.3530948553495,72.5056398879805,11.9973568613451));
#56135=CARTESIAN_POINT('Ctrl Pts',(15.348465803747,72.4504863152568,11.9677979960783));
#56136=CARTESIAN_POINT('Ctrl Pts',(15.3438719432836,72.3957520329663,11.9384638442582));
#56137=CARTESIAN_POINT('Ctrl Pts',(15.3392780828202,72.3394482025744,11.9121441018625));
#56138=CARTESIAN_POINT('Ctrl Pts',(15.3346842223568,72.2819416499901,11.8889909666837));
#56139=CARTESIAN_POINT('Ctrl Pts',(15.3300375751847,72.2237743064078,11.8655717855916));
#56140=CARTESIAN_POINT('Ctrl Pts',(15.3253909280126,72.1643769223286,11.8453926367438));
#56141=CARTESIAN_POINT('Ctrl Pts',(15.3207442808405,72.1041446427351,11.8285591121329));
#56142=CARTESIAN_POINT('Ctrl Pts',(15.3160976336684,72.0439123631416,11.811725587522));
#56143=CARTESIAN_POINT('Ctrl Pts',(15.3114509864963,71.9828457192163,11.798237740532));
#56144=CARTESIAN_POINT('Ctrl Pts',(15.3068043393242,71.9213476093244,11.7881475235598));
#56145=CARTESIAN_POINT('Ctrl Pts',(15.3022001718672,71.8604117160359,11.7781495514959));
#56146=CARTESIAN_POINT('Ctrl Pts',(15.2975960044103,71.79881131457,11.7714477650766));
#56147=CARTESIAN_POINT('Ctrl Pts',(15.2929918369534,71.7369338960352,11.7681197511351));
#56148=CARTESIAN_POINT('Ctrl Pts',(15.2883796314264,71.6749484503643,11.764785927064));
#56149=CARTESIAN_POINT('Ctrl Pts',(15.2837674258994,71.6126855166509,11.7648377959761));
#56150=CARTESIAN_POINT('Ctrl Pts',(15.2791552203724,71.550544182294,11.7683016690825));
#56151=CARTESIAN_POINT('Ctrl Pts',(15.274563304546,71.4886762158662,11.7717503041541));
#56152=CARTESIAN_POINT('Ctrl Pts',(15.2699713887197,71.4269292909023,11.7785809859631));
#56153=CARTESIAN_POINT('Ctrl Pts',(15.2653794728934,71.3656991640179,11.7887676311851));
#56154=CARTESIAN_POINT('Ctrl Pts',(15.2607902700722,71.3045052132431,11.7989482579124));
#56155=CARTESIAN_POINT('Ctrl Pts',(15.2562010672511,71.2438279543311,11.8124808326942));
#56156=CARTESIAN_POINT('Ctrl Pts',(15.2516118644299,71.1840567609523,11.8292875780976));
#56157=CARTESIAN_POINT('Ctrl Pts',(15.2470237026838,71.1242991268559,11.8460905108381));
#56158=CARTESIAN_POINT('Ctrl Pts',(15.2424355409376,71.0654476381596,11.8661660020247));
#56159=CARTESIAN_POINT('Ctrl Pts',(15.2378473791915,71.0078782486064,11.8893859256289));
#56160=CARTESIAN_POINT('Ctrl Pts',(15.2332183396177,70.9497959495882,11.9128127251212));
#56161=CARTESIAN_POINT('Ctrl Pts',(15.2285893000438,70.8930192079004,11.9394401021789));
#56162=CARTESIAN_POINT('Ctrl Pts',(15.22396026047,70.8379131137208,11.9690870231465));
#56163=CARTESIAN_POINT('Ctrl Pts',(15.2193663882507,70.7832256669776,11.9985087129915));
#56164=CARTESIAN_POINT('Ctrl Pts',(15.2147725160314,70.7301839795792,12.0309039078793));
#56165=CARTESIAN_POINT('Ctrl Pts',(15.210178643812,70.6791175554324,12.0660509008798));
#56166=CARTESIAN_POINT('Ctrl Pts',(15.205532020561,70.6274647400162,12.1016014837182));
#56167=CARTESIAN_POINT('Ctrl Pts',(15.2008853973099,70.5778332722583,12.1399671531862));
#56168=CARTESIAN_POINT('Ctrl Pts',(15.1962387740588,70.5305294428678,12.1808768575346));
#56169=CARTESIAN_POINT('Ctrl Pts',(15.1915921508077,70.4832256134773,12.2217865618831));
#56170=CARTESIAN_POINT('Ctrl Pts',(15.1869455275566,70.4382497603648,12.2652398878373));
#56171=CARTESIAN_POINT('Ctrl Pts',(15.1822989043055,70.3958677455696,12.3109296912015));
#56172=CARTESIAN_POINT('Ctrl Pts',(15.1776947235287,70.3538728500822,12.3562021617623));
#56173=CARTESIAN_POINT('Ctrl Pts',(15.173090542752,70.3142585503185,12.4038493581946));
#56174=CARTESIAN_POINT('Ctrl Pts',(15.1684863619753,70.2773035691007,12.4535911298298));
#56175=CARTESIAN_POINT('Ctrl Pts',(15.1638741581133,70.2402841914179,12.5034195797463));
#56176=CARTESIAN_POINT('Ctrl Pts',(15.1592619542512,70.2059337915272,12.5553495686052));
#56177=CARTESIAN_POINT('Ctrl Pts',(15.1546497503892,70.1744947529164,12.6090629583402));
#56178=CARTESIAN_POINT('Ctrl Pts',(15.1500578207962,70.1431939136448,12.6625402354172));
#56179=CARTESIAN_POINT('Ctrl Pts',(15.1454658912032,70.1147791748378,12.7177848420542));
#56180=CARTESIAN_POINT('Ctrl Pts',(15.1408739616102,70.0894474072078,12.77445247137));
#56181=CARTESIAN_POINT('Ctrl Pts',(15.1362847448956,70.064130605401,12.8310866218645));
#56182=CARTESIAN_POINT('Ctrl Pts',(15.131695528181,70.0418933691153,12.8891416656004));
#56183=CARTESIAN_POINT('Ctrl Pts',(15.1271063114665,70.022885951727,12.948250061086));
#56184=CARTESIAN_POINT('Ctrl Pts',(15.1225181357252,70.0038828457964,13.0073450489981));
#56185=CARTESIAN_POINT('Ctrl Pts',(15.1179299599839,69.988108259134,13.0674924315786));
#56186=CARTESIAN_POINT('Ctrl Pts',(15.1133417842426,69.9756630622344,13.1283080418545));
#56187=CARTESIAN_POINT('Ctrl Pts',(15.1087127579963,69.9631070603859,13.1896651197058));
#56188=CARTESIAN_POINT('Ctrl Pts',(15.1040837317499,69.9539401682231,13.2517018770536));
#56189=CARTESIAN_POINT('Ctrl Pts',(15.0994547055036,69.9482131515873,13.3140139840398));
#56190=CARTESIAN_POINT('Ctrl Pts',(15.094860819207,69.9425296099863,13.3758530662059));
#56191=CARTESIAN_POINT('Ctrl Pts',(15.0902669329104,69.9402338592575,13.4379628160748));
#56192=CARTESIAN_POINT('Ctrl Pts',(15.0856730466139,69.9413231041099,13.4999460931263));
#56193=CARTESIAN_POINT('Ctrl Pts',(15.0810264503927,69.9424248468802,13.5626405618899));
#56194=CARTESIAN_POINT('Ctrl Pts',(15.0763798541715,69.9469897370778,13.6252051050966));
#56195=CARTESIAN_POINT('Ctrl Pts',(15.0717332579503,69.9549610253152,13.6872346852293));
#56196=CARTESIAN_POINT('Ctrl Pts',(15.0670866617291,69.9629323135527,13.749264265362));
#56197=CARTESIAN_POINT('Ctrl Pts',(15.0624400655079,69.9743098420003,13.8107583724795));
#56198=CARTESIAN_POINT('Ctrl Pts',(15.0577934692867,69.9889844444823,13.8713257318424));
#56199=CARTESIAN_POINT('Ctrl Pts',(15.0531893714168,70.0035248312108,13.9313391345461));
#56200=CARTESIAN_POINT('Ctrl Pts',(15.048585273547,70.0213596651757,13.9906799489558));
#56201=CARTESIAN_POINT('Ctrl Pts',(15.0439811756772,70.0424093923433,14.0489610931354));
#56202=CARTESIAN_POINT('Ctrl Pts',(15.0393689614518,70.0634962271214,14.1073449785038));
#56203=CARTESIAN_POINT('Ctrl Pts',(15.0347567472264,70.087809226176,14.16466494563));
#56204=CARTESIAN_POINT('Ctrl Pts',(15.030144533001,70.1152170875011,14.2205431965559));
#56205=CARTESIAN_POINT('Ctrl Pts',(15.0255526864647,70.1425039148126,14.2761746872949));
#56206=CARTESIAN_POINT('Ctrl Pts',(15.0209608399285,70.1728581284923,14.3303766992204));
#56207=CARTESIAN_POINT('Ctrl Pts',(15.0163689933922,70.2061014787994,14.3827949399891));
#56208=CARTESIAN_POINT('Ctrl Pts',(15.0117798595527,70.2393251901385,14.4351822139586));
#56209=CARTESIAN_POINT('Ctrl Pts',(15.0071907257131,70.2754343820395,14.4857873791719));
#56210=CARTESIAN_POINT('Ctrl Pts',(15.0026015918736,70.3142056854256,14.5342821676815));
#56211=CARTESIAN_POINT('Ctrl Pts',(14.9980134986852,70.3529681968686,14.5827659593098));
#56212=CARTESIAN_POINT('Ctrl Pts',(14.9934254054969,70.3943913044572,14.6291399285655));
#56213=CARTESIAN_POINT('Ctrl Pts',(14.9888373123086,70.4382105014878,14.6731077883058));
#56214=CARTESIAN_POINT('Ctrl Pts',(14.9842082058052,70.4824214016638,14.7174686800986));
#56215=CARTESIAN_POINT('Ctrl Pts',(14.9795790993018,70.5290710975088,14.7593798349948));
#56216=CARTESIAN_POINT('Ctrl Pts',(14.9749499927984,70.5778505644227,14.7985755673648));
#56217=CARTESIAN_POINT('Ctrl Pts',(14.970356187313,70.6262580448987,14.8374723977215));
#56218=CARTESIAN_POINT('Ctrl Pts',(14.9657623818276,70.6767624744858,14.8736948247573));
#56219=CARTESIAN_POINT('Ctrl Pts',(14.9611685763422,70.7290312669044,14.9070258106954));
#56220=CARTESIAN_POINT('Ctrl Pts',(14.9565218193298,70.7819025472562,14.9407409937022));
#56221=CARTESIAN_POINT('Ctrl Pts',(14.9518750623174,70.836578670003,14.9714973752288));
#56222=CARTESIAN_POINT('Ctrl Pts',(14.9472283053051,70.8926906051386,14.9991185050504));
#56223=CARTESIAN_POINT('Ctrl Pts',(14.9425815482927,70.9488025402743,15.0267396348719));
#56224=CARTESIAN_POINT('Ctrl Pts',(14.9379347912803,71.0063497753763,15.0512253628403));
#56225=CARTESIAN_POINT('Ctrl Pts',(14.9332880342679,71.0649457963341,15.0724505462093));
#56226=CARTESIAN_POINT('Ctrl Pts',(14.9279993725813,71.1316362925666,15.0966077839939));
#56227=CARTESIAN_POINT('Ctrl Pts',(14.9227107108947,71.1999016312767,15.1166213767754));
#56228=CARTESIAN_POINT('Ctrl Pts',(14.917422049208,71.2692533052774,15.1323142000384));
#56229=CARTESIAN_POINT('Ctrl Pts',(14.9121766025752,71.3380382884026,15.1478787930909));
#56230=CARTESIAN_POINT('Ctrl Pts',(14.9069311559423,71.4078917346752,15.1591928399152));
#56231=CARTESIAN_POINT('Ctrl Pts',(14.9016857093095,71.478316607017,15.1661302943434));
#56232=CARTESIAN_POINT('Ctrl Pts',(14.8975855010802,71.5333656164401,15.171553094293));
#56233=CARTESIAN_POINT('Ctrl Pts',(14.893485292851,71.5887633394563,15.1743026527472));
#56234=CARTESIAN_POINT('Ctrl Pts',(14.8893850846217,71.6442647494568,15.1743396219082));
#56235=CARTESIAN_POINT('',(14.0956350845187,71.6466915584598,15.1743395106248));
#56236=CARTESIAN_POINT('Ctrl Pts',(14.8893850845702,71.6442647501543,15.1743396219087));
#56237=CARTESIAN_POINT('Ctrl Pts',(14.8847838848648,71.706547701914,15.174381108189));
#56238=CARTESIAN_POINT('Ctrl Pts',(14.8801826851594,71.7688576998196,15.1710041874919));
#56239=CARTESIAN_POINT('Ctrl Pts',(14.875581485454,71.8307953836467,15.1642264864305));
#56240=CARTESIAN_POINT('Ctrl Pts',(14.8709803942258,71.8927316072403,15.1574489451591));
#56241=CARTESIAN_POINT('Ctrl Pts',(14.8663793029975,71.9542950347125,15.1472708391474));
#56242=CARTESIAN_POINT('Ctrl Pts',(14.8617782117693,72.0150920328097,15.1337615924396));
#56243=CARTESIAN_POINT('Ctrl Pts',(14.8571720998765,72.0759553719816,15.1202376045772));
#56244=CARTESIAN_POINT('Ctrl Pts',(14.8525659879837,72.1360501195801,15.1033753258721));
#56245=CARTESIAN_POINT('Ctrl Pts',(14.8479598760909,72.194994496164,15.0832949901944));
#56246=CARTESIAN_POINT('Ctrl Pts',(14.8433512710408,72.2539707776611,15.0632037856025));
#56247=CARTESIAN_POINT('Ctrl Pts',(14.8387426659907,72.3117949807797,15.0398912423987));
#56248=CARTESIAN_POINT('Ctrl Pts',(14.8341340609407,72.3681050013233,15.0135259365046));
#56249=CARTESIAN_POINT('Ctrl Pts',(14.8295163898702,72.4245257946042,14.9871087649376));
#56250=CARTESIAN_POINT('Ctrl Pts',(14.8248987187997,72.4794260101098,14.9576270709721));
#56251=CARTESIAN_POINT('Ctrl Pts',(14.8202810477292,72.5324685061645,14.9252952624712));
#56252=CARTESIAN_POINT('Ctrl Pts',(14.8164482315691,72.5764954914006,14.8984588169529));
#56253=CARTESIAN_POINT('Ctrl Pts',(14.8126154154091,72.6192429818788,14.8696596754254));
#56254=CARTESIAN_POINT('Ctrl Pts',(14.8087825992491,72.6605353656926,14.839041644699));
#56255=CARTESIAN_POINT('Ctrl Pts',(14.8041783207442,72.7101390062721,14.8022608718026));
#56256=CARTESIAN_POINT('Ctrl Pts',(14.7995740422393,72.7578391002769,14.762708075234));
#56257=CARTESIAN_POINT('Ctrl Pts',(14.7949697637345,72.803310164833,14.7206074067334));
#56258=CARTESIAN_POINT('Ctrl Pts',(14.7903575720885,72.8488593782131,14.6784343819384));
#56259=CARTESIAN_POINT('Ctrl Pts',(14.7857453804425,72.8921714543769,14.6337049862599));
#56260=CARTESIAN_POINT('Ctrl Pts',(14.7811331887965,72.9329496690055,14.5866873713998));
#56261=CARTESIAN_POINT('Ctrl Pts',(14.7765411590811,72.9735496240125,14.5398752913408));
#56262=CARTESIAN_POINT('Ctrl Pts',(14.7719491293658,73.011637470106,14.4907953222569));
#56263=CARTESIAN_POINT('Ctrl Pts',(14.7673570996505,73.0469563879207,14.4397497239385));
#56264=CARTESIAN_POINT('Ctrl Pts',(14.7627677822103,73.0822544446723,14.388734275622));
#56265=CARTESIAN_POINT('Ctrl Pts',(14.7581784647701,73.114786528635,14.3357559168311));
#56266=CARTESIAN_POINT('Ctrl Pts',(14.7535891473299,73.1443373721587,14.2811483156279));
#56267=CARTESIAN_POINT('Ctrl Pts',(14.7490008704379,73.1738815155408,14.2265530957517));
#56268=CARTESIAN_POINT('Ctrl Pts',(14.7444125935458,73.2004455195007,14.1703298128512));
#56269=CARTESIAN_POINT('Ctrl Pts',(14.7398243166538,73.2238596012906,14.1128375554472));
#56270=CARTESIAN_POINT('Ctrl Pts',(14.7351953872852,73.2474811335972,14.0548359123408));
#56271=CARTESIAN_POINT('Ctrl Pts',(14.7305664579166,73.2678964206968,13.9955431691668));
#56272=CARTESIAN_POINT('Ctrl Pts',(14.725937528548,73.2849812384895,13.935347394957));
#56273=CARTESIAN_POINT('Ctrl Pts',(14.7213435412563,73.3019370893071,13.8756060163989));
#56274=CARTESIAN_POINT('Ctrl Pts',(14.7167495539647,73.315612522751,13.8149757075223));
#56275=CARTESIAN_POINT('Ctrl Pts',(14.7121555666731,73.3259372675668,13.7538473672929));
#56276=CARTESIAN_POINT('Ctrl Pts',(14.707509166266,73.336379808103,13.6920216096451));
#56277=CARTESIAN_POINT('Ctrl Pts',(14.7028627658589,73.343394642505,13.6296869111642));
#56278=CARTESIAN_POINT('Ctrl Pts',(14.6982163654517,73.3469630837017,13.5672517752208));
#56279=CARTESIAN_POINT('Ctrl Pts',(14.6935699650446,73.3505315248984,13.5048166392774));
#56280=CARTESIAN_POINT('Ctrl Pts',(14.6889235646375,73.3506536342372,13.4422815959432));
#56281=CARTESIAN_POINT('Ctrl Pts',(14.6842771642304,73.3473647645392,13.3800512597816));
#56282=CARTESIAN_POINT('Ctrl Pts',(14.6796735451174,73.3441061767993,13.3183939035797));
#56283=CARTESIAN_POINT('Ctrl Pts',(14.6750699260045,73.3374863237172,13.256791804077));
#56284=CARTESIAN_POINT('Ctrl Pts',(14.6704663068915,73.3275121922856,13.1956400026169));
#56285=CARTESIAN_POINT('Ctrl Pts',(14.6658540328215,73.3175193091552,13.1343732337361));
#56286=CARTESIAN_POINT('Ctrl Pts',(14.6612417587516,73.3041595013438,13.0735589715084));
#56287=CARTESIAN_POINT('Ctrl Pts',(14.6566294846816,73.2874923525458,13.0135927900321));
#56288=CARTESIAN_POINT('Ctrl Pts',(14.6520381171708,73.2709007527565,12.953898423827));
#56289=CARTESIAN_POINT('Ctrl Pts',(14.6474467496601,73.2510318408939,12.8950449644891));
#56290=CARTESIAN_POINT('Ctrl Pts',(14.6428553821494,73.2279956529882,12.8374133776764));
#56291=CARTESIAN_POINT('Ctrl Pts',(14.6382667260684,73.2049730690915,12.7798158251677));
#56292=CARTESIAN_POINT('Ctrl Pts',(14.6336780699874,73.1787871065311,12.7234391843144));
#56293=CARTESIAN_POINT('Ctrl Pts',(14.6290894139064,73.1495969370155,12.6686471374774));
#56294=CARTESIAN_POINT('Ctrl Pts',(14.6245017964041,73.1204133742902,12.6138674920607));
#56295=CARTESIAN_POINT('Ctrl Pts',(14.6199141789018,73.0882271932799,12.5606721760087));
#56296=CARTESIAN_POINT('Ctrl Pts',(14.6153265613995,73.0532438821944,12.5094009999132));
#56297=CARTESIAN_POINT('Ctrl Pts',(14.6106969920505,73.0179406633348,12.4576609703183));
#56298=CARTESIAN_POINT('Ctrl Pts',(14.6060674227015,72.9797891625929,12.4078809045185));
#56299=CARTESIAN_POINT('Ctrl Pts',(14.6014378533525,72.9390444113478,12.3603789058474));
#56300=CARTESIAN_POINT('Ctrl Pts',(14.5968445129989,72.8986185107977,12.3132486371493));
#56301=CARTESIAN_POINT('Ctrl Pts',(14.5922511726452,72.8556402011786,12.2683612386279));
#56302=CARTESIAN_POINT('Ctrl Pts',(14.5876578322916,72.8103964656305,12.2259911291842));
#56303=CARTESIAN_POINT('Ctrl Pts',(14.5830101484449,72.7646174545664,12.1831197418968));
#56304=CARTESIAN_POINT('Ctrl Pts',(14.5783624645983,72.7165194588078,12.1428259543845));
#56305=CARTESIAN_POINT('Ctrl Pts',(14.5737147807516,72.6664330419732,12.1053511943365));
#56306=CARTESIAN_POINT('Ctrl Pts',(14.5690670969049,72.6163466251387,12.0678764342884));
#56307=CARTESIAN_POINT('Ctrl Pts',(14.5644194130582,72.5642722641935,12.0332209438036));
#56308=CARTESIAN_POINT('Ctrl Pts',(14.5597717292116,72.5105671637858,12.0015788702464));
#56309=CARTESIAN_POINT('Ctrl Pts',(14.5551668265409,72.4573564101171,11.9702280568444));
#56310=CARTESIAN_POINT('Ctrl Pts',(14.5505619238703,72.4023343486674,11.9417113462341));
#56311=CARTESIAN_POINT('Ctrl Pts',(14.5459570211996,72.3458343412366,11.9162411483063));
#56312=CARTESIAN_POINT('Ctrl Pts',(14.5413449075743,72.2892458587566,11.8907310658349));
#56313=CARTESIAN_POINT('Ctrl Pts',(14.536732793949,72.2311752148467,11.8682773441838));
#56314=CARTESIAN_POINT('Ctrl Pts',(14.5321206803237,72.1719849151098,11.8490486858703));
#56315=CARTESIAN_POINT('Ctrl Pts',(14.5275280398947,72.1130445277594,11.8299012145065));
#56316=CARTESIAN_POINT('Ctrl Pts',(14.5229353994657,72.0529943950421,11.8139518123152));
#56317=CARTESIAN_POINT('Ctrl Pts',(14.5183427590366,71.9922130427281,11.8013192189656));
#56318=CARTESIAN_POINT('Ctrl Pts',(14.5137528376327,71.9314676753825,11.7886941046116));
#56319=CARTESIAN_POINT('Ctrl Pts',(14.5091629162287,71.8699924424387,11.7793820076052));
#56320=CARTESIAN_POINT('Ctrl Pts',(14.5045729948247,71.8081786019903,11.7734511612293));
#56321=CARTESIAN_POINT('Ctrl Pts',(14.4999841216952,71.7463788789666,11.7675216693766));
#56322=CARTESIAN_POINT('Ctrl Pts',(14.4953952485657,71.6842412064689,11.764971943071));
#56323=CARTESIAN_POINT('Ctrl Pts',(14.4908063754362,71.6221625296889,11.7658184205979));
#56324=CARTESIAN_POINT('Ctrl Pts',(14.4861780353326,71.5595499402336,11.7666721783231));
#56325=CARTESIAN_POINT('Ctrl Pts',(14.481549695229,71.4969978898257,11.7709808662977));
#56326=CARTESIAN_POINT('Ctrl Pts',(14.4769213551254,71.4349119549069,11.7787077075583));
#56327=CARTESIAN_POINT('Ctrl Pts',(14.4723267972193,71.3732791844643,11.7863781506993));
#56328=CARTESIAN_POINT('Ctrl Pts',(14.4677322393132,71.312106243243,11.7974168674359));
#56329=CARTESIAN_POINT('Ctrl Pts',(14.4631376814072,71.251780603494,11.8117362675695));
#56330=CARTESIAN_POINT('Ctrl Pts',(14.4584924502048,71.1907896333514,11.8262135961092));
#56331=CARTESIAN_POINT('Ctrl Pts',(14.4538472190024,71.1306652827134,11.8440442820284));
#56332=CARTESIAN_POINT('Ctrl Pts',(14.4492019878,71.0717907212702,11.8650865347456));
#56333=CARTESIAN_POINT('Ctrl Pts',(14.4445567565976,71.0129161598269,11.8861287874627));
#56334=CARTESIAN_POINT('Ctrl Pts',(14.4399115253952,70.9552918509495,11.9103823446695));
#56335=CARTESIAN_POINT('Ctrl Pts',(14.4352662941928,70.8992763763392,11.9376572270489));
#56336=CARTESIAN_POINT('Ctrl Pts',(14.4306615361222,70.8437489553025,11.9646944678855));
#56337=CARTESIAN_POINT('Ctrl Pts',(14.4260567780516,70.7895836007335,11.9948070939335));
#56338=CARTESIAN_POINT('Ctrl Pts',(14.4214520199811,70.7371414975494,12.0278345003689));
#56339=CARTESIAN_POINT('Ctrl Pts',(14.4168398882808,70.6846154184768,12.0609147938098));
#56340=CARTESIAN_POINT('Ctrl Pts',(14.4122277565805,70.6338185941214,12.0969190279969));
#56341=CARTESIAN_POINT('Ctrl Pts',(14.4076156248802,70.5850918980863,12.1356381432999));
#56342=CARTESIAN_POINT('Ctrl Pts',(14.4030230932803,70.5365722750922,12.1741927146136));
#56343=CARTESIAN_POINT('Ctrl Pts',(14.3984305616805,70.490105637244,12.215438844973));
#56344=CARTESIAN_POINT('Ctrl Pts',(14.3938380300807,70.4460000194499,12.2591265457297));
#56345=CARTESIAN_POINT('Ctrl Pts',(14.3892482038997,70.4019203838768,12.3027885104566));
#56346=CARTESIAN_POINT('Ctrl Pts',(14.3846583777187,70.3601993694717,12.3488888369503));
#56347=CARTESIAN_POINT('Ctrl Pts',(14.3800685515377,70.3211099353246,12.3971390303482));
#56348=CARTESIAN_POINT('Ctrl Pts',(14.3754797599858,70.2820293126359,12.4453783472886));
#56349=CARTESIAN_POINT('Ctrl Pts',(14.3708909684338,70.2455794112319,12.4957661749858));
#56350=CARTESIAN_POINT('Ctrl Pts',(14.3663021768819,70.211993149495,12.5479806745381));
#56351=CARTESIAN_POINT('Ctrl Pts',(14.3616737337395,70.1781166700228,12.6006463577894));
#56352=CARTESIAN_POINT('Ctrl Pts',(14.3570452905972,70.1471538701477,12.6551700120064));
#56353=CARTESIAN_POINT('Ctrl Pts',(14.3524168474549,70.1192980902112,12.7111931757429));
#56354=CARTESIAN_POINT('Ctrl Pts',(14.3478223372381,70.0916465318836,12.766805611772));
#56355=CARTESIAN_POINT('Ctrl Pts',(14.3432278270213,70.0670567385342,12.8238951491533));
#56356=CARTESIAN_POINT('Ctrl Pts',(14.3386333168044,70.0456696681031,12.8820903974172));
#56357=CARTESIAN_POINT('Ctrl Pts',(14.3339879071994,70.0240456651701,12.9409303504252));
#56358=CARTESIAN_POINT('Ctrl Pts',(14.3293424975943,70.0056959548617,13.0009001610863));
#56359=CARTESIAN_POINT('Ctrl Pts',(14.3246970879893,69.9907139442805,13.0616020413769));
#56360=CARTESIAN_POINT('Ctrl Pts',(14.3200516783842,69.9757319336994,13.1223039216675));
#56361=CARTESIAN_POINT('Ctrl Pts',(14.3154062687791,69.964117659956,13.1837373402832));
#56362=CARTESIAN_POINT('Ctrl Pts',(14.3107608591741,69.9559107672478,13.2454984008646));
#56363=CARTESIAN_POINT('Ctrl Pts',(14.3061611205119,69.9477845598957,13.3066522629185));
#56364=CARTESIAN_POINT('Ctrl Pts',(14.3015613818498,69.9429667228472,13.3683702260757));
#56365=CARTESIAN_POINT('Ctrl Pts',(14.2969616431876,69.9415232932443,13.4302633195206));
#56366=CARTESIAN_POINT('Ctrl Pts',(14.2923488840613,69.9400757777304,13.4923316135295));
#56367=CARTESIAN_POINT('Ctrl Pts',(14.2877361249349,69.9420219261382,13.5545755284543));
#56368=CARTESIAN_POINT('Ctrl Pts',(14.2831233658086,69.9473761995002,13.6165947084177));
#56369=CARTESIAN_POINT('Ctrl Pts',(14.2785358895706,69.9527011256771,13.6782739564746));
#56370=CARTESIAN_POINT('Ctrl Pts',(14.2739484133326,69.9613968904335,13.7397304151198));
#56371=CARTESIAN_POINT('Ctrl Pts',(14.2693609370947,69.9734256073589,13.8005699108396));
#56372=CARTESIAN_POINT('Ctrl Pts',(14.2647761653569,69.9854472328759,13.86137353925));
#56373=CARTESIAN_POINT('Ctrl Pts',(14.2601913936191,70.0007978156185,13.9215604283667));
#56374=CARTESIAN_POINT('Ctrl Pts',(14.2556066218814,70.0193879899528,13.9807443379835));
#56375=CARTESIAN_POINT('Ctrl Pts',(14.2510228753126,70.0379740074674,14.0399150138973));
#56376=CARTESIAN_POINT('Ctrl Pts',(14.2464391287438,70.0597980259357,14.0980826709205));
#56377=CARTESIAN_POINT('Ctrl Pts',(14.241855382175,70.0847207610753,14.1548760097927));
#56378=CARTESIAN_POINT('Ctrl Pts',(14.23722205234,70.1099130902232,14.2122836931091));
#56379=CARTESIAN_POINT('Ctrl Pts',(14.232588722505,70.1382714009772,14.268286646983));
#56380=CARTESIAN_POINT('Ctrl Pts',(14.22795539267,70.1696027349112,14.3225240571129));
#56381=CARTESIAN_POINT('Ctrl Pts',(14.2233658460228,70.2006379997706,14.3762489445442));
#56382=CARTESIAN_POINT('Ctrl Pts',(14.2187762993756,70.2345900042183,14.42824111596));
#56383=CARTESIAN_POINT('Ctrl Pts',(14.2141867527284,70.2712272732066,14.478178631264));
#56384=CARTESIAN_POINT('Ctrl Pts',(14.2095315312995,70.3083888084951,14.5288307346667));
#56385=CARTESIAN_POINT('Ctrl Pts',(14.2048763098707,70.3483127374649,14.5773684850226));
#56386=CARTESIAN_POINT('Ctrl Pts',(14.2002210884418,70.3907166117566,14.6234922760323));
#56387=CARTESIAN_POINT('Ctrl Pts',(14.195565867013,70.4331204860483,14.6696160670419));
#56388=CARTESIAN_POINT('Ctrl Pts',(14.1909106455841,70.4780038747041,14.7133255692536));
#56389=CARTESIAN_POINT('Ctrl Pts',(14.1862554241553,70.5250491772928,14.7543632156284));
#56390=CARTESIAN_POINT('Ctrl Pts',(14.1816850784947,70.571236732025,14.7946526480205));
#56391=CARTESIAN_POINT('Ctrl Pts',(14.1771147328342,70.6196991503876,14.8325335042692));
#56392=CARTESIAN_POINT('Ctrl Pts',(14.1725443871736,70.6701535700373,14.8677371843251));
#56393=CARTESIAN_POINT('Ctrl Pts',(14.1679804721886,70.7205369981191,14.9028913312685));
#56394=CARTESIAN_POINT('Ctrl Pts',(14.1634165572037,70.7729064546098,14.9353754743146));
#56395=CARTESIAN_POINT('Ctrl Pts',(14.1588526422187,70.8269450467072,14.9649603088479));
#56396=CARTESIAN_POINT('Ctrl Pts',(14.154293423454,70.8809280336649,14.9945147008993));
#56397=CARTESIAN_POINT('Ctrl Pts',(14.1497342046893,70.9365763011329,15.0211754531287));
#56398=CARTESIAN_POINT('Ctrl Pts',(14.1451749859246,70.9935447046724,15.0447569684092));
#56399=CARTESIAN_POINT('Ctrl Pts',(14.1406177721829,71.0504880550248,15.0683281131671));
#56400=CARTESIAN_POINT('Ctrl Pts',(14.1360605584412,71.1087499187007,15.0888225003503));
#56401=CARTESIAN_POINT('Ctrl Pts',(14.1315033446995,71.1679630181875,15.1061016973274));
#56402=CARTESIAN_POINT('Ctrl Pts',(14.1269474062919,71.227159546917,15.1233760587296));
#56403=CARTESIAN_POINT('Ctrl Pts',(14.1223914678843,71.2873062868815,15.1374368764556));
#56404=CARTESIAN_POINT('Ctrl Pts',(14.1178355294766,71.3480208531988,15.1481956020225));
#56405=CARTESIAN_POINT('Ctrl Pts',(14.1132769416049,71.4087707275143,15.1589605842275));
#56406=CARTESIAN_POINT('Ctrl Pts',(14.1087183537331,71.4700885788062,15.1664195531591));
#56407=CARTESIAN_POINT('Ctrl Pts',(14.1041597658614,71.5315834484369,15.1705353945715));
#56408=CARTESIAN_POINT('Ctrl Pts',(14.101318205431,71.5699157989656,15.1731009724268));
#56409=CARTESIAN_POINT('Ctrl Pts',(14.0984766450006,71.6083168025979,15.1743685912238));
#56410=CARTESIAN_POINT('Ctrl Pts',(14.0956350845702,71.6466915577646,15.1743395106253));
#56411=CARTESIAN_POINT('',(13.9390000020058,73.2573116306334,14.0236386281943));
#56412=CARTESIAN_POINT('Ctrl Pts',(14.0956350845187,71.6466915584598,15.1743395106248));
#56413=CARTESIAN_POINT('Ctrl Pts',(14.0899102231617,71.7240047665774,15.174280922223));
#56414=CARTESIAN_POINT('Ctrl Pts',(14.0841853618047,71.8010986838953,15.1689576896067));
#56415=CARTESIAN_POINT('Ctrl Pts',(14.0784605004477,71.8773531425193,15.1584823289793));
#56416=CARTESIAN_POINT('Ctrl Pts',(14.0728903300106,71.9515471368597,15.148290022049));
#56417=CARTESIAN_POINT('Ctrl Pts',(14.0673201595735,72.0249466919968,15.1332206059659));
#56418=CARTESIAN_POINT('Ctrl Pts',(14.0617499891365,72.0969995652456,15.1134210258695));
#56419=CARTESIAN_POINT('Ctrl Pts',(14.0571556162791,72.1564300205421,15.0970899899683));
#56420=CARTESIAN_POINT('Ctrl Pts',(14.0525612434217,72.2150920063269,15.0774984774246));
#56421=CARTESIAN_POINT('Ctrl Pts',(14.0479668705642,72.2726022507899,15.0547372565205));
#56422=CARTESIAN_POINT('Ctrl Pts',(14.0433801850032,72.3300162692153,15.0320141196502));
#56423=CARTESIAN_POINT('Ctrl Pts',(14.0387934994422,72.3862819023425,15.0061319904094));
#56424=CARTESIAN_POINT('Ctrl Pts',(14.0342068138811,72.4410305366652,14.9772315299004));
#56425=CARTESIAN_POINT('Ctrl Pts',(14.0296244126719,72.4957280311387,14.9483580648627));
#56426=CARTESIAN_POINT('Ctrl Pts',(14.0250420114626,72.5489108869029,14.9164720935188));
#56427=CARTESIAN_POINT('Ctrl Pts',(14.0204596102533,72.6002315075143,14.8817618878047));
#56428=CARTESIAN_POINT('Ctrl Pts',(14.015879802325,72.6515230846649,14.8470713253547));
#56429=CARTESIAN_POINT('Ctrl Pts',(14.0112999943968,72.7009540952428,14.8095599829552));
#56430=CARTESIAN_POINT('Ctrl Pts',(14.0067201864685,72.7482043460189,14.7694604303333));
#56431=CARTESIAN_POINT('Ctrl Pts',(14.0021412843155,72.7954452518376,14.7293688084334));
#56432=CARTESIAN_POINT('Ctrl Pts',(13.9975623821625,72.8405058661429,14.6866903225734));
#56433=CARTESIAN_POINT('Ctrl Pts',(13.9929834800095,72.883099252963,14.6416976550351));
#56434=CARTESIAN_POINT('Ctrl Pts',(13.9884005179902,72.9257304050486,14.5966650949181));
#56435=CARTESIAN_POINT('Ctrl Pts',(13.9838175559709,72.9658896065511,14.5493146232578));
#56436=CARTESIAN_POINT('Ctrl Pts',(13.9792345939516,73.0033278615039,14.4999547361663));
#56437=CARTESIAN_POINT('Ctrl Pts',(13.9746497437218,73.0407815412642,14.4505745124765));
#56438=CARTESIAN_POINT('Ctrl Pts',(13.9700648934919,73.0755117530719,14.3991836455102));
#56439=CARTESIAN_POINT('Ctrl Pts',(13.9654800432621,73.1073126056581,14.3461200654122));
#56440=CARTESIAN_POINT('Ctrl Pts',(13.9608866089702,73.1391729979194,14.292957136144));
#56441=CARTESIAN_POINT('Ctrl Pts',(13.9562931746783,73.1680928320662,14.2381156874062));
#56442=CARTESIAN_POINT('Ctrl Pts',(13.9516997403865,73.1939123920431,14.1819580094984));
#56443=CARTESIAN_POINT('Ctrl Pts',(13.9474664942596,73.2177073448659,14.1302038627333));
#56444=CARTESIAN_POINT('Ctrl Pts',(13.9432332481327,73.2388696027766,14.0773323512853));
#56445=CARTESIAN_POINT('Ctrl Pts',(13.9390000020058,73.2573116306334,14.0236386281943));
#56446=CARTESIAN_POINT('',(13.939,72.0984538423728,15.1130207093982));
#56447=CARTESIAN_POINT('Origin',(13.939,71.6454,13.47));
#56448=CARTESIAN_POINT('',(13.9729899143421,71.6451742442358,15.171860356376));
#56449=CARTESIAN_POINT('Ctrl Pts',(13.939,72.0984538423728,15.1130207093982));
#56450=CARTESIAN_POINT('Ctrl Pts',(13.9447857228067,72.0232055254717,15.1337700151793));
#56451=CARTESIAN_POINT('Ctrl Pts',(13.9505714456135,71.9465687943793,15.1493352443956));
#56452=CARTESIAN_POINT('Ctrl Pts',(13.9563571684203,71.8691762668991,15.1595854574341));
#56453=CARTESIAN_POINT('Ctrl Pts',(13.9619014045005,71.7950139785347,15.1694078431334));
#56454=CARTESIAN_POINT('Ctrl Pts',(13.9674456405806,71.720157559446,15.1743499093407));
#56455=CARTESIAN_POINT('Ctrl Pts',(13.9729898766608,71.6451744249067,15.1743399850722));
#56456=CARTESIAN_POINT('',(14.766739959622,71.6442542797994,15.1740410878602));
#56457=CARTESIAN_POINT('Ctrl Pts',(13.9729899154298,71.6451742390203,15.1717887764722));
#56458=CARTESIAN_POINT('Ctrl Pts',(14.0031617552928,71.2377257485833,15.1690257382362));
#56459=CARTESIAN_POINT('Ctrl Pts',(14.0748354068288,70.2684391229546,14.8219893666021));
#56460=CARTESIAN_POINT('Ctrl Pts',(14.1880108700375,69.6552364071702,13.2070658961577));
#56461=CARTESIAN_POINT('Ctrl Pts',(14.3125163050564,70.7660383371287,11.6669646452173));
#56462=CARTESIAN_POINT('Ctrl Pts',(14.4370217400751,72.6622260268806,11.7404213989368));
#56463=CARTESIAN_POINT('Ctrl Pts',(14.5615271750938,73.6490321077662,13.362480576396));
#56464=CARTESIAN_POINT('Ctrl Pts',(14.6714332335455,72.9363884810012,14.879191736923));
#56465=CARTESIAN_POINT('Ctrl Pts',(14.7398374803241,72.0080403161166,15.1703558387755));
#56466=CARTESIAN_POINT('Ctrl Pts',(14.7667399154298,71.6442558079889,15.1726571393383));
#56467=CARTESIAN_POINT('',(15.5604899154688,71.6456305596758,15.1743399844052));
#56468=CARTESIAN_POINT('Ctrl Pts',(14.7667399691545,71.6442539501588,15.1743396146806));
#56469=CARTESIAN_POINT('Ctrl Pts',(14.7719829711192,71.5732864489064,15.1742918939724));
#56470=CARTESIAN_POINT('Ctrl Pts',(14.7772259730839,71.5024894639145,15.1698075684678));
#56471=CARTESIAN_POINT('Ctrl Pts',(14.7824689750485,71.4323729178381,15.160974363456));
#56472=CARTESIAN_POINT('Ctrl Pts',(14.787757410458,71.3616487740059,15.1520646139503));
#56473=CARTESIAN_POINT('Ctrl Pts',(14.7930458458675,71.2916171145709,15.1387304010231));
#56474=CARTESIAN_POINT('Ctrl Pts',(14.7983342812769,71.2227823845175,15.121111500379));
#56475=CARTESIAN_POINT('Ctrl Pts',(14.8024022025617,71.1698339712652,15.1075588528763));
#56476=CARTESIAN_POINT('Ctrl Pts',(14.8064701238466,71.1175934009965,15.0914720431421));
#56477=CARTESIAN_POINT('Ctrl Pts',(14.8105380451314,71.0662816943619,15.0729338176216));
#56478=CARTESIAN_POINT('Ctrl Pts',(14.8151416958287,71.0082124355223,15.0519541798978));
#56479=CARTESIAN_POINT('Ctrl Pts',(14.819745346526,70.9511696380993,15.0277734201126));
#56480=CARTESIAN_POINT('Ctrl Pts',(14.8243489972233,70.8955293886369,15.0005126271331));
#56481=CARTESIAN_POINT('Ctrl Pts',(14.8289612673452,70.8397849638209,14.9732007937148));
#56482=CARTESIAN_POINT('Ctrl Pts',(14.8335735374672,70.78544884212,14.9427975104087));
#56483=CARTESIAN_POINT('Ctrl Pts',(14.8381858075891,70.7328823826295,14.9094743601705));
#56484=CARTESIAN_POINT('Ctrl Pts',(14.8427771879991,70.6805540050749,14.8763021358308));
#56485=CARTESIAN_POINT('Ctrl Pts',(14.847368568409,70.6299797387178,14.8402366865257));
#56486=CARTESIAN_POINT('Ctrl Pts',(14.851959948819,70.5814923562384,14.8014936579442));
#56487=CARTESIAN_POINT('Ctrl Pts',(14.856548610765,70.533033682162,14.7627735683299));
#56488=CARTESIAN_POINT('Ctrl Pts',(14.861137272711,70.4866598370754,14.7213793595562));
#56489=CARTESIAN_POINT('Ctrl Pts',(14.865725934657,70.4426728224686,14.6775687028188));
#56490=CARTESIAN_POINT('Ctrl Pts',(14.8703135510013,70.3986958310231,14.6337680290566));
#56491=CARTESIAN_POINT('Ctrl Pts',(14.8749011673457,70.3571049493374,14.5875523585866));
#56492=CARTESIAN_POINT('Ctrl Pts',(14.87948878369,70.318165917844,14.5392167819313));
#56493=CARTESIAN_POINT('Ctrl Pts',(14.8841183417283,70.2788708912493,14.4904393034657));
#56494=CARTESIAN_POINT('Ctrl Pts',(14.8887478997666,70.2422768074236,14.4395033453739));
#56495=CARTESIAN_POINT('Ctrl Pts',(14.893377457805,70.2086142824763,14.3867451322587));
#56496=CARTESIAN_POINT('Ctrl Pts',(14.89797077985,70.1752152373298,14.334399862721));
#56497=CARTESIAN_POINT('Ctrl Pts',(14.902564101895,70.1447022241691,14.2802612397332));
#56498=CARTESIAN_POINT('Ctrl Pts',(14.90715742394,70.1172547941091,14.2246834205895));
#56499=CARTESIAN_POINT('Ctrl Pts',(14.911805099975,70.0894825713773,14.1684479344682));
#56500=CARTESIAN_POINT('Ctrl Pts',(14.9164527760101,70.0648491854927,14.1107394511286));
#56501=CARTESIAN_POINT('Ctrl Pts',(14.9211004520451,70.043489991238,14.0519442923754));
#56502=CARTESIAN_POINT('Ctrl Pts',(14.9257481280801,70.0221307969833,13.9931491336223));
#56503=CARTESIAN_POINT('Ctrl Pts',(14.9303958041151,70.0040458880126,13.933267826093));
#56504=CARTESIAN_POINT('Ctrl Pts',(14.9350434801501,69.9893176493714,13.8726985020292));
#56505=CARTESIAN_POINT('Ctrl Pts',(14.9396477604633,69.9747269294693,13.8126947185755));
#56506=CARTESIAN_POINT('Ctrl Pts',(14.9442520407764,69.9633726913063,13.7517783712946));
#56507=CARTESIAN_POINT('Ctrl Pts',(14.9488563210896,69.9553616753097,13.6903299722646));
#56508=CARTESIAN_POINT('Ctrl Pts',(14.9534685125096,69.9473368947291,13.6287759921632));
#56509=CARTESIAN_POINT('Ctrl Pts',(14.9580807039295,69.9426670021147,13.5666886161985));
#56510=CARTESIAN_POINT('Ctrl Pts',(14.9626928953495,69.9414084847753,13.5044637728968));
#56511=CARTESIAN_POINT('Ctrl Pts',(14.967284925864,69.9401554686927,13.4425109281029));
#56512=CARTESIAN_POINT('Ctrl Pts',(14.9718769563785,69.9422841044234,13.3804223235053));
#56513=CARTESIAN_POINT('Ctrl Pts',(14.976468986893,69.9477983883997,13.3185945711275));
#56514=CARTESIAN_POINT('Ctrl Pts',(14.9810583047522,69.9533094149169,13.2568033423269));
#56515=CARTESIAN_POINT('Ctrl Pts',(14.9856476226114,69.9622020782475,13.1952731643083));
#56516=CARTESIAN_POINT('Ctrl Pts',(14.9902369404706,69.9744283455657,13.1343982037041));
#56517=CARTESIAN_POINT('Ctrl Pts',(14.9948252174018,69.9866518397781,13.0735370504784));
#56518=CARTESIAN_POINT('Ctrl Pts',(14.999413494333,70.0022073366833,13.0133313165563));
#56519=CARTESIAN_POINT('Ctrl Pts',(15.0040017712643,70.0209955822639,12.9541656048311));
#56520=CARTESIAN_POINT('Ctrl Pts',(15.008630699923,70.0399502900372,12.8944756901369));
#56521=CARTESIAN_POINT('Ctrl Pts',(15.0132596285817,70.0621951881863,12.8358448276789));
#56522=CARTESIAN_POINT('Ctrl Pts',(15.0178885572404,70.0875774671697,12.7786507454216));
#56523=CARTESIAN_POINT('Ctrl Pts',(15.0224825436428,70.112768143697,12.7218884024357));
#56524=CARTESIAN_POINT('Ctrl Pts',(15.0270765300451,70.1410487119256,12.666541653862));
#56525=CARTESIAN_POINT('Ctrl Pts',(15.0316705164474,70.172223086198,12.6129558843088));
#56526=CARTESIAN_POINT('Ctrl Pts',(15.0363169162344,70.2037531329355,12.5587587477854));
#56527=CARTESIAN_POINT('Ctrl Pts',(15.0409633160213,70.2382431576301,12.5063634811408));
#56528=CARTESIAN_POINT('Ctrl Pts',(15.0456097158082,70.2754461663039,12.4560959960917));
#56529=CARTESIAN_POINT('Ctrl Pts',(15.0502561155951,70.3126491749777,12.4058285110425));
#56530=CARTESIAN_POINT('Ctrl Pts',(15.054902515382,70.3525647813502,12.357689175729));
#56531=CARTESIAN_POINT('Ctrl Pts',(15.0595489151689,70.3949069468999,12.3119663391126));
#56532=CARTESIAN_POINT('Ctrl Pts',(15.0641531360115,70.4368647400483,12.2666585638487));
#56533=CARTESIAN_POINT('Ctrl Pts',(15.0687573568541,70.481370989419,12.2235445099839));
#56534=CARTESIAN_POINT('Ctrl Pts',(15.0733615776967,70.5281674762515,12.1829233420349));
#56535=CARTESIAN_POINT('Ctrl Pts',(15.0779737765505,70.5750450501797,12.1422317873378));
#56536=CARTESIAN_POINT('Ctrl Pts',(15.0825859754043,70.6242204927978,12.1040421730639));
#56537=CARTESIAN_POINT('Ctrl Pts',(15.0871981742581,70.6753949616811,12.0686203008335));
#56538=CARTESIAN_POINT('Ctrl Pts',(15.0917901472714,70.7263450155555,12.0333537638698));
#56539=CARTESIAN_POINT('Ctrl Pts',(15.0963821202846,70.7792761970361,12.0008310574532));
#56540=CARTESIAN_POINT('Ctrl Pts',(15.1009740932979,70.8338601108457,11.9712745935591));
#56541=CARTESIAN_POINT('Ctrl Pts',(15.1055633545697,70.888411790698,11.9417355839245));
#56542=CARTESIAN_POINT('Ctrl Pts',(15.1101526158415,70.944613822131,11.915159583856));
#56543=CARTESIAN_POINT('Ctrl Pts',(15.1147418771134,71.002111107896,11.8917242836261));
#56544=CARTESIAN_POINT('Ctrl Pts',(15.1193300984737,71.0595953649657,11.8682942937579));
#56545=CARTESIAN_POINT('Ctrl Pts',(15.1239183198341,71.1183738240929,11.8480037818434));
#56546=CARTESIAN_POINT('Ctrl Pts',(15.1285065411944,71.1780710663744,11.8309824578741));
#56547=CARTESIAN_POINT('Ctrl Pts',(15.1331355252772,71.238298671497,11.813809912887));
#56548=CARTESIAN_POINT('Ctrl Pts',(15.13776450936,71.2994609717384,11.799965109451));
#56549=CARTESIAN_POINT('Ctrl Pts',(15.1423934934427,71.361158667484,11.7895293217406));
#56550=CARTESIAN_POINT('Ctrl Pts',(15.1469874274447,71.4223891960973,11.7791725524921));
#56551=CARTESIAN_POINT('Ctrl Pts',(15.1515813614467,71.4841465228903,11.7721733515128));
#56552=CARTESIAN_POINT('Ctrl Pts',(15.1561752954487,71.5460344327724,11.7685590460878));
#56553=CARTESIAN_POINT('Ctrl Pts',(15.1608218045719,71.6086306167306,11.7649033768676));
#56554=CARTESIAN_POINT('Ctrl Pts',(15.1654683136951,71.6713598596993,11.7647105911223));
#56555=CARTESIAN_POINT('Ctrl Pts',(15.1701148228182,71.7338140167254,11.7679548192699));
#56556=CARTESIAN_POINT('Ctrl Pts',(15.1747613319414,71.7962681737516,11.7711990474176));
#56557=CARTESIAN_POINT('Ctrl Pts',(15.1794078410646,71.8584467244815,11.7778801707693));
#56558=CARTESIAN_POINT('Ctrl Pts',(15.1840543501877,71.9199512711816,11.787919016488));
#56559=CARTESIAN_POINT('Ctrl Pts',(15.1886584522427,71.9808944873354,11.7978662411633));
#56560=CARTESIAN_POINT('Ctrl Pts',(15.1932625542977,72.0414169105433,11.8111494280926));
#56561=CARTESIAN_POINT('Ctrl Pts',(15.1978666563527,72.1011265402971,11.8277186123965));
#56562=CARTESIAN_POINT('Ctrl Pts',(15.202478870055,72.1609413682952,11.844316988794));
#56563=CARTESIAN_POINT('Ctrl Pts',(15.2070910837572,72.2199400235554,11.8642129166003));
#56564=CARTESIAN_POINT('Ctrl Pts',(15.2117032974595,72.2777358385527,11.887304128115));
#56565=CARTESIAN_POINT('Ctrl Pts',(15.2162951457023,72.335276453249,11.9102933792346));
#56566=CARTESIAN_POINT('Ctrl Pts',(15.2208869939451,72.3916243448091,11.9364495923407));
#56567=CARTESIAN_POINT('Ctrl Pts',(15.2254788421879,72.4464127216951,11.9656219041469));
#56568=CARTESIAN_POINT('Ctrl Pts',(15.2300679768008,72.5011687204691,11.9947769760853));
#56569=CARTESIAN_POINT('Ctrl Pts',(15.2346571114137,72.5543665855262,12.0269443738947));
#56570=CARTESIAN_POINT('Ctrl Pts',(15.2392462460267,72.6056620523399,12.0619262709517));
#56571=CARTESIAN_POINT('Ctrl Pts',(15.2438343390567,72.656945876767,12.0969002282668));
#56572=CARTESIAN_POINT('Ctrl Pts',(15.2484224320868,72.7063277415258,12.1346871306779));
#56573=CARTESIAN_POINT('Ctrl Pts',(15.2530105251169,72.7534921503756,12.175045706646));
#56574=CARTESIAN_POINT('Ctrl Pts',(15.2576396301243,72.8010781517384,12.2157650392499));
#56575=CARTESIAN_POINT('Ctrl Pts',(15.2622687351318,72.8464064356783,12.25910193594));
#56576=CARTESIAN_POINT('Ctrl Pts',(15.2668978401393,72.8891886426184,12.3047684143942));
#56577=CARTESIAN_POINT('Ctrl Pts',(15.2714916431915,72.9316445887475,12.3500866363334));
#56578=CARTESIAN_POINT('Ctrl Pts',(15.2760854462438,72.9715928707069,12.3976986006646));
#56579=CARTESIAN_POINT('Ctrl Pts',(15.280679249296,73.0087918493918,12.4472891412467));
#56580=CARTESIAN_POINT('Ctrl Pts',(15.2853260052811,73.0464196220407,12.497451313772));
#56581=CARTESIAN_POINT('Ctrl Pts',(15.2899727612662,73.0812339932799,12.549637535583));
#56582=CARTESIAN_POINT('Ctrl Pts',(15.2946195172513,73.113031030015,12.6034932225671));
#56583=CARTESIAN_POINT('Ctrl Pts',(15.2992662732363,73.1448280667501,12.6573489095512));
#56584=CARTESIAN_POINT('Ctrl Pts',(15.3039130292214,73.1736075803916,12.7128735621519));
#56585=CARTESIAN_POINT('Ctrl Pts',(15.3085597852065,73.1992154713234,12.7696912704556));
#56586=CARTESIAN_POINT('Ctrl Pts',(15.3131639657683,73.2245887325911,12.8259883923568));
#56587=CARTESIAN_POINT('Ctrl Pts',(15.3177681463301,73.246948614108,12.8837775277029));
#56588=CARTESIAN_POINT('Ctrl Pts',(15.3223723268919,73.2661202331561,12.942704294121));
#56589=CARTESIAN_POINT('Ctrl Pts',(15.3269845307808,73.2853252610092,13.0017337473723));
#56590=CARTESIAN_POINT('Ctrl Pts',(15.3315967346697,73.3013306509221,13.0619043533235));
#56591=CARTESIAN_POINT('Ctrl Pts',(15.3362089385586,73.3140080727277,13.1228373072639));
#56592=CARTESIAN_POINT('Ctrl Pts',(15.3408008680718,73.3266297669858,13.1835024114678));
#56593=CARTESIAN_POINT('Ctrl Pts',(15.3453927975851,73.3359525592773,13.2449226827745));
#56594=CARTESIAN_POINT('Ctrl Pts',(15.3499847270984,73.3418995996425,13.3067090204182));
#56595=CARTESIAN_POINT('Ctrl Pts',(15.354573943784,73.3478431266055,13.3684588558289));
#56596=CARTESIAN_POINT('Ctrl Pts',(15.3591631604697,73.3504148083483,13.430573824812));
#56597=CARTESIAN_POINT('Ctrl Pts',(15.3637523771554,73.349589386739,13.4926576637407));
#56598=CARTESIAN_POINT('Ctrl Pts',(15.3683405529185,73.3487641523512,13.5547274208618));
#56599=CARTESIAN_POINT('Ctrl Pts',(15.3729287286817,73.34454335145,13.6167655550409));
#56600=CARTESIAN_POINT('Ctrl Pts',(15.3775169044448,73.3369538322894,13.6783757857026));
#56601=CARTESIAN_POINT('Ctrl Pts',(15.3821459307598,73.3292967402932,13.7405345594138));
#56602=CARTESIAN_POINT('Ctrl Pts',(15.3867749570749,73.3182106749259,13.8022572477504));
#56603=CARTESIAN_POINT('Ctrl Pts',(15.3914039833899,73.3037764025269,13.8631444303841));
#56604=CARTESIAN_POINT('Ctrl Pts',(15.3959978698321,73.2894517036023,13.9235694061282));
#56605=CARTESIAN_POINT('Ctrl Pts',(15.4005917562743,73.2718296576399,13.9831710408981));
#56606=CARTESIAN_POINT('Ctrl Pts',(15.4051856427165,73.2510395064569,14.0415738018005));
#56607=CARTESIAN_POINT('Ctrl Pts',(15.409832238968,73.2300108110877,14.1006466703395));
#56608=CARTESIAN_POINT('Ctrl Pts',(15.4144788352194,73.205741036146,14.1584924808248));
#56609=CARTESIAN_POINT('Ctrl Pts',(15.4191254314709,73.178413080281,14.2147454137404));
#56610=CARTESIAN_POINT('Ctrl Pts',(15.4237720277223,73.151085124416,14.270998346656));
#56611=CARTESIAN_POINT('Ctrl Pts',(15.4284186239738,73.1206992997734,14.3256579689713));
#56612=CARTESIAN_POINT('Ctrl Pts',(15.4330652202252,73.0874838004644,14.3783882143875));
#56613=CARTESIAN_POINT('Ctrl Pts',(15.4376693867961,73.0545716033901,14.4306369616596));
#56614=CARTESIAN_POINT('Ctrl Pts',(15.4422735533669,73.0187511318237,14.481198000377));
#56615=CARTESIAN_POINT('Ctrl Pts',(15.4468777199378,72.9802211865124,14.5297297936916));
#56616=CARTESIAN_POINT('Ctrl Pts',(15.4514899255755,72.9416239663092,14.5783463255419));
#56617=CARTESIAN_POINT('Ctrl Pts',(15.4561021312133,72.9003080344869,14.6249260610246));
#56618=CARTESIAN_POINT('Ctrl Pts',(15.460714336851,72.8565182678733,14.6691527745969));
#56619=CARTESIAN_POINT('Ctrl Pts',(15.4653062523124,72.8129211427332,14.7131849244635));
#56620=CARTESIAN_POINT('Ctrl Pts',(15.4698981677737,72.7668722415645,14.7548843308449));
#56621=CARTESIAN_POINT('Ctrl Pts',(15.4744900832351,72.7186534588276,14.7939719969526));
#56622=CARTESIAN_POINT('Ctrl Pts',(15.4790792858875,72.6704631627531,14.8330365708733));
#56623=CARTESIAN_POINT('Ctrl Pts',(15.4836684885399,72.6201059206686,14.8694921457964));
#56624=CARTESIAN_POINT('Ctrl Pts',(15.4882576911923,72.5678980969526,14.9030987742367));
#56625=CARTESIAN_POINT('Ctrl Pts',(15.4928458529655,72.5157021145166,14.9366977803425));
#56626=CARTESIAN_POINT('Ctrl Pts',(15.4974340147388,72.4616568102192,14.9674488487201));
#56627=CARTESIAN_POINT('Ctrl Pts',(15.5020221765121,72.4061073458497,14.9951554575093));
#56628=CARTESIAN_POINT('Ctrl Pts',(15.5066512164064,72.3500629648139,15.0231089176878));
#56629=CARTESIAN_POINT('Ctrl Pts',(15.5112802563007,72.2924879411894,15.0479631342202));
#56630=CARTESIAN_POINT('Ctrl Pts',(15.5159092961951,72.2337598447896,15.0695647935108));
#56631=CARTESIAN_POINT('Ctrl Pts',(15.52050316892,72.1754779102213,15.0910023433467));
#56632=CARTESIAN_POINT('Ctrl Pts',(15.5250970416448,72.1160608708911,15.1092364899732));
#56633=CARTESIAN_POINT('Ctrl Pts',(15.5296909143697,72.0558931552801,15.1241675263008));
#56634=CARTESIAN_POINT('Ctrl Pts',(15.5343375378488,71.9950345427799,15.1392700134879));
#56635=CARTESIAN_POINT('Ctrl Pts',(15.5389841613278,71.9334084238037,15.1509929319953));
#56636=CARTESIAN_POINT('Ctrl Pts',(15.5436307848069,71.8714207801692,15.1592866667714));
#56637=CARTESIAN_POINT('Ctrl Pts',(15.5482774082859,71.8094331365347,15.1675804015476));
#56638=CARTESIAN_POINT('Ctrl Pts',(15.552924031765,71.7470845016633,15.1724449735931));
#56639=CARTESIAN_POINT('Ctrl Pts',(15.557570655244,71.684781076219,15.1738849627941));
#56640=CARTESIAN_POINT('Ctrl Pts',(15.5585437419726,71.6717336156878,15.1741865224938));
#56641=CARTESIAN_POINT('Ctrl Pts',(15.5595168287012,71.6586826780926,15.1743382187369));
#56642=CARTESIAN_POINT('Ctrl Pts',(15.5604899154299,71.6456305601979,15.1743399844051));
#56643=CARTESIAN_POINT('',(16.3542399153822,71.6462368438886,15.1743397945516));
#56644=CARTESIAN_POINT('Ctrl Pts',(15.5604899154688,71.6456305596758,15.1743399844052));
#56645=CARTESIAN_POINT('Ctrl Pts',(15.5650762026696,71.5841141917248,15.1743483062154));
#56646=CARTESIAN_POINT('Ctrl Pts',(15.5696624898704,71.5224716406624,15.171021778295));
#56647=CARTESIAN_POINT('Ctrl Pts',(15.5742487770713,71.4610952352599,15.1643454751892));
#56648=CARTESIAN_POINT('Ctrl Pts',(15.5788273156343,71.399822526707,15.1576804518512));
#56649=CARTESIAN_POINT('Ctrl Pts',(15.5834058541973,71.3388155757472,15.1476769437711));
#56650=CARTESIAN_POINT('Ctrl Pts',(15.5879843927603,71.2784659257297,15.1343720199341));
#56651=CARTESIAN_POINT('Ctrl Pts',(15.5925586200818,71.2181731021245,15.1210796242739));
#56652=CARTESIAN_POINT('Ctrl Pts',(15.5971328474032,71.1585368501406,15.104492083317));
#56653=CARTESIAN_POINT('Ctrl Pts',(15.6017070747247,71.0999411665725,15.0846979583303));
#56654=CARTESIAN_POINT('Ctrl Pts',(15.6062786955914,71.0413788715929,15.0649151122954));
#56655=CARTESIAN_POINT('Ctrl Pts',(15.6108503164582,70.98385645321,15.0419294686012));
#56656=CARTESIAN_POINT('Ctrl Pts',(15.6154219373249,70.9277432952677,15.0158795844932));
#56657=CARTESIAN_POINT('Ctrl Pts',(15.6199926529081,70.8716412489911,14.9898348588473));
#56658=CARTESIAN_POINT('Ctrl Pts',(15.6245633684912,70.8169483728025,14.9607273133252));
#56659=CARTESIAN_POINT('Ctrl Pts',(15.6291340840744,70.7640126540446,14.9287430143756));
#56660=CARTESIAN_POINT('Ctrl Pts',(15.6337088025551,70.7110305757495,14.8967307045229));
#56661=CARTESIAN_POINT('Ctrl Pts',(15.6382835210358,70.6598091689236,14.8618368720041));
#56662=CARTESIAN_POINT('Ctrl Pts',(15.6428582395164,70.6106693274308,14.8242921659836));
#56663=CARTESIAN_POINT('Ctrl Pts',(15.6474348741354,70.561508903528,14.7867317342198));
#56664=CARTESIAN_POINT('Ctrl Pts',(15.6520115087544,70.5144321728164,14.7465185484755));
#56665=CARTESIAN_POINT('Ctrl Pts',(15.6565881433734,70.4697262601586,14.703923049889));
#56666=CARTESIAN_POINT('Ctrl Pts',(15.6611731743483,70.4249383294268,14.6612494050227));
#56667=CARTESIAN_POINT('Ctrl Pts',(15.6657582053233,70.3825302586924,14.6161850885475));
#56668=CARTESIAN_POINT('Ctrl Pts',(15.6703432362982,70.3427510441729,14.5690361838823));
#56669=CARTESIAN_POINT('Ctrl Pts',(15.6742541876198,70.3088200691273,14.5288189918904));
#56670=CARTESIAN_POINT('Ctrl Pts',(15.6781651389413,70.2768012186877,14.4870858181692));
#56671=CARTESIAN_POINT('Ctrl Pts',(15.6820760902628,70.2468237658147,14.4440427879575));
#56672=CARTESIAN_POINT('Ctrl Pts',(15.6866802550219,70.2115328299943,14.3933704101823));
#56673=CARTESIAN_POINT('Ctrl Pts',(15.691284419781,70.1789295745051,14.3406774457886));
#56674=CARTESIAN_POINT('Ctrl Pts',(15.6958885845401,70.1492510550151,14.2862800806223));
#56675=CARTESIAN_POINT('Ctrl Pts',(15.7005007904043,70.1195207024331,14.2317877112683));
#56676=CARTESIAN_POINT('Ctrl Pts',(15.7051129962685,70.092725642573,14.1755853749444));
#56677=CARTESIAN_POINT('Ctrl Pts',(15.7097252021328,70.0690616645609,14.118021826658));
#56678=CARTESIAN_POINT('Ctrl Pts',(15.7143171155079,70.0455018018095,14.0607115427987));
#56679=CARTESIAN_POINT('Ctrl Pts',(15.718909028883,70.0250457459363,14.0020524600338));
#56680=CARTESIAN_POINT('Ctrl Pts',(15.7235009422582,70.0078405740573,13.9424129148386));
#56681=CARTESIAN_POINT('Ctrl Pts',(15.728090142727,69.9906455670086,13.8828086047376));
#56682=CARTESIAN_POINT('Ctrl Pts',(15.7326793431958,69.9766977752377,13.8222254673645));
#56683=CARTESIAN_POINT('Ctrl Pts',(15.7372685436646,69.9660948804296,13.7610483653701));
#56684=CARTESIAN_POINT('Ctrl Pts',(15.7418567031604,69.9554943906868,13.6998851402398));
#56685=CARTESIAN_POINT('Ctrl Pts',(15.7464448626562,69.9482373778168,13.6381287175427));
#56686=CARTESIAN_POINT('Ctrl Pts',(15.751033022152,69.9443703084637,13.5761735565569));
#56687=CARTESIAN_POINT('Ctrl Pts',(15.7556620640795,69.9404687818955,13.5136663490179));
#56688=CARTESIAN_POINT('Ctrl Pts',(15.7602911060069,69.9400179785039,13.4509573647327));
#56689=CARTESIAN_POINT('Ctrl Pts',(15.7649201479344,69.9430119428877,13.3884540706023));
#56690=CARTESIAN_POINT('Ctrl Pts',(15.7695140181765,69.9459831589846,13.3264256795361));
#56691=CARTESIAN_POINT('Ctrl Pts',(15.7741078884186,69.952346866061,13.2646003691596));
#56692=CARTESIAN_POINT('Ctrl Pts',(15.7787017586607,69.9620450677426,13.2033710299972));
#56693=CARTESIAN_POINT('Ctrl Pts',(15.7833483864309,69.9718546467859,13.1414385128155));
#56694=CARTESIAN_POINT('Ctrl Pts',(15.787995014201,69.9850757024932,13.0801162666477));
#56695=CARTESIAN_POINT('Ctrl Pts',(15.7926416419712,70.0015957067538,13.0197975109959));
#56696=CARTESIAN_POINT('Ctrl Pts',(15.7972882697413,70.0181157110145,12.9594787553441));
#56697=CARTESIAN_POINT('Ctrl Pts',(15.8019348975115,70.0379344366011,12.9001639732733));
#56698=CARTESIAN_POINT('Ctrl Pts',(15.8065815252816,70.0608893599134,12.8422254647946));
#56699=CARTESIAN_POINT('Ctrl Pts',(15.8111856876317,70.0836344987306,12.7848164549592));
#56700=CARTESIAN_POINT('Ctrl Pts',(15.8157898499818,70.10954861961,12.7285316886502));
#56701=CARTESIAN_POINT('Ctrl Pts',(15.8203940123319,70.1384991038188,12.6737434303641));
#56702=CARTESIAN_POINT('Ctrl Pts',(15.8250062184972,70.1675001666843,12.6188594529017));
#56703=CARTESIAN_POINT('Ctrl Pts',(15.8296184246626,70.1995480678181,12.5654777103989));
#56704=CARTESIAN_POINT('Ctrl Pts',(15.8342306308279,70.2344602436447,12.5139540599238));
#56705=CARTESIAN_POINT('Ctrl Pts',(15.8388225417529,70.2692187942917,12.462657130639));
#56706=CARTESIAN_POINT('Ctrl Pts',(15.8434144526779,70.3068162023768,12.413202412115));
#56707=CARTESIAN_POINT('Ctrl Pts',(15.8480063636028,70.3470266736192,12.3659159719736));
#56708=CARTESIAN_POINT('Ctrl Pts',(15.8525955616132,70.3872133883956,12.3186574688018));
#56709=CARTESIAN_POINT('Ctrl Pts',(15.8571847596235,70.4300097767036,12.2735650890779));
#56710=CARTESIAN_POINT('Ctrl Pts',(15.8617739576338,70.475148982573,12.2309328541959));
#56711=CARTESIAN_POINT('Ctrl Pts',(15.8663621146672,70.5202779494261,12.188310289669));
#56712=CARTESIAN_POINT('Ctrl Pts',(15.8709502717005,70.5677483099836,12.1481471099338));
#56713=CARTESIAN_POINT('Ctrl Pts',(15.8755384287339,70.6172569178041,12.1106999455114));
#56714=CARTESIAN_POINT('Ctrl Pts',(15.8801674730311,70.6672067205304,12.0729190714796));
#56715=CARTESIAN_POINT('Ctrl Pts',(15.8847965173283,70.7192308819633,12.0379032049952));
#56716=CARTESIAN_POINT('Ctrl Pts',(15.8894255616255,70.7729864540195,12.0058724644384));
#56717=CARTESIAN_POINT('Ctrl Pts',(15.8940194294244,70.8263335329464,11.9740851281825));
#56718=CARTESIAN_POINT('Ctrl Pts',(15.8986132972232,70.8813853167274,11.9452378931465));
#56719=CARTESIAN_POINT('Ctrl Pts',(15.9032071650221,70.9377822618517,11.9194994446122));
#56720=CARTESIAN_POINT('Ctrl Pts',(15.9078537975685,70.9948269771555,11.8934653666002));
#56721=CARTESIAN_POINT('Ctrl Pts',(15.9125004301148,71.0532474624081,11.8706121550289));
#56722=CARTESIAN_POINT('Ctrl Pts',(15.9171470626612,71.1126537750681,11.8510632206844));
#56723=CARTESIAN_POINT('Ctrl Pts',(15.9217936952076,71.1720600877282,11.8315142863399));
#56724=CARTESIAN_POINT('Ctrl Pts',(15.9264403277539,71.2324516995971,11.8152697066516));
#56725=CARTESIAN_POINT('Ctrl Pts',(15.9310869603003,71.2934284890502,11.802399660866));
#56726=CARTESIAN_POINT('Ctrl Pts',(15.9356911216906,71.3538479383828,11.7896472498876));
#56727=CARTESIAN_POINT('Ctrl Pts',(15.9402952830808,71.4150807634737,11.7801574727491));
#56728=CARTESIAN_POINT('Ctrl Pts',(15.9448994444711,71.4767433933052,11.774025417461));
#56729=CARTESIAN_POINT('Ctrl Pts',(15.9495116507564,71.5385137668374,11.7678826475744));
#56730=CARTESIAN_POINT('Ctrl Pts',(15.9541238570418,71.6007149577268,11.7651094963736));
#56731=CARTESIAN_POINT('Ctrl Pts',(15.9587360633271,71.6629494823739,11.7657503553562));
#56732=CARTESIAN_POINT('Ctrl Pts',(15.9633279732294,71.7249101390122,11.7663883941876));
#56733=CARTESIAN_POINT('Ctrl Pts',(15.9679198831317,71.7869033274104,11.7704104814037));
#56734=CARTESIAN_POINT('Ctrl Pts',(15.9725117930339,71.8485325158393,11.7778085165653));
#56735=CARTESIAN_POINT('Ctrl Pts',(15.9771009900009,71.9101252932745,11.7852021809115));
#56736=CARTESIAN_POINT('Ctrl Pts',(15.9816901869678,71.971353994652,11.7959677772661));
#56737=CARTESIAN_POINT('Ctrl Pts',(15.9862793839347,72.0318261191956,11.8100452747128));
#56738=CARTESIAN_POINT('Ctrl Pts',(15.9908675399058,72.0922845264737,11.8241195788738));
#56739=CARTESIAN_POINT('Ctrl Pts',(15.9954556958768,72.1519862039588,11.8415041773498));
#56740=CARTESIAN_POINT('Ctrl Pts',(16.0000438518479,72.2105497726291,11.8620881336039));
#56741=CARTESIAN_POINT('Ctrl Pts',(16.0046728971372,72.2696352556394,11.8828555326056));
#56742=CARTESIAN_POINT('Ctrl Pts',(16.0093019424264,72.3275617374471,11.906879457176));
#56743=CARTESIAN_POINT('Ctrl Pts',(16.0139309877157,72.3839562882486,11.9339956234801));
#56744=CARTESIAN_POINT('Ctrl Pts',(16.018524854418,72.4399222667451,11.9609057195569));
#56745=CARTESIAN_POINT('Ctrl Pts',(16.0231187211203,72.4943790953525,11.9908609217262));
#56746=CARTESIAN_POINT('Ctrl Pts',(16.0277125878226,72.5469875513231,12.0236547013596));
#56747=CARTESIAN_POINT('Ctrl Pts',(16.0323592224054,72.6002002992542,12.0568251698165));
#56748=CARTESIAN_POINT('Ctrl Pts',(16.0370058569881,72.6515214953787,12.0928995509853));
#56749=CARTESIAN_POINT('Ctrl Pts',(16.0416524915709,72.7006328641361,12.1316209662255));
#56750=CARTESIAN_POINT('Ctrl Pts',(16.0462991261536,72.7497442328934,12.1703423814656));
#56751=CARTESIAN_POINT('Ctrl Pts',(16.0509457607364,72.7966454179646,12.2117104332495));
#56752=CARTESIAN_POINT('Ctrl Pts',(16.0555923953191,72.8410568939521,12.255430352946));
#56753=CARTESIAN_POINT('Ctrl Pts',(16.060196557806,72.885062431312,12.2987506551157));
#56754=CARTESIAN_POINT('Ctrl Pts',(16.064800720293,72.9267975936672,12.344551233288));
#56755=CARTESIAN_POINT('Ctrl Pts',(16.0694048827799,72.9659712349874,12.3925648748423));
#56756=CARTESIAN_POINT('Ctrl Pts',(16.0740170889281,73.0052133142713,12.4406623982043));
#56757=CARTESIAN_POINT('Ctrl Pts',(16.0786292950764,73.041884516254,12.4909803995974));
#56758=CARTESIAN_POINT('Ctrl Pts',(16.0832415012246,73.0757282696727,12.5432120649388));
#56759=CARTESIAN_POINT('Ctrl Pts',(16.0878334122674,73.109423100315,12.5952138951162));
#56760=CARTESIAN_POINT('Ctrl Pts',(16.0924253233102,73.1403150134699,12.6491121710601));
#56761=CARTESIAN_POINT('Ctrl Pts',(16.097017234353,73.1681917198803,12.7045718757035));
#56762=CARTESIAN_POINT('Ctrl Pts',(16.1016064324736,73.1960519566043,12.7599988144984));
#56763=CARTESIAN_POINT('Ctrl Pts',(16.1061956305943,73.2209002921553,12.8169849001973));
#56764=CARTESIAN_POINT('Ctrl Pts',(16.1107848287149,73.2425699523366,12.8751697898112));
#56765=CARTESIAN_POINT('Ctrl Pts',(16.1153729858509,73.264234697109,12.9333414811325));
#56766=CARTESIAN_POINT('Ctrl Pts',(16.1199611429868,73.282722021386,12.9927109612972));
#56767=CARTESIAN_POINT('Ctrl Pts',(16.1245493001227,73.2979137286391,13.05289903829));
#56768=CARTESIAN_POINT('Ctrl Pts',(16.1291783443073,73.3132408157528,13.1136234772163));
#56769=CARTESIAN_POINT('Ctrl Pts',(16.1338073884919,73.325213094183,13.1751806757362));
#56770=CARTESIAN_POINT('Ctrl Pts',(16.1384364326765,73.3337615042061,13.2371690168494));
#56771=CARTESIAN_POINT('Ctrl Pts',(16.1430303005577,73.3422449544982,13.2986863059242));
#56772=CARTESIAN_POINT('Ctrl Pts',(16.1476241684388,73.3473564086421,13.3606276905436));
#56773=CARTESIAN_POINT('Ctrl Pts',(16.1522180363199,73.3490806409208,13.4225963149988));
#56774=CARTESIAN_POINT('Ctrl Pts',(16.1568646686562,73.3508246774645,13.4852767014799));
#56775=CARTESIAN_POINT('Ctrl Pts',(16.1615113009926,73.3491031829668,13.5479844251041));
#56776=CARTESIAN_POINT('Ctrl Pts',(16.1661579333289,73.343954473631,13.6103122792496));
#56777=CARTESIAN_POINT('Ctrl Pts',(16.1708045656652,73.3388057642951,13.6726401333951));
#56778=CARTESIAN_POINT('Ctrl Pts',(16.1754511980016,73.3302299746642,13.7345876014508));
#56779=CARTESIAN_POINT('Ctrl Pts',(16.1800978303379,73.3183184105988,13.7957588480447));
#56780=CARTESIAN_POINT('Ctrl Pts',(16.1847019924617,73.3065157182112,13.8563709895367));
#56781=CARTESIAN_POINT('Ctrl Pts',(16.1893061545855,73.2913913686667,13.9164606737471));
#56782=CARTESIAN_POINT('Ctrl Pts',(16.1939103167092,73.2730072786163,13.9756375996653));
#56783=CARTESIAN_POINT('Ctrl Pts',(16.1985225229029,73.2545910691702,14.0349179153672));
#56784=CARTESIAN_POINT('Ctrl Pts',(16.2031347290965,73.2329037695676,14.0932817691944));
#56785=CARTESIAN_POINT('Ctrl Pts',(16.2077469352901,73.2080594064967,14.1503458053722));
#56786=CARTESIAN_POINT('Ctrl Pts',(16.2123388459611,73.1833243684022,14.2071587373299));
#56787=CARTESIAN_POINT('Ctrl Pts',(16.2169307566321,73.1554601710129,14.26268278935));
#56788=CARTESIAN_POINT('Ctrl Pts',(16.2215226673031,73.1246288116329,14.3165559393419));
#56789=CARTESIAN_POINT('Ctrl Pts',(16.2261118650498,73.0938156675777,14.3703972608012));
#56790=CARTESIAN_POINT('Ctrl Pts',(16.2307010627965,73.0600390895782,14.422589175253));
#56791=CARTESIAN_POINT('Ctrl Pts',(16.2352902605432,73.0235073284427,14.4727936113141));
#56792=CARTESIAN_POINT('Ctrl Pts',(16.2398784173036,72.9869838539538,14.5229866593007));
#56793=CARTESIAN_POINT('Ctrl Pts',(16.2444665740641,72.9477067356623,14.5711927142205));
#56794=CARTESIAN_POINT('Ctrl Pts',(16.2490547308245,72.9059267706146,14.6171037861344));
#56795=CARTESIAN_POINT('Ctrl Pts',(16.2536837753689,72.8637744795392,14.6634239988175));
#56796=CARTESIAN_POINT('Ctrl Pts',(16.2583128199132,72.8190748379485,14.7074077100018));
#56797=CARTESIAN_POINT('Ctrl Pts',(16.2629418644576,72.7721244789935,14.7487755018129));
#56798=CARTESIAN_POINT('Ctrl Pts',(16.2675357319639,72.725530905234,14.7898289314761));
#56799=CARTESIAN_POINT('Ctrl Pts',(16.2721295994702,72.6767211430397,14.8283057896959));
#56800=CARTESIAN_POINT('Ctrl Pts',(16.2767234669765,72.6260175940621,14.86397416397));
#56801=CARTESIAN_POINT('Ctrl Pts',(16.2813701000399,72.5747316597627,14.9000522282568));
#56802=CARTESIAN_POINT('Ctrl Pts',(16.2860167331032,72.5215085991454,14.9332565837703));
#56803=CARTESIAN_POINT('Ctrl Pts',(16.2906633661666,72.4667090186912,14.9633942317474));
#56804=CARTESIAN_POINT('Ctrl Pts',(16.2953099992299,72.411909438237,14.9935318797246));
#56805=CARTESIAN_POINT('Ctrl Pts',(16.2999566322933,72.3555338429059,15.0206026469455));
#56806=CARTESIAN_POINT('Ctrl Pts',(16.3046032653567,72.2979626314675,15.0444639873977));
#56807=CARTESIAN_POINT('Ctrl Pts',(16.3097079245347,72.2347165328731,15.0706773786592));
#56808=CARTESIAN_POINT('Ctrl Pts',(16.3148125837127,72.169816198335,15.0931062139384));
#56809=CARTESIAN_POINT('Ctrl Pts',(16.3199172428907,72.1037055186798,15.1115635495306));
#56810=CARTESIAN_POINT('Ctrl Pts',(16.3250050814713,72.037812683368,15.1299600655068));
#56811=CARTESIAN_POINT('Ctrl Pts',(16.3300929200518,71.9707177406488,15.1444110519676));
#56812=CARTESIAN_POINT('Ctrl Pts',(16.3351807586324,71.9028819957496,15.1547782813963));
#56813=CARTESIAN_POINT('Ctrl Pts',(16.3402418161921,71.8354033200608,15.1650909405033));
#56814=CARTESIAN_POINT('Ctrl Pts',(16.3453028737517,71.7671919133591,15.1713625929221));
#56815=CARTESIAN_POINT('Ctrl Pts',(16.3503639313113,71.6987191891739,15.1735057674296));
#56816=CARTESIAN_POINT('Ctrl Pts',(16.3516559260016,71.6812393650395,15.1740528803702));
#56817=CARTESIAN_POINT('Ctrl Pts',(16.3529479206919,71.663742587001,15.1743311990977));
#56818=CARTESIAN_POINT('Ctrl Pts',(16.3542399153822,71.6462368438885,15.1743397945516));
#56819=CARTESIAN_POINT('',(17.1479899153848,71.6439440199028,15.174339378094));
#56820=CARTESIAN_POINT('Ctrl Pts',(16.3542399154298,71.6462368432431,15.174339794552));
#56821=CARTESIAN_POINT('Ctrl Pts',(16.3588871624829,71.5832694690705,15.1743707119909));
#56822=CARTESIAN_POINT('Ctrl Pts',(16.363534409536,71.5203035798291,15.1709077637263));
#56823=CARTESIAN_POINT('Ctrl Pts',(16.3681816565891,71.4577458076997,15.163977786074));
#56824=CARTESIAN_POINT('Ctrl Pts',(16.3728305705312,71.3951655971534,15.1570453227556));
#56825=CARTESIAN_POINT('Ctrl Pts',(16.3774794844734,71.3329942797243,15.1466434159465));
#56826=CARTESIAN_POINT('Ctrl Pts',(16.3821283984155,71.2716314321484,15.1328505324551));
#56827=CARTESIAN_POINT('Ctrl Pts',(16.3867839971765,71.2101803490142,15.119037815745));
#56828=CARTESIAN_POINT('Ctrl Pts',(16.3914395959375,71.1495405328699,15.1018245005813));
#56829=CARTESIAN_POINT('Ctrl Pts',(16.3960951946984,71.0900985982484,15.0813395634728));
#56830=CARTESIAN_POINT('Ctrl Pts',(16.4007546246755,71.030607747277,15.0608377687644));
#56831=CARTESIAN_POINT('Ctrl Pts',(16.4054140546525,70.9723171923226,15.0370591771749));
#56832=CARTESIAN_POINT('Ctrl Pts',(16.4100734846296,70.9155929391788,15.0101806678359));
#56833=CARTESIAN_POINT('Ctrl Pts',(16.4147419584392,70.8587585857334,14.9832499880086));
#56834=CARTESIAN_POINT('Ctrl Pts',(16.4194104322488,70.803497031157,14.9532076138302));
#56835=CARTESIAN_POINT('Ctrl Pts',(16.4240789060584,70.7501483512317,14.9202756017315));
#56836=CARTESIAN_POINT('Ctrl Pts',(16.4257555041641,70.730989135747,14.9084486639885));
#56837=CARTESIAN_POINT('Ctrl Pts',(16.4274321022698,70.7120763427755,14.8962494254406));
#56838=CARTESIAN_POINT('Ctrl Pts',(16.4291087003754,70.69342469322,14.8836894464065));
#56839=CARTESIAN_POINT('Ctrl Pts',(16.4337128625557,70.642204774032,14.8491980675494));
#56840=CARTESIAN_POINT('Ctrl Pts',(16.4383170247359,70.5927605262358,14.8118512798714));
#56841=CARTESIAN_POINT('Ctrl Pts',(16.4429211869162,70.5454272604206,14.7718582133943));
#56842=CARTESIAN_POINT('Ctrl Pts',(16.4475333931028,70.49801129789,14.731795274383));
#56843=CARTESIAN_POINT('Ctrl Pts',(16.4521455992894,70.452714151242,14.6890770477523));
#56844=CARTESIAN_POINT('Ctrl Pts',(16.456757805476,70.4098444265217,14.6439579466262));
#56845=CARTESIAN_POINT('Ctrl Pts',(16.4613497162028,70.3671633448792,14.5990373866887));
#56846=CARTESIAN_POINT('Ctrl Pts',(16.4659416269297,70.3268887374615,14.5517373873812));
#56847=CARTESIAN_POINT('Ctrl Pts',(16.4705335376566,70.2892908682312,14.5023482253257));
#56848=CARTESIAN_POINT('Ctrl Pts',(16.4751227354588,70.2517152120173,14.4529882426438));
#56849=CARTESIAN_POINT('Ctrl Pts',(16.479711933261,70.2168134642751,14.4015419478507));
#56850=CARTESIAN_POINT('Ctrl Pts',(16.4843011310632,70.1848158059665,14.3483328798009));
#56851=CARTESIAN_POINT('Ctrl Pts',(16.4888892878786,70.152825405819,14.2951358813841));
#56852=CARTESIAN_POINT('Ctrl Pts',(16.4934774446941,70.1237380482417,14.2401773381916));
#56853=CARTESIAN_POINT('Ctrl Pts',(16.4980656015095,70.0977396300053,14.1838082478845));
#56854=CARTESIAN_POINT('Ctrl Pts',(16.5026946459999,70.0715095250773,14.1269368205534));
#56855=CARTESIAN_POINT('Ctrl Pts',(16.5073236904903,70.0484239391731,14.0686300418957));
#56856=CARTESIAN_POINT('Ctrl Pts',(16.5119527349807,70.0286245927657,14.0092699863355));
#56857=CARTESIAN_POINT('Ctrl Pts',(16.5165466025402,70.0089757051069,13.9503610183765));
#56858=CARTESIAN_POINT('Ctrl Pts',(16.5211404700996,69.9925633636205,13.8904152375184));
#56859=CARTESIAN_POINT('Ctrl Pts',(16.5257343376591,69.9794754969945,13.8298199353646));
#56860=CARTESIAN_POINT('Ctrl Pts',(16.530380970615,69.9662373024668,13.7685286324888));
#56861=CARTESIAN_POINT('Ctrl Pts',(16.5350276035708,69.9564005406046,13.7065733151398));
#56862=CARTESIAN_POINT('Ctrl Pts',(16.5396742365267,69.9500024138971,13.6443612934011));
#56863=CARTESIAN_POINT('Ctrl Pts',(16.5443208694825,69.9436042871896,13.5821492716623));
#56864=CARTESIAN_POINT('Ctrl Pts',(16.5489675024384,69.9406447583667,13.5196810780754));
#56865=CARTESIAN_POINT('Ctrl Pts',(16.5536141353942,69.9411068528548,13.457362587531));
#56866=CARTESIAN_POINT('Ctrl Pts',(16.5582182975238,69.9415647237395,13.3956136960519));
#56867=CARTESIAN_POINT('Ctrl Pts',(16.5628224596533,69.9453836854699,13.3337676644005));
#56868=CARTESIAN_POINT('Ctrl Pts',(16.5674266217829,69.9525746342542,13.2722195239975));
#56869=CARTESIAN_POINT('Ctrl Pts',(16.5720388279758,69.959778146551,13.2105638510776));
#56870=CARTESIAN_POINT('Ctrl Pts',(16.5766510341687,69.9703654829862,13.1492076232064));
#56871=CARTESIAN_POINT('Ctrl Pts',(16.5812632403617,69.9842950411052,13.0885486254645));
#56872=CARTESIAN_POINT('Ctrl Pts',(16.5858551510364,69.998163303699,13.0281565511301));
#56873=CARTESIAN_POINT('Ctrl Pts',(16.5904470617111,70.0153443485486,12.9684560858829));
#56874=CARTESIAN_POINT('Ctrl Pts',(16.5950389723858,70.0357454980589,12.9098328642444));
#56875=CARTESIAN_POINT('Ctrl Pts',(16.5996281701355,70.0561345944622,12.8512442775151));
#56876=CARTESIAN_POINT('Ctrl Pts',(16.6042173678851,70.0797398561651,12.7937321502646));
#56877=CARTESIAN_POINT('Ctrl Pts',(16.6088065656347,70.1064187371306,12.7376670783469));
#56878=CARTESIAN_POINT('Ctrl Pts',(16.6133947223973,70.1330915664134,12.6816147239051));
#56879=CARTESIAN_POINT('Ctrl Pts',(16.6179828791599,70.1628364126363,12.6270092307533));
#56880=CARTESIAN_POINT('Ctrl Pts',(16.6225710359226,70.195463378247,12.574199448259));
#56881=CARTESIAN_POINT('Ctrl Pts',(16.6272000804634,70.2283811020432,12.5209190465623));
#56882=CARTESIAN_POINT('Ctrl Pts',(16.6318291250043,70.2642323236069,12.4694669842057));
#56883=CARTESIAN_POINT('Ctrl Pts',(16.6364581695452,70.3027768375861,12.4201724525668));
#56884=CARTESIAN_POINT('Ctrl Pts',(16.6410520370517,70.3410284441021,12.371252519923));
#56885=CARTESIAN_POINT('Ctrl Pts',(16.6456459045582,70.3819321685111,12.3244577889898));
#56886=CARTESIAN_POINT('Ctrl Pts',(16.6502397720647,70.4252137422743,12.2800754931268));
#56887=CARTESIAN_POINT('Ctrl Pts',(16.6548864051227,70.4689924518623,12.2351834184518));
#56888=CARTESIAN_POINT('Ctrl Pts',(16.6595330381808,70.5152036032517,12.1927599238098));
#56889=CARTESIAN_POINT('Ctrl Pts',(16.6641796712388,70.5635282199637,12.1530610161586));
#56890=CARTESIAN_POINT('Ctrl Pts',(16.6688263042969,70.6118528366758,12.1133621085074));
#56891=CARTESIAN_POINT('Ctrl Pts',(16.673472937355,70.6622904542047,12.0763880509518));
#56892=CARTESIAN_POINT('Ctrl Pts',(16.678119570413,70.7144933653474,12.0423488965578));
#56893=CARTESIAN_POINT('Ctrl Pts',(16.6827237325413,70.7662191339778,12.008620865189));
#56894=CARTESIAN_POINT('Ctrl Pts',(16.6873278946696,70.8198825227819,11.9776409233246));
#56895=CARTESIAN_POINT('Ctrl Pts',(16.691932056798,70.8751602591703,11.9496363667706));
#56896=CARTESIAN_POINT('Ctrl Pts',(16.696544262991,70.9305345728899,11.9215828826463));
#56897=CARTESIAN_POINT('Ctrl Pts',(16.7011564691841,70.9875284777049,11.8965155093395));
#56898=CARTESIAN_POINT('Ctrl Pts',(16.7057686753772,71.0457874056845,11.8746193017533));
#56899=CARTESIAN_POINT('Ctrl Pts',(16.7103605860502,71.1037899714826,11.8528194460866));
#56900=CARTESIAN_POINT('Ctrl Pts',(16.7149524967232,71.1630459838935,11.8341631108941));
#56901=CARTESIAN_POINT('Ctrl Pts',(16.7195444073963,71.2231827898986,11.8187860638021));
#56902=CARTESIAN_POINT('Ctrl Pts',(16.724133605144,71.2832840667586,11.8034181015514));
#56903=CARTESIAN_POINT('Ctrl Pts',(16.7287228028918,71.3442646147717,11.7913257104668));
#56904=CARTESIAN_POINT('Ctrl Pts',(16.7333120006395,71.4057367698828,11.7825947814085));
#56905=CARTESIAN_POINT('Ctrl Pts',(16.7379001574001,71.4671949810043,11.7738658328238));
#56906=CARTESIAN_POINT('Ctrl Pts',(16.7424883141607,71.5291440758616,11.7684969034079));
#56907=CARTESIAN_POINT('Ctrl Pts',(16.7470764709212,71.5911883612235,11.766522399965));
#56908=CARTESIAN_POINT('Ctrl Pts',(16.7517055154638,71.6537855599544,11.7645303005526));
#56909=CARTESIAN_POINT('Ctrl Pts',(16.7563345600063,71.7164791315643,11.7659934791591));
#56910=CARTESIAN_POINT('Ctrl Pts',(16.7609636045489,71.7788619796757,11.7708935478961));
#56911=CARTESIAN_POINT('Ctrl Pts',(16.7655574720529,71.8407707680047,11.7757563800274));
#56912=CARTESIAN_POINT('Ctrl Pts',(16.770151339557,71.9023730372047,11.7840039215462));
#56913=CARTESIAN_POINT('Ctrl Pts',(16.774745207061,71.9632778501082,11.7955662127123));
#56914=CARTESIAN_POINT('Ctrl Pts',(16.7793918401228,72.0248822209372,11.8072613093504));
#56915=CARTESIAN_POINT('Ctrl Pts',(16.7840384731846,72.085772490495,11.8223476771256));
#56916=CARTESIAN_POINT('Ctrl Pts',(16.7886851062464,72.1455590550303,11.8407008392345));
#56917=CARTESIAN_POINT('Ctrl Pts',(16.7933317393082,72.2053456195656,11.8590540013434));
#56918=CARTESIAN_POINT('Ctrl Pts',(16.7979783723699,72.2640280031684,11.8806737159195));
#56919=CARTESIAN_POINT('Ctrl Pts',(16.8026250054317,72.3212390378092,11.9053861720626));
#56920=CARTESIAN_POINT('Ctrl Pts',(16.8072291675718,72.37792715503,11.9298727526575));
#56921=CARTESIAN_POINT('Ctrl Pts',(16.8118333297119,72.4333948401411,11.9574925286597));
#56922=CARTESIAN_POINT('Ctrl Pts',(16.816437491852,72.487274049383,11.9881015822347));
#56923=CARTESIAN_POINT('Ctrl Pts',(16.8210496980436,72.5412473923939,12.0187641136839));
#56924=CARTESIAN_POINT('Ctrl Pts',(16.8256619042352,72.5936262154243,12.0524262182956));
#56925=CARTESIAN_POINT('Ctrl Pts',(16.8302741104268,72.6440603986762,12.0888945573505));
#56926=CARTESIAN_POINT('Ctrl Pts',(16.8348660211122,72.6942726518502,12.1252024214895));
#56927=CARTESIAN_POINT('Ctrl Pts',(16.8394579317976,72.7425569150337,12.1642915990056));
#56928=CARTESIAN_POINT('Ctrl Pts',(16.844049842483,72.7885941633852,12.2059264497657));
#56929=CARTESIAN_POINT('Ctrl Pts',(16.8486390402434,72.8346042126872,12.247536702436));
#56930=CARTESIAN_POINT('Ctrl Pts',(16.8532282380037,72.8783695045443,12.2916893060575));
#56931=CARTESIAN_POINT('Ctrl Pts',(16.857817435764,72.91960429855,12.338108555931));
#56932=CARTESIAN_POINT('Ctrl Pts',(16.8624055925373,72.9608297390943,12.3845172763311));
#56933=CARTESIAN_POINT('Ctrl Pts',(16.8669937493107,72.999525484948,12.4331912429753));
#56934=CARTESIAN_POINT('Ctrl Pts',(16.871581906084,73.0354442766861,12.4838196187045));
#56935=CARTESIAN_POINT('Ctrl Pts',(16.8762109506146,73.0716831618535,12.5348991735971));
#56936=CARTESIAN_POINT('Ctrl Pts',(16.8808399951451,73.1050950208235,12.5879677374539));
#56937=CARTESIAN_POINT('Ctrl Pts',(16.8854690396756,73.1354703039202,12.6426758041884));
#56938=CARTESIAN_POINT('Ctrl Pts',(16.8900629071927,73.1656147593083,12.6969681336393));
#56939=CARTESIAN_POINT('Ctrl Pts',(16.8946567747098,73.1927684582529,12.7528746463588));
#56940=CARTESIAN_POINT('Ctrl Pts',(16.8992506422269,73.2167737667556,12.8100308183313));
#56941=CARTESIAN_POINT('Ctrl Pts',(16.9038972752642,73.2410548021018,12.8678434905477));
#56942=CARTESIAN_POINT('Ctrl Pts',(16.9085439083015,73.2621144654426,12.9269342170202));
#56943=CARTESIAN_POINT('Ctrl Pts',(16.9131905413387,73.2798413038651,12.9869094703685));
#56944=CARTESIAN_POINT('Ctrl Pts',(16.917837174376,73.2975681422877,13.0468847237168));
#56945=CARTESIAN_POINT('Ctrl Pts',(16.9224838074133,73.3119620945183,13.1077439736246));
#56946=CARTESIAN_POINT('Ctrl Pts',(16.9271304404505,73.3229652250746,13.169085142905));
#56947=CARTESIAN_POINT('Ctrl Pts',(16.9317346025836,73.3338677854115,13.2298656449451));
#56948=CARTESIAN_POINT('Ctrl Pts',(16.9363387647168,73.3414844073172,13.2913595729054));
#56949=CARTESIAN_POINT('Ctrl Pts',(16.9409429268499,73.3457317532,13.3531806323423));
#56950=CARTESIAN_POINT('Ctrl Pts',(16.9455551330423,73.3499865197386,13.4151097010669));
#56951=CARTESIAN_POINT('Ctrl Pts',(16.9501673392348,73.3508600892818,13.4773665502191));
#56952=CARTESIAN_POINT('Ctrl Pts',(16.9547795454273,73.3483202217464,13.5395525266776));
#56953=CARTESIAN_POINT('Ctrl Pts',(16.9593714561055,73.3457915306232,13.6014648604752));
#56954=CARTESIAN_POINT('Ctrl Pts',(16.9639633667837,73.3398793734571,13.6633064343219));
#56955=CARTESIAN_POINT('Ctrl Pts',(16.9685552774618,73.330603948578,13.7246811482951));
#56956=CARTESIAN_POINT('Ctrl Pts',(16.9731444752149,73.3213340036691,13.7860196017623));
#56957=CARTESIAN_POINT('Ctrl Pts',(16.9777336729679,73.3087048074216,13.8468912418622));
#56958=CARTESIAN_POINT('Ctrl Pts',(16.9823228707209,73.2927883414332,13.9069055826033));
#56959=CARTESIAN_POINT('Ctrl Pts',(16.9869110274869,73.2768754858439,13.9669063100386));
#56960=CARTESIAN_POINT('Ctrl Pts',(16.9914991842528,73.2576769711982,14.0260496342609));
#56961=CARTESIAN_POINT('Ctrl Pts',(16.9960873410188,73.2353153215806,14.0839577394278));
#56962=CARTESIAN_POINT('Ctrl Pts',(17.0007163855563,73.2127543941117,14.1423818978809));
#56963=CARTESIAN_POINT('Ctrl Pts',(17.0053454300939,73.1869738302626,14.1995482107794));
#56964=CARTESIAN_POINT('Ctrl Pts',(17.0099744746314,73.1581492185228,14.2550889360185));
#56965=CARTESIAN_POINT('Ctrl Pts',(17.0145683421411,73.1295436507266,14.3102075962668));
#56966=CARTESIAN_POINT('Ctrl Pts',(17.0191622096507,73.0979404514304,14.3637248767813));
#56967=CARTESIAN_POINT('Ctrl Pts',(17.0237560771604,73.0635564057154,14.4153080156903));
#56968=CARTESIAN_POINT('Ctrl Pts',(17.0284027102119,73.02877742201,14.4674836427953));
#56969=CARTESIAN_POINT('Ctrl Pts',(17.0330493432634,72.991153607696,14.517679977289));
#56970=CARTESIAN_POINT('Ctrl Pts',(17.0376959763149,72.9509514347238,14.5655867317975));
#56971=CARTESIAN_POINT('Ctrl Pts',(17.0423426093664,72.9107492617515,14.6134934863059));
#56972=CARTESIAN_POINT('Ctrl Pts',(17.0469892424178,72.8679691383366,14.6591103168089));
#56973=CARTESIAN_POINT('Ctrl Pts',(17.0516358754693,72.8229142261024,14.7021668243085));
#56974=CARTESIAN_POINT('Ctrl Pts',(17.0561790386785,72.7788625832488,14.7442645623095));
#56975=CARTESIAN_POINT('Ctrl Pts',(17.0607222018877,72.7324519488316,14.7840909041797));
#56976=CARTESIAN_POINT('Ctrl Pts',(17.0652653650969,72.6839488770977,14.8213663698195));
#56977=CARTESIAN_POINT('Ctrl Pts',(17.0698023105883,72.6355121860765,14.8585908207115));
#56978=CARTESIAN_POINT('Ctrl Pts',(17.0743392560797,72.5849891390917,14.8932709945406));
#56979=CARTESIAN_POINT('Ctrl Pts',(17.0788762015711,72.5326822271473,14.9251649683072));
#56980=CARTESIAN_POINT('Ctrl Pts',(17.0834086977726,72.4804266115247,14.9570276643041));
#56981=CARTESIAN_POINT('Ctrl Pts',(17.087941193974,72.4263910408378,14.9861093042422));
#56982=CARTESIAN_POINT('Ctrl Pts',(17.0924736901755,72.3709083198828,15.0122102688612));
#56983=CARTESIAN_POINT('Ctrl Pts',(17.0971000422763,72.3142766998578,15.0388517147951));
#56984=CARTESIAN_POINT('Ctrl Pts',(17.1017263943771,72.2561377765807,15.0623873233133));
#56985=CARTESIAN_POINT('Ctrl Pts',(17.1063527464778,72.1968719525397,15.0826541852369));
#56986=CARTESIAN_POINT('Ctrl Pts',(17.1108831137178,72.1388357413225,15.1025005621049));
#56987=CARTESIAN_POINT('Ctrl Pts',(17.1154134809578,72.0797194742587,15.1192124147451));
#56988=CARTESIAN_POINT('Ctrl Pts',(17.1199438481978,72.0198979852371,15.132686408994));
#56989=CARTESIAN_POINT('Ctrl Pts',(17.1246181927289,71.9581753399763,15.1465886133836));
#56990=CARTESIAN_POINT('Ctrl Pts',(17.1292925372601,71.8957024531013,15.1570434910494));
#56991=CARTESIAN_POINT('Ctrl Pts',(17.1339668817913,71.832901938976,15.1639946453517));
#56992=CARTESIAN_POINT('Ctrl Pts',(17.1386412263225,71.7701014248507,15.170945799654));
#56993=CARTESIAN_POINT('Ctrl Pts',(17.1433155708536,71.7069738919126,15.1743932231441));
#56994=CARTESIAN_POINT('Ctrl Pts',(17.1479899153848,71.6439440199028,15.174339378094));
#56995=CARTESIAN_POINT('',(17.9417399154741,71.6466202076947,15.1743395632013));
#56996=CARTESIAN_POINT('Ctrl Pts',(17.1479899154299,71.6439440192947,15.1743393780935));
#56997=CARTESIAN_POINT('Ctrl Pts',(17.154145561567,71.5609399562498,15.1742684694964));
#56998=CARTESIAN_POINT('Ctrl Pts',(17.1603012077041,71.4781926934508,15.1681301741125));
#56999=CARTESIAN_POINT('Ctrl Pts',(17.1664568538413,71.3964381367899,15.1560583697687));
#57000=CARTESIAN_POINT('Ctrl Pts',(17.1696850060568,71.3535643023719,15.1497276579196));
#57001=CARTESIAN_POINT('Ctrl Pts',(17.1729131582724,71.3109630137133,15.1417659085998));
#57002=CARTESIAN_POINT('Ctrl Pts',(17.176141310488,71.2687378943283,15.132197489395));
#57003=CARTESIAN_POINT('Ctrl Pts',(17.1807454726154,71.2085141866116,15.1185505017749));
#57004=CARTESIAN_POINT('Ctrl Pts',(17.1853496347428,71.1489140648698,15.1015993488436));
#57005=CARTESIAN_POINT('Ctrl Pts',(17.1899537968702,71.0903257587081,15.0814178298177));
#57006=CARTESIAN_POINT('Ctrl Pts',(17.1945660030634,71.0316350912098,15.0612010510718));
#57007=CARTESIAN_POINT('Ctrl Pts',(17.1991782092565,70.9739602875218,15.0377426749009));
#57008=CARTESIAN_POINT('Ctrl Pts',(17.2037904154497,70.9176810449265,15.0111683743273));
#57009=CARTESIAN_POINT('Ctrl Pts',(17.2083823261224,70.8616494531249,14.9847110111241));
#57010=CARTESIAN_POINT('Ctrl Pts',(17.212974236795,70.8070016382065,14.9551652808883));
#57011=CARTESIAN_POINT('Ctrl Pts',(17.2175661474677,70.7540945097158,14.9227041538418));
#57012=CARTESIAN_POINT('Ctrl Pts',(17.2221553452153,70.7012186390359,14.8902622050005));
#57013=CARTESIAN_POINT('Ctrl Pts',(17.2267445429629,70.6500818466847,14.8549085400333));
#57014=CARTESIAN_POINT('Ctrl Pts',(17.2313337407104,70.6010156910675,14.8168616301817));
#57015=CARTESIAN_POINT('Ctrl Pts',(17.2359218974711,70.5519606653323,14.7788233506702));
#57016=CARTESIAN_POINT('Ctrl Pts',(17.2405100542317,70.5049757442545,14.7380933500799));
#57017=CARTESIAN_POINT('Ctrl Pts',(17.2450982109923,70.4603611203596,14.6949317080314));
#57018=CARTESIAN_POINT('Ctrl Pts',(17.2497272555352,70.4153489091278,14.6513854270277));
#57019=CARTESIAN_POINT('Ctrl Pts',(17.2543563000781,70.3727498524199,14.6053642886211));
#57020=CARTESIAN_POINT('Ctrl Pts',(17.2589853446209,70.3328341851558,14.5571733152089));
#57021=CARTESIAN_POINT('Ctrl Pts',(17.2635792121255,70.2932218450562,14.5093485546732));
#57022=CARTESIAN_POINT('Ctrl Pts',(17.2681730796301,70.2562525110266,14.4593872711379));
#57023=CARTESIAN_POINT('Ctrl Pts',(17.2727669471347,70.2221481483269,14.4076187937051));
#57024=CARTESIAN_POINT('Ctrl Pts',(17.2774135801968,70.1876520599828,14.3552556990863));
#57025=CARTESIAN_POINT('Ctrl Pts',(17.2820602132588,70.1560874600736,14.3010440817876));
#57026=CARTESIAN_POINT('Ctrl Pts',(17.2867068463208,70.1276362522913,14.245350270356));
#57027=CARTESIAN_POINT('Ctrl Pts',(17.2913534793828,70.0991850445089,14.1896564589244));
#57028=CARTESIAN_POINT('Ctrl Pts',(17.2960001124449,70.0738473865819,14.1324809633711));
#57029=CARTESIAN_POINT('Ctrl Pts',(17.3006467455069,70.0517541489216,14.07420835557));
#57030=CARTESIAN_POINT('Ctrl Pts',(17.305250907637,70.0298628468088,14.0164683682541));
#57031=CARTESIAN_POINT('Ctrl Pts',(17.3098550697672,70.0110703066881,13.957422991343));
#57032=CARTESIAN_POINT('Ctrl Pts',(17.3144592318973,69.9955294663945,13.8974366127747));
#57033=CARTESIAN_POINT('Ctrl Pts',(17.3190714380902,69.9799614742565,13.8373454302971));
#57034=CARTESIAN_POINT('Ctrl Pts',(17.323683644283,69.9676567804078,13.7763104165833));
#57035=CARTESIAN_POINT('Ctrl Pts',(17.3282958504759,69.9587203683434,13.7147175019381));
#57036=CARTESIAN_POINT('Ctrl Pts',(17.3328877611508,69.9498232800003,13.653395620297));
#57037=CARTESIAN_POINT('Ctrl Pts',(17.3374796718258,69.9442649925582,13.5915212371243));
#57038=CARTESIAN_POINT('Ctrl Pts',(17.3420715825008,69.9420984755528,13.5294874139279));
#57039=CARTESIAN_POINT('Ctrl Pts',(17.3466607802506,69.9399332385372,13.4674902406439));
#57040=CARTESIAN_POINT('Ctrl Pts',(17.3512499780003,69.9411558154965,13.4053343200391));
#57041=CARTESIAN_POINT('Ctrl Pts',(17.35583917575,69.9457672432653,13.3434167158172));
#57042=CARTESIAN_POINT('Ctrl Pts',(17.3604273325126,69.9503776250044,13.2815131566273));
#57043=CARTESIAN_POINT('Ctrl Pts',(17.3650154892753,69.9583752934179,13.2198483120309));
#57044=CARTESIAN_POINT('Ctrl Pts',(17.3696036460379,69.969709274973,13.1588160838692));
#57045=CARTESIAN_POINT('Ctrl Pts',(17.3742326905785,69.9811442603399,13.0972399614319));
#57046=CARTESIAN_POINT('Ctrl Pts',(17.3788617351191,69.9959752570609,13.036308308371));
#57047=CARTESIAN_POINT('Ctrl Pts',(17.3834907796598,70.0140972796604,12.976414880479));
#57048=CARTESIAN_POINT('Ctrl Pts',(17.388084647166,70.0320815893888,12.916976594714));
#57049=CARTESIAN_POINT('Ctrl Pts',(17.3926785146721,70.0533068491446,12.8585612725601));
#57050=CARTESIAN_POINT('Ctrl Pts',(17.3972723821783,70.0776211479283,12.8015358599022));
#57051=CARTESIAN_POINT('Ctrl Pts',(17.4019190152362,70.1022147228096,12.7438554485189));
#57052=CARTESIAN_POINT('Ctrl Pts',(17.4065656482941,70.1299685313298,12.6875975644117));
#57053=CARTESIAN_POINT('Ctrl Pts',(17.411212281352,70.1606776906095,12.633116197075));
#57054=CARTESIAN_POINT('Ctrl Pts',(17.4158589144098,70.1913868498893,12.5786348297384));
#57055=CARTESIAN_POINT('Ctrl Pts',(17.4205055474677,70.2250510219201,12.5259303923793));
#57056=CARTESIAN_POINT('Ctrl Pts',(17.4251521805256,70.2614219260227,12.4753244115039));
#57057=CARTESIAN_POINT('Ctrl Pts',(17.4297563427082,70.2974603949805,12.4251809763637));
#57058=CARTESIAN_POINT('Ctrl Pts',(17.4343605048907,70.3362987518513,12.3768995283544));
#57059=CARTESIAN_POINT('Ctrl Pts',(17.4389646670733,70.3777177308449,12.3308088395402));
#57060=CARTESIAN_POINT('Ctrl Pts',(17.4435768732596,70.4192090735843,12.2846376249629));
#57061=CARTESIAN_POINT('Ctrl Pts',(17.4481890794459,70.4632898039885,12.2406652747666));
#57062=CARTESIAN_POINT('Ctrl Pts',(17.4528012856322,70.5096962092413,12.1991924869374));
#57063=CARTESIAN_POINT('Ctrl Pts',(17.45739319636,70.5558984086906,12.1579021951217));
#57064=CARTESIAN_POINT('Ctrl Pts',(17.4619851070879,70.6044054971416,12.1190898735605));
#57065=CARTESIAN_POINT('Ctrl Pts',(17.4665770178157,70.6549190851283,12.0830168015167));
#57066=CARTESIAN_POINT('Ctrl Pts',(17.4711662156183,70.7054028294192,12.0469650416352));
#57067=CARTESIAN_POINT('Ctrl Pts',(17.4757554134209,70.7578903102951,12.0136496158755));
#57068=CARTESIAN_POINT('Ctrl Pts',(17.4803446112235,70.8120511148244,11.9832907240565));
#57069=CARTESIAN_POINT('Ctrl Pts',(17.4849327680389,70.8661996338284,11.9529387186738));
#57070=CARTESIAN_POINT('Ctrl Pts',(17.4895209248543,70.9220202805256,11.9255421633639));
#57071=CARTESIAN_POINT('Ctrl Pts',(17.4941090816697,70.9791565474556,11.9012761563801));
#57072=CARTESIAN_POINT('Ctrl Pts',(17.4987381261593,71.0368019881473,11.8767939012106));
#57073=CARTESIAN_POINT('Ctrl Pts',(17.5033671706488,71.0957861455202,11.8554985051479));
#57074=CARTESIAN_POINT('Ctrl Pts',(17.5079962151384,71.1557227980214,11.8375199623082));
#57075=CARTESIAN_POINT('Ctrl Pts',(17.5125900826965,71.2152039812526,11.8196780416092));
#57076=CARTESIAN_POINT('Ctrl Pts',(17.5171839502547,71.2756227198441,11.8051028014983));
#57077=CARTESIAN_POINT('Ctrl Pts',(17.5217778178128,71.3365892191394,11.7938703101418));
#57078=CARTESIAN_POINT('Ctrl Pts',(17.5264244507681,71.3982559827556,11.7825088018165));
#57079=CARTESIAN_POINT('Ctrl Pts',(17.5310710837234,71.4604826448642,11.7745674065155));
#57080=CARTESIAN_POINT('Ctrl Pts',(17.5357177166786,71.5228609497408,11.7700708789007));
#57081=CARTESIAN_POINT('Ctrl Pts',(17.5403643496339,71.5852392546174,11.7655743512858));
#57082=CARTESIAN_POINT('Ctrl Pts',(17.5450109825892,71.647768671106,11.7645226378518));
#57083=CARTESIAN_POINT('Ctrl Pts',(17.5496576155444,71.7100440314096,11.7668863852335));
#57084=CARTESIAN_POINT('Ctrl Pts',(17.5542617775941,71.7717501858019,11.7692285276179));
#57085=CARTESIAN_POINT('Ctrl Pts',(17.5588659396438,71.8334508596207,11.774933159723));
#57086=CARTESIAN_POINT('Ctrl Pts',(17.5634701016935,71.8947508729253,11.7839991169126));
#57087=CARTESIAN_POINT('Ctrl Pts',(17.5680823078964,71.9561579864345,11.7930809136726));
#57088=CARTESIAN_POINT('Ctrl Pts',(17.5726945140993,72.0171625250871,11.8055358197998));
#57089=CARTESIAN_POINT('Ctrl Pts',(17.5773067203022,72.0773681587226,11.8213101124075));
#57090=CARTESIAN_POINT('Ctrl Pts',(17.5818986308978,72.1373088627685,11.8370149916295));
#57091=CARTESIAN_POINT('Ctrl Pts',(17.5864905414935,72.1964571786997,11.8560100030348));
#57092=CARTESIAN_POINT('Ctrl Pts',(17.5910824520891,72.2544304800156,11.878190743207));
#57093=CARTESIAN_POINT('Ctrl Pts',(17.5956716497601,72.3123695304044,11.9003583788827));
#57094=CARTESIAN_POINT('Ctrl Pts',(17.6002608474311,72.3691344701657,11.9257078297304));
#57095=CARTESIAN_POINT('Ctrl Pts',(17.6048500451021,72.4243592263726,11.9540853060779));
#57096=CARTESIAN_POINT('Ctrl Pts',(17.6094382017868,72.4795714557233,11.9824563454469));
#57097=CARTESIAN_POINT('Ctrl Pts',(17.6140263584714,72.5332437443721,12.0138538146624));
#57098=CARTESIAN_POINT('Ctrl Pts',(17.618614515156,72.585033200847,12.048077258264));
#57099=CARTESIAN_POINT('Ctrl Pts',(17.6232435597733,72.6372841855461,12.0826056883673));
#57100=CARTESIAN_POINT('Ctrl Pts',(17.6278726043905,72.6876181564677,12.1200104517166));
#57101=CARTESIAN_POINT('Ctrl Pts',(17.6325016490078,72.7357134062617,12.1600414083926));
#57102=CARTESIAN_POINT('Ctrl Pts',(17.6370955164387,72.7834431690703,12.1997681605215));
#57103=CARTESIAN_POINT('Ctrl Pts',(17.6416893838697,72.8289677814321,12.2420809370951));
#57104=CARTESIAN_POINT('Ctrl Pts',(17.6462832513006,72.8720085140621,12.2866968313951));
#57105=CARTESIAN_POINT('Ctrl Pts',(17.650929884511,72.9155436183387,12.3318251898606));
#57106=CARTESIAN_POINT('Ctrl Pts',(17.6555765177215,72.9565370577431,12.37930951984));
#57107=CARTESIAN_POINT('Ctrl Pts',(17.6602231509319,72.9947426792337,12.4288231804356));
#57108=CARTESIAN_POINT('Ctrl Pts',(17.6648697841423,73.0329483007243,12.4783368410311));
#57109=CARTESIAN_POINT('Ctrl Pts',(17.6695164173527,73.0683658554946,12.5298793599239));
#57110=CARTESIAN_POINT('Ctrl Pts',(17.6741630505631,73.1007959998186,12.583096781316));
#57111=CARTESIAN_POINT('Ctrl Pts',(17.6787672126947,73.132929726682,12.6358277857267));
#57112=CARTESIAN_POINT('Ctrl Pts',(17.6833713748263,73.1622575108099,12.6904116401468));
#57113=CARTESIAN_POINT('Ctrl Pts',(17.6879755369578,73.1885620280686,12.7465182858378));
#57114=CARTESIAN_POINT('Ctrl Pts',(17.6925877431505,73.214912502689,12.8027229570269));
#57115=CARTESIAN_POINT('Ctrl Pts',(17.6971999493432,73.2382288299098,12.8604553332266));
#57116=CARTESIAN_POINT('Ctrl Pts',(17.7018121555359,73.2583368619122,12.9193553640644));
#57117=CARTESIAN_POINT('Ctrl Pts',(17.7064040662101,73.2783564106775,12.9779962116365));
#57118=CARTESIAN_POINT('Ctrl Pts',(17.7109959768843,73.2951956498906,13.03779398638));
#57119=CARTESIAN_POINT('Ctrl Pts',(17.7155878875585,73.3087302479811,13.0983720654324));
#57120=CARTESIAN_POINT('Ctrl Pts',(17.7201770853067,73.3222568497568,13.158914354623));
#57121=CARTESIAN_POINT('Ctrl Pts',(17.7247662830548,73.3324825720767,13.2202355398255));
#57122=CARTESIAN_POINT('Ctrl Pts',(17.729355480803,73.3393333950186,13.2819455162975));
#57123=CARTESIAN_POINT('Ctrl Pts',(17.7339436375632,73.3461826639582,13.3436414948236));
#57124=CARTESIAN_POINT('Ctrl Pts',(17.7385317943235,73.3496584977824,13.4057255856276));
#57125=CARTESIAN_POINT('Ctrl Pts',(17.7431199510837,73.3497385816819,13.4678012297476));
#57126=CARTESIAN_POINT('Ctrl Pts',(17.7477489956252,73.3498193792564,13.530430066684));
#57127=CARTESIAN_POINT('Ctrl Pts',(17.7523780401667,73.346443567122,13.5930497816456));
#57128=CARTESIAN_POINT('Ctrl Pts',(17.7570070847083,73.3396419485777,13.6552540290513));
#57129=CARTESIAN_POINT('Ctrl Pts',(17.7616009522102,73.3328920168994,13.7169855738816));
#57130=CARTESIAN_POINT('Ctrl Pts',(17.766194819712,73.3227683069389,13.778307446046));
#57131=CARTESIAN_POINT('Ctrl Pts',(17.7707886872139,73.30935267667,13.8388310255427));
#57132=CARTESIAN_POINT('Ctrl Pts',(17.7754353202753,73.2957829533114,13.9000497841081));
#57133=CARTESIAN_POINT('Ctrl Pts',(17.7800819533366,73.2788453317756,13.9604512774611));
#57134=CARTESIAN_POINT('Ctrl Pts',(17.7847285863979,73.2586761210118,14.0196498821734));
#57135=CARTESIAN_POINT('Ctrl Pts',(17.7893752194593,73.2385069102479,14.0788484868857));
#57136=CARTESIAN_POINT('Ctrl Pts',(17.7940218525206,73.2151063665341,14.1368437346505));
#57137=CARTESIAN_POINT('Ctrl Pts',(17.7986684855819,73.188659425232,14.1932739329139));
#57138=CARTESIAN_POINT('Ctrl Pts',(17.8032726480834,73.1624542108728,14.2491883551123));
#57139=CARTESIAN_POINT('Ctrl Pts',(17.8078768105848,73.1331545058933,14.3037872928552));
#57140=CARTESIAN_POINT('Ctrl Pts',(17.8124809730863,73.1009153932975,14.3567072659418));
#57141=CARTESIAN_POINT('Ctrl Pts',(17.8170931792327,73.0686199577599,14.4097196922112));
#57142=CARTESIAN_POINT('Ctrl Pts',(17.8217053853791,73.0333750087894,14.461046798619));
#57143=CARTESIAN_POINT('Ctrl Pts',(17.8263175915256,72.9953844801837,14.5103445289244));
#57144=CARTESIAN_POINT('Ctrl Pts',(17.8309095025744,72.9575611213583,14.559425334353));
#57145=CARTESIAN_POINT('Ctrl Pts',(17.8355014136231,72.9170165837424,14.606494165908));
#57146=CARTESIAN_POINT('Ctrl Pts',(17.8400933246719,72.8739961339218,14.6512393387085));
#57147=CARTESIAN_POINT('Ctrl Pts',(17.8446825227953,72.8310011008107,14.6959580758239));
#57148=CARTESIAN_POINT('Ctrl Pts',(17.8492717209188,72.7855334073483,14.7383555119124));
#57149=CARTESIAN_POINT('Ctrl Pts',(17.8538609190422,72.7378773502305,14.7781544537375));
#57150=CARTESIAN_POINT('Ctrl Pts',(17.8584490761777,72.690232103145,14.8179443677942));
#57151=CARTESIAN_POINT('Ctrl Pts',(17.8630372333132,72.6403998672494,14.8551366331016));
#57152=CARTESIAN_POINT('Ctrl Pts',(17.8676253904487,72.5886988809515,14.8894935916712));
#57153=CARTESIAN_POINT('Ctrl Pts',(17.872254434628,72.5365371649029,14.9241567198923));
#57154=CARTESIAN_POINT('Ctrl Pts',(17.8768834788074,72.482473643401,14.9559334375672));
#57155=CARTESIAN_POINT('Ctrl Pts',(17.8815125229867,72.4268640547575,14.9846249590978));
#57156=CARTESIAN_POINT('Ctrl Pts',(17.8861063908595,72.371677045778,15.0130984525181));
#57157=CARTESIAN_POINT('Ctrl Pts',(17.8907002587324,72.3149678786595,15.0385333196578));
#57158=CARTESIAN_POINT('Ctrl Pts',(17.8952941266052,72.2571057184215,15.0607831246435));
#57159=CARTESIAN_POINT('Ctrl Pts',(17.8999407589378,72.1985789623117,15.0832884874666));
#57160=CARTESIAN_POINT('Ctrl Pts',(17.9045873912704,72.1388730591315,15.1025349754775));
#57161=CARTESIAN_POINT('Ctrl Pts',(17.909234023603,72.078384754109,15.1184231975768));
#57162=CARTESIAN_POINT('Ctrl Pts',(17.9138806559356,72.0178964490865,15.134311419676));
#57163=CARTESIAN_POINT('Ctrl Pts',(17.9185272882681,71.9566262741602,15.1468413308028));
#57164=CARTESIAN_POINT('Ctrl Pts',(17.9231739206007,71.894977887111,15.1559672932371));
#57165=CARTESIAN_POINT('Ctrl Pts',(17.9293625855438,71.8128708503543,15.1681217999306));
#57166=CARTESIAN_POINT('Ctrl Pts',(17.9355512504868,71.7298551795929,15.1742799717883));
#57167=CARTESIAN_POINT('Ctrl Pts',(17.9417399154298,71.6466202082904,15.1743395632009));
#57168=CARTESIAN_POINT('',(18.7354899154876,71.6451863826151,15.1743399866129));
#57169=CARTESIAN_POINT('Ctrl Pts',(17.9417399154741,71.6466202076947,15.1743395632013));
#57170=CARTESIAN_POINT('Ctrl Pts',(17.9462717923975,71.585668346648,15.1743832011778));
#57171=CARTESIAN_POINT('Ctrl Pts',(17.950803669321,71.5245990262305,15.1711528932889));
#57172=CARTESIAN_POINT('Ctrl Pts',(17.9553355462444,71.4637980963487,15.1646373016638));
#57173=CARTESIAN_POINT('Ctrl Pts',(17.9598626640451,71.4030610161902,15.1581285523472));
#57174=CARTESIAN_POINT('Ctrl Pts',(17.9643897818458,71.3425922856912,15.1483414059901));
#57175=CARTESIAN_POINT('Ctrl Pts',(17.9689168996465,71.2827767009868,15.1353165400646));
#57176=CARTESIAN_POINT('Ctrl Pts',(17.9734410287427,71.2230006052276,15.1223002728717));
#57177=CARTESIAN_POINT('Ctrl Pts',(17.9779651578389,71.1638773111853,15.1060506318105));
#57178=CARTESIAN_POINT('Ctrl Pts',(17.9824892869351,71.1057832030213,15.0866596883755));
#57179=CARTESIAN_POINT('Ctrl Pts',(17.9870121931421,71.0477047979148,15.0672739863861));
#57180=CARTESIAN_POINT('Ctrl Pts',(17.9915350993491,70.9906555229741,15.0447488323605));
#57181=CARTESIAN_POINT('Ctrl Pts',(17.9960580055561,70.9349961577852,15.0192260056449));
#57182=CARTESIAN_POINT('Ctrl Pts',(18.0005845415412,70.87929212416,14.9936826960374));
#57183=CARTESIAN_POINT('Ctrl Pts',(18.0051110775263,70.8249807064607,14.9651371243569));
#57184=CARTESIAN_POINT('Ctrl Pts',(18.0096376135114,70.7724008933841,14.9337784652904));
#57185=CARTESIAN_POINT('Ctrl Pts',(18.0141659003803,70.7198007422072,14.9024076765582));
#57186=CARTESIAN_POINT('Ctrl Pts',(18.0186941872493,70.6689339652024,14.8682219251408));
#57187=CARTESIAN_POINT('Ctrl Pts',(18.0232224741182,70.6201104803191,14.8314537217374));
#57188=CARTESIAN_POINT('Ctrl Pts',(18.0277588628083,70.5711996425019,14.7946197342047));
#57189=CARTESIAN_POINT('Ctrl Pts',(18.0322952514984,70.5243397990785,14.7551944049274));
#57190=CARTESIAN_POINT('Ctrl Pts',(18.0368316401885,70.4798068340605,14.7134498008023));
#57191=CARTESIAN_POINT('Ctrl Pts',(18.0404475453321,70.4443101012468,14.6801756395501));
#57192=CARTESIAN_POINT('Ctrl Pts',(18.0440634504758,70.4102911126563,14.6454287521193));
#57193=CARTESIAN_POINT('Ctrl Pts',(18.0476793556195,70.3778711177324,14.6093618249781));
#57194=CARTESIAN_POINT('Ctrl Pts',(18.0522835180563,70.3365904654751,14.5634375032501));
#57195=CARTESIAN_POINT('Ctrl Pts',(18.0568876804932,70.2977272769018,14.5151760381375));
#57196=CARTESIAN_POINT('Ctrl Pts',(18.06149184293,70.2615558534696,14.4648619068562));
#57197=CARTESIAN_POINT('Ctrl Pts',(18.0661040490845,70.225321236629,14.4144598741006));
#57198=CARTESIAN_POINT('Ctrl Pts',(18.070716255239,70.1917881761899,14.3619983451011));
#57199=CARTESIAN_POINT('Ctrl Pts',(18.0753284613936,70.161194047235,14.3077992154312));
#57200=CARTESIAN_POINT('Ctrl Pts',(18.0799203723543,70.1307345423091,14.2538385794021));
#57201=CARTESIAN_POINT('Ctrl Pts',(18.0845122833151,70.1031884329188,14.1981560322717));
#57202=CARTESIAN_POINT('Ctrl Pts',(18.0891041942758,70.0787471739964,14.1410989184725));
#57203=CARTESIAN_POINT('Ctrl Pts',(18.0936933923027,70.0543203551446,14.0840755144241));
#57204=CARTESIAN_POINT('Ctrl Pts',(18.0982825903297,70.0329949481222,14.0256796195907));
#57205=CARTESIAN_POINT('Ctrl Pts',(18.1028717883566,70.0149154324902,13.9662810803491));
#57206=CARTESIAN_POINT('Ctrl Pts',(18.1074599453874,69.9968400179464,13.906896014845));
#57207=CARTESIAN_POINT('Ctrl Pts',(18.1120481024182,69.9820091803124,13.8465092415604));
#57208=CARTESIAN_POINT('Ctrl Pts',(18.116636259449,69.9705177620195,13.7855064571404));
#57209=CARTESIAN_POINT('Ctrl Pts',(18.1212653037147,69.958923938269,13.7239600480877));
#57210=CARTESIAN_POINT('Ctrl Pts',(18.1258943479805,69.9507294795822,13.661787102663));
#57211=CARTESIAN_POINT('Ctrl Pts',(18.1305233922463,69.9459788150061,13.599392703017));
#57212=CARTESIAN_POINT('Ctrl Pts',(18.1351172599958,69.9412642511498,13.5374724439251));
#57213=CARTESIAN_POINT('Ctrl Pts',(18.1397111277453,69.9399412755248,13.4753345999021));
#57214=CARTESIAN_POINT('Ctrl Pts',(18.1443049954948,69.9420008739233,13.4133762162947));
#57215=CARTESIAN_POINT('Ctrl Pts',(18.1489516280187,69.9440841286939,13.3507061839613));
#57216=CARTESIAN_POINT('Ctrl Pts',(18.1535982605426,69.949628127205,13.2882202924725));
#57217=CARTESIAN_POINT('Ctrl Pts',(18.1582448930665,69.9585697815553,13.2263226523824));
#57218=CARTESIAN_POINT('Ctrl Pts',(18.1628915255904,69.9675114359056,13.1644250122922));
#57219=CARTESIAN_POINT('Ctrl Pts',(18.1675381581143,69.9798505802848,13.1031161310414));
#57220=CARTESIAN_POINT('Ctrl Pts',(18.1721847906382,69.9954719295671,13.0427855362965));
#57221=CARTESIAN_POINT('Ctrl Pts',(18.176788955474,70.0109505082331,12.9830063302976));
#57222=CARTESIAN_POINT('Ctrl Pts',(18.1813931203098,70.0297126859196,12.9239512599727));
#57223=CARTESIAN_POINT('Ctrl Pts',(18.1859972851456,70.051672849213,12.8660061221797));
#57224=CARTESIAN_POINT('Ctrl Pts',(18.1906094910002,70.0736713651922,12.8079597851546));
#57225=CARTESIAN_POINT('Ctrl Pts',(18.1952216968549,70.0988789650903,12.7510277683002));
#57226=CARTESIAN_POINT('Ctrl Pts',(18.1998339027095,70.1271584465421,12.69558575623));
#57227=CARTESIAN_POINT('Ctrl Pts',(18.2044258161163,70.1553135059884,12.640387673892));
#57228=CARTESIAN_POINT('Ctrl Pts',(18.2090177295231,70.1865132661784,12.5866669785811));
#57229=CARTESIAN_POINT('Ctrl Pts',(18.2136096429299,70.2205739447844,12.5347751350724));
#57230=CARTESIAN_POINT('Ctrl Pts',(18.2181988434134,70.2546145001867,12.4829139495009));
#57231=CARTESIAN_POINT('Ctrl Pts',(18.2227880438968,70.2915123441123,12.4328798960513));
#57232=CARTESIAN_POINT('Ctrl Pts',(18.2273772443803,70.3310389880981,12.3849977115267));
#57233=CARTESIAN_POINT('Ctrl Pts',(18.2319654038738,70.3705566660694,12.3371263883432));
#57234=CARTESIAN_POINT('Ctrl Pts',(18.2365535633674,70.4127016372396,12.2914063557475));
#57235=CARTESIAN_POINT('Ctrl Pts',(18.2411417228609,70.4572047813951,12.2481297294375));
#57236=CARTESIAN_POINT('Ctrl Pts',(18.2457707647606,70.5021044670432,12.2044674904182));
#57237=CARTESIAN_POINT('Ctrl Pts',(18.2503998066603,70.5494042079811,12.1632928081916));
#57238=CARTESIAN_POINT('Ctrl Pts',(18.2550288485599,70.5987908775215,12.1248664823354));
#57239=CARTESIAN_POINT('Ctrl Pts',(18.2596227187584,70.6478023045769,12.0867321217026));
#57240=CARTESIAN_POINT('Ctrl Pts',(18.2642165889569,70.6988686009911,12.0513047425673));
#57241=CARTESIAN_POINT('Ctrl Pts',(18.2688104591553,70.7516538167364,12.0187961564612));
#57242=CARTESIAN_POINT('Ctrl Pts',(18.2734570869056,70.8050452356688,11.9859142308087));
#57243=CARTESIAN_POINT('Ctrl Pts',(18.2781037146559,70.8601948474178,11.9560188353314));
#57244=CARTESIAN_POINT('Ctrl Pts',(18.2827503424062,70.916730944274,11.9292806086677));
#57245=CARTESIAN_POINT('Ctrl Pts',(18.2873969701565,70.9732670411301,11.902542382004));
#57246=CARTESIAN_POINT('Ctrl Pts',(18.2920435979068,71.0311891085112,11.8789614662436));
#57247=CARTESIAN_POINT('Ctrl Pts',(18.296690225657,71.0901087614014,11.8586569341274));
#57248=CARTESIAN_POINT('Ctrl Pts',(18.3012943804412,71.1484898533054,11.8385379976199));
#57249=CARTESIAN_POINT('Ctrl Pts',(18.3058985352253,71.2080811556222,11.821556207845));
#57250=CARTESIAN_POINT('Ctrl Pts',(18.3105026900094,71.2685137839003,11.8078533110119));
#57251=CARTESIAN_POINT('Ctrl Pts',(18.3151148971205,71.3290521043859,11.7941264488234));
#57252=CARTESIAN_POINT('Ctrl Pts',(18.3197271042316,71.3904342281563,11.7836901707823));
#57253=CARTESIAN_POINT('Ctrl Pts',(18.3243393113427,71.4522711997435,11.7766376341398));
#57254=CARTESIAN_POINT('Ctrl Pts',(18.3289312147021,71.5138359540407,11.7696161440116));
#57255=CARTESIAN_POINT('Ctrl Pts',(18.3335231180614,71.5758510573455,11.7659487512926));
#57256=CARTESIAN_POINT('Ctrl Pts',(18.3381150214207,71.6379220157181,11.7656764053294));
#57257=CARTESIAN_POINT('Ctrl Pts',(18.342704211887,71.6999563026153,11.7654042202679));
#57258=CARTESIAN_POINT('Ctrl Pts',(18.3472934023533,71.762045872943,11.7685231062559));
#57259=CARTESIAN_POINT('Ctrl Pts',(18.3518825928196,71.823793817313,11.7750219819878));
#57260=CARTESIAN_POINT('Ctrl Pts',(18.3564707423432,71.8855277557106,11.7815193836128));
#57261=CARTESIAN_POINT('Ctrl Pts',(18.3610588918667,71.9469197178515,11.7913951994893));
#57262=CARTESIAN_POINT('Ctrl Pts',(18.3656470413903,72.0075775420149,11.8045864586656));
#57263=CARTESIAN_POINT('Ctrl Pts',(18.3702760929974,72.0687761138982,11.8178953142678));
#57264=CARTESIAN_POINT('Ctrl Pts',(18.3749051446046,72.129226873885,11.8345789426527));
#57265=CARTESIAN_POINT('Ctrl Pts',(18.3795341962117,72.1885394510549,11.8545203893865));
#57266=CARTESIAN_POINT('Ctrl Pts',(18.3841280566705,72.2474011199443,11.8743102365123));
#57267=CARTESIAN_POINT('Ctrl Pts',(18.3887219171293,72.3051413956357,11.8973082953942));
#57268=CARTESIAN_POINT('Ctrl Pts',(18.3933157775881,72.3613981403934,11.9233515271552));
#57269=CARTESIAN_POINT('Ctrl Pts',(18.3979624247694,72.4183013151414,11.9496940141633));
#57270=CARTESIAN_POINT('Ctrl Pts',(18.4026090719507,72.4736861697953,11.9791518683659));
#57271=CARTESIAN_POINT('Ctrl Pts',(18.407255719132,72.5272051290434,12.011509496091));
#57272=CARTESIAN_POINT('Ctrl Pts',(18.4119023663132,72.5807240882916,12.0438671238161));
#57273=CARTESIAN_POINT('Ctrl Pts',(18.4165490134945,72.6323767494258,12.0791241745914));
#57274=CARTESIAN_POINT('Ctrl Pts',(18.4211956606758,72.6818493101953,12.1170226672277));
#57275=CARTESIAN_POINT('Ctrl Pts',(18.4257998281339,72.7308695920193,12.1545746912353));
#57276=CARTESIAN_POINT('Ctrl Pts',(18.430403995592,72.7779433012867,12.1948684785823));
#57277=CARTESIAN_POINT('Ctrl Pts',(18.43500816305,72.8227485102806,12.2376748314913));
#57278=CARTESIAN_POINT('Ctrl Pts',(18.4396203685769,72.8676319413103,12.2805559167839));
#57279=CARTESIAN_POINT('Ctrl Pts',(18.4442325741038,72.9102385090048,12.3259580752481));
#57280=CARTESIAN_POINT('Ctrl Pts',(18.4488447796306,72.9502757042091,12.3736085406367));
#57281=CARTESIAN_POINT('Ctrl Pts',(18.453436695458,72.990136770519,12.4210493853528));
#57282=CARTESIAN_POINT('Ctrl Pts',(18.4580286112853,73.0274506743401,12.4707184253993));
#57283=CARTESIAN_POINT('Ctrl Pts',(18.4626205271126,73.0619653640192,12.5223094360176));
#57284=CARTESIAN_POINT('Ctrl Pts',(18.4672097299348,73.0964596616579,12.5738699655283));
#57285=CARTESIAN_POINT('Ctrl Pts',(18.4717989327569,73.1281577436136,12.6273497928535));
#57286=CARTESIAN_POINT('Ctrl Pts',(18.4763881355791,73.1568495958325,12.6824119383474));
#57287=CARTESIAN_POINT('Ctrl Pts',(18.4809762973261,73.1855349392146,12.7374615928207));
#57288=CARTESIAN_POINT('Ctrl Pts',(18.4855644590732,73.211215172838,12.7940924030778));
#57289=CARTESIAN_POINT('Ctrl Pts',(18.4901526208202,73.2337261595506,12.8519426834936));
#57290=CARTESIAN_POINT('Ctrl Pts',(18.4947816603931,73.2564377059305,12.9103083759232));
#57291=CARTESIAN_POINT('Ctrl Pts',(18.4994106999659,73.2759230296784,12.9699149004168));
#57292=CARTESIAN_POINT('Ctrl Pts',(18.5040397395388,73.2920639842587,13.0303722500284));
#57293=CARTESIAN_POINT('Ctrl Pts',(18.5086336117589,73.3080823141274,13.0903702981142));
#57294=CARTESIAN_POINT('Ctrl Pts',(18.5132274839791,73.3208068662135,13.1512057732044));
#57295=CARTESIAN_POINT('Ctrl Pts',(18.5178213561992,73.3301735030541,13.2124867401343));
#57296=CARTESIAN_POINT('Ctrl Pts',(18.5224679794484,73.3396476961586,13.2744713909966));
#57297=CARTESIAN_POINT('Ctrl Pts',(18.5271146026976,73.3456862965543,13.3369113020137));
#57298=CARTESIAN_POINT('Ctrl Pts',(18.5317612259469,73.3482770197843,13.3993976552055));
#57299=CARTESIAN_POINT('Ctrl Pts',(18.5364078491961,73.3508677430143,13.4618840083973));
#57300=CARTESIAN_POINT('Ctrl Pts',(18.5410544724453,73.3500106587655,13.524416274497));
#57301=CARTESIAN_POINT('Ctrl Pts',(18.5457010956945,73.3457474705212,13.5865903730673));
#57302=CARTESIAN_POINT('Ctrl Pts',(18.5503052764862,73.3415232224227,13.6481965707345));
#57303=CARTESIAN_POINT('Ctrl Pts',(18.5549094572779,73.333938189835,13.7096946632185));
#57304=CARTESIAN_POINT('Ctrl Pts',(18.5595136380695,73.3230055995048,13.7706896874024));
#57305=CARTESIAN_POINT('Ctrl Pts',(18.5641258419297,73.3120539584629,13.8317909991711));
#57306=CARTESIAN_POINT('Ctrl Pts',(18.5687380457898,73.2977430700227,13.8923869741468));
#57307=CARTESIAN_POINT('Ctrl Pts',(18.57335024965,73.2801387287715,13.9520831092813));
#57308=CARTESIAN_POINT('Ctrl Pts',(18.5779421792581,73.2626117724025,14.0115168330985));
#57309=CARTESIAN_POINT('Ctrl Pts',(18.5825341088662,73.2418203745654,14.0700581154847));
#57310=CARTESIAN_POINT('Ctrl Pts',(18.5871260384743,73.2178805692773,14.1273276921333));
#57311=CARTESIAN_POINT('Ctrl Pts',(18.5917152552039,73.1939549074511,14.1845634343347));
#57312=CARTESIAN_POINT('Ctrl Pts',(18.5963044719336,73.1668847223054,14.2405284937931));
#57313=CARTESIAN_POINT('Ctrl Pts',(18.6008936886632,73.1368349058593,14.2948616594219));
#57314=CARTESIAN_POINT('Ctrl Pts',(18.6054818644196,73.1067919056215,14.3491825006437));
#57315=CARTESIAN_POINT('Ctrl Pts',(18.6100700401759,73.0737708615674,14.4018717394724));
#57316=CARTESIAN_POINT('Ctrl Pts',(18.6146582159323,73.037982602253,14.4525927597444));
#57317=CARTESIAN_POINT('Ctrl Pts',(18.619287242164,73.0018757048819,14.5037653707796));
#57318=CARTESIAN_POINT('Ctrl Pts',(18.6239162683958,72.9629523455289,14.5529340929907));
#57319=CARTESIAN_POINT('Ctrl Pts',(18.6285452946276,72.9214723610863,14.5997850082523));
#57320=CARTESIAN_POINT('Ctrl Pts',(18.633139180939,72.880307260007,14.6462802682752));
#57321=CARTESIAN_POINT('Ctrl Pts',(18.6377330672504,72.8366246183834,14.6904924650606));
#57322=CARTESIAN_POINT('Ctrl Pts',(18.6423269535618,72.7907157191772,14.7321516307503));
#57323=CARTESIAN_POINT('Ctrl Pts',(18.6469735497538,72.7442800649696,14.7742887903423));
#57324=CARTESIAN_POINT('Ctrl Pts',(18.6516201459457,72.6955671421928,14.8138136103111));
#57325=CARTESIAN_POINT('Ctrl Pts',(18.6562667421376,72.6449109413609,14.8504900266572));
#57326=CARTESIAN_POINT('Ctrl Pts',(18.6609133383295,72.594254740529,14.8871664430032));
#57327=CARTESIAN_POINT('Ctrl Pts',(18.6655599345214,72.5416557412991,14.9209942214633));
#57328=CARTESIAN_POINT('Ctrl Pts',(18.6702065307133,72.4874738068746,14.9517849167054));
#57329=CARTESIAN_POINT('Ctrl Pts',(18.6749930460121,72.4316603366847,14.9835027866795));
#57330=CARTESIAN_POINT('Ctrl Pts',(18.6797795613109,72.373961918635,15.0121150505961));
#57331=CARTESIAN_POINT('Ctrl Pts',(18.6845660766097,72.3147425716321,15.0374040185609));
#57332=CARTESIAN_POINT('Ctrl Pts',(18.6893401544225,72.2556771027128,15.0626272745899));
#57333=CARTESIAN_POINT('Ctrl Pts',(18.6941142322353,72.1950989810462,15.0845442444087));
#57334=CARTESIAN_POINT('Ctrl Pts',(18.698888310048,72.1333960632559,15.1029833672903));
#57335=CARTESIAN_POINT('Ctrl Pts',(18.7036549356628,72.0717894619435,15.121393707232));
#57336=CARTESIAN_POINT('Ctrl Pts',(18.7084215612776,72.009061981251,15.1363368575986));
#57337=CARTESIAN_POINT('Ctrl Pts',(18.7131881868923,71.9456203696711,15.1476896510483));
#57338=CARTESIAN_POINT('Ctrl Pts',(18.717946530032,71.8822889940553,15.1590227179163));
#57339=CARTESIAN_POINT('Ctrl Pts',(18.7227048731716,71.8182463977651,15.1667777619715));
#57340=CARTESIAN_POINT('Ctrl Pts',(18.7274632163113,71.7539115768951,15.1708821456173));
#57341=CARTESIAN_POINT('Ctrl Pts',(18.7301387826841,71.7177367827973,15.173189997435));
#57342=CARTESIAN_POINT('Ctrl Pts',(18.732814349057,71.6814698195352,15.1743445342645));
#57343=CARTESIAN_POINT('Ctrl Pts',(18.7354899154298,71.6451863833987,15.174339986613));
#57344=CARTESIAN_POINT('Ctrl Pts',(18.7354899154876,71.6451863826151,15.1743399866129));
#57345=CARTESIAN_POINT('Ctrl Pts',(18.7404250863413,71.5782603820836,15.1743315982882));
#57346=CARTESIAN_POINT('Ctrl Pts',(18.745360257195,71.5114232487074,15.1703765618724));
#57347=CARTESIAN_POINT('Ctrl Pts',(18.7502954280487,71.4451369577199,15.1625334707168));
#57348=CARTESIAN_POINT('Ctrl Pts',(18.7551622095479,71.3797692320236,15.1547990655536));
#57349=CARTESIAN_POINT('Ctrl Pts',(18.7600289910471,71.3149375632485,15.1432838780447));
#57350=CARTESIAN_POINT('Ctrl Pts',(18.7648957725463,71.2510718358305,15.1280953333698));
#57351=CARTESIAN_POINT('Ctrl Pts',(18.7698651380773,71.185859920216,15.1125866382732));
#57352=CARTESIAN_POINT('Ctrl Pts',(18.7748345036083,71.1216555675429,15.0932481155449));
#57353=CARTESIAN_POINT('Ctrl Pts',(18.7798038691392,71.0588960841977,15.0702462286625));
#57354=CARTESIAN_POINT('Ctrl Pts',(18.7847732346702,70.9961366008525,15.0472443417801));
#57355=CARTESIAN_POINT('Ctrl Pts',(18.7897426002011,70.9348223677971,15.0205793412336));
#57356=CARTESIAN_POINT('Ctrl Pts',(18.7947119657321,70.8753642096513,14.9904669405094));
#57357=CARTESIAN_POINT('Ctrl Pts',(18.799316195139,70.8202748831543,14.962567121093));
#57358=CARTESIAN_POINT('Ctrl Pts',(18.803920424546,70.7665949169974,14.9316143274008));
#57359=CARTESIAN_POINT('Ctrl Pts',(18.8085246539529,70.7146828958061,14.8977746697434));
#57360=CARTESIAN_POINT('Ctrl Pts',(18.8131368517362,70.6626810323236,14.8638764469925));
#57361=CARTESIAN_POINT('Ctrl Pts',(18.8177490495194,70.6124537165645,14.8270815477019));
#57362=CARTESIAN_POINT('Ctrl Pts',(18.8223612473027,70.564338610821,14.7876043064693));
#57363=CARTESIAN_POINT('Ctrl Pts',(18.8269532238489,70.5164344559088,14.7483001451194));
#57364=CARTESIAN_POINT('Ctrl Pts',(18.8315452003952,70.4706244396919,14.70633741437));
#57365=CARTESIAN_POINT('Ctrl Pts',(18.8361371769414,70.4272126232424,14.6619707843351));
#57366=CARTESIAN_POINT('Ctrl Pts',(18.8407264398518,70.3838264610755,14.6176303728315));
#57367=CARTESIAN_POINT('Ctrl Pts',(18.8453157027621,70.3428360420209,14.5708892411813));
#57368=CARTESIAN_POINT('Ctrl Pts',(18.8499049656725,70.3045097605242,14.5220400188578));
#57369=CARTESIAN_POINT('Ctrl Pts',(18.8544931867798,70.2661921794301,14.4732018857371));
#57370=CARTESIAN_POINT('Ctrl Pts',(18.8590814078871,70.2305378478503,14.4222570110851));
#57371=CARTESIAN_POINT('Ctrl Pts',(18.8636696289945,70.1977746077564,14.3695307439613));
#57372=CARTESIAN_POINT('Ctrl Pts',(18.8682986099742,70.1647203124902,14.3163360783301));
#57373=CARTESIAN_POINT('Ctrl Pts',(18.8729275909539,70.1346090361727,14.2613286395754));
#57374=CARTESIAN_POINT('Ctrl Pts',(18.8775565719336,70.1076286077453,14.204870043452));
#57375=CARTESIAN_POINT('Ctrl Pts',(18.8821505010633,70.0808524821512,14.1488389665277));
#57376=CARTESIAN_POINT('Ctrl Pts',(18.8867444301931,70.0571600946983,14.0913791310703));
#57377=CARTESIAN_POINT('Ctrl Pts',(18.8913383593228,70.0366865554042,14.0328640055793));
#57378=CARTESIAN_POINT('Ctrl Pts',(18.8959848662275,70.0159786953117,13.9736791712154));
#57379=CARTESIAN_POINT('Ctrl Pts',(18.9006313731322,69.9985639957566,13.9134152439124));
#57380=CARTESIAN_POINT('Ctrl Pts',(18.9052778800368,69.9845296933773,13.8524717769704));
#57381=CARTESIAN_POINT('Ctrl Pts',(18.9099243869415,69.9704953909979,13.7915283100284));
#57382=CARTESIAN_POINT('Ctrl Pts',(18.9145708938462,69.9598415146185,13.7299058363891));
#57383=CARTESIAN_POINT('Ctrl Pts',(18.9192174007509,69.9526013703753,13.6680091794354));
#57384=CARTESIAN_POINT('Ctrl Pts',(18.9238216793447,69.945427025897,13.6066750507048));
#57385=CARTESIAN_POINT('Ctrl Pts',(18.9284259579385,69.9415762144442,13.5448293225974));
#57386=CARTESIAN_POINT('Ctrl Pts',(18.9330302365323,69.941108538074,13.4828626749172));
#57387=CARTESIAN_POINT('Ctrl Pts',(18.9376424281672,69.9406400579421,13.4207895296351));
#57388=CARTESIAN_POINT('Ctrl Pts',(18.9422546198021,69.9435664584075,13.3585955513503));
#57389=CARTESIAN_POINT('Ctrl Pts',(18.946866811437,69.9498955848858,13.2966806014082));
#57390=CARTESIAN_POINT('Ctrl Pts',(18.9514588412422,69.95619704409,13.2350363077556));
#57391=CARTESIAN_POINT('Ctrl Pts',(18.9560508710474,69.965871517759,13.1736691171281));
#57392=CARTESIAN_POINT('Ctrl Pts',(18.9606429008527,69.9788746679288,13.1129731758468));
#57393=CARTESIAN_POINT('Ctrl Pts',(18.9652322183829,69.9918701378089,13.0523130845251));
#57394=CARTESIAN_POINT('Ctrl Pts',(18.9698215359132,70.0081902789825,12.992323951191));
#57395=CARTESIAN_POINT('Ctrl Pts',(18.9744108534434,70.027739409392,12.9333911581107));
#57396=CARTESIAN_POINT('Ctrl Pts',(18.9789991304254,70.047284107375,12.8744717270197));
#57397=CARTESIAN_POINT('Ctrl Pts',(18.9835874074075,70.0700561811619,12.8166086417205));
#57398=CARTESIAN_POINT('Ctrl Pts',(18.9881756843895,70.0959102736314,12.7601715534875));
#57399=CARTESIAN_POINT('Ctrl Pts',(18.9928046136712,70.1219934342932,12.7032344306163));
#57400=CARTESIAN_POINT('Ctrl Pts',(18.9974335429529,70.1512133108252,12.647749189379));
#57401=CARTESIAN_POINT('Ctrl Pts',(19.0020624722345,70.1833722265965,12.5940721345927));
#57402=CARTESIAN_POINT('Ctrl Pts',(19.006656459615,70.2152883878152,12.5408002660236));
#57403=CARTESIAN_POINT('Ctrl Pts',(19.0112504469955,70.2500990333393,12.4893097723984));
#57404=CARTESIAN_POINT('Ctrl Pts',(19.015844434376,70.2875674718241,12.4399195851646));
#57405=CARTESIAN_POINT('Ctrl Pts',(19.0204908346083,70.3254633881294,12.3899659047496));
#57406=CARTESIAN_POINT('Ctrl Pts',(19.0251372348405,70.3660777959415,12.342161175751));
#57407=CARTESIAN_POINT('Ctrl Pts',(19.0297836350728,70.4091258464664,12.2967988011834));
#57408=CARTESIAN_POINT('Ctrl Pts',(19.0344300353051,70.4521738969912,12.2514364266159));
#57409=CARTESIAN_POINT('Ctrl Pts',(19.0390764355373,70.4976551619854,12.2085167248299));
#57410=CARTESIAN_POINT('Ctrl Pts',(19.0437228357696,70.5452506138259,12.1682910602978));
#57411=CARTESIAN_POINT('Ctrl Pts',(19.0483264546595,70.5924078345151,12.1284357702152));
#57412=CARTESIAN_POINT('Ctrl Pts',(19.0529300735493,70.641826949787,12.0910674439044));
#57413=CARTESIAN_POINT('Ctrl Pts',(19.0575336924392,70.6932153353122,12.0564515572739));
#57414=CARTESIAN_POINT('Ctrl Pts',(19.0621459665371,70.7447003355176,12.0217705897349));
#57415=CARTESIAN_POINT('Ctrl Pts',(19.066758240635,70.7981616585012,11.9898527893657));
#57416=CARTESIAN_POINT('Ctrl Pts',(19.0713705147328,70.8532702678118,11.9609256734728));
#57417=CARTESIAN_POINT('Ctrl Pts',(19.0759618820208,70.9081290773066,11.9321296802541));
#57418=CARTESIAN_POINT('Ctrl Pts',(19.0805532493088,70.9646198330223,11.906297577776));
#57419=CARTESIAN_POINT('Ctrl Pts',(19.0851446165967,71.0223895875124,11.883610116796));
#57420=CARTESIAN_POINT('Ctrl Pts',(19.0897332724557,71.0801252261114,11.8609360538814));
#57421=CARTESIAN_POINT('Ctrl Pts',(19.0943219283147,71.1391378942585,11.841403134612));
#57422=CARTESIAN_POINT('Ctrl Pts',(19.0989105841737,71.1990535842303,11.8251444705599));
#57423=CARTESIAN_POINT('Ctrl Pts',(19.1034982014551,71.2589557131298,11.8088894864275));
#57424=CARTESIAN_POINT('Ctrl Pts',(19.1080858187364,71.3197599685948,11.7959074186996));
#57425=CARTESIAN_POINT('Ctrl Pts',(19.1126734360178,71.3810780140583,11.7862812814048));
#57426=CARTESIAN_POINT('Ctrl Pts',(19.1173030055821,71.4429567933031,11.7765671161841));
#57427=CARTESIAN_POINT('Ctrl Pts',(19.1219325751463,71.5053582945914,11.770270688795));
#57428=CARTESIAN_POINT('Ctrl Pts',(19.1265621447105,71.5678760653021,11.7674240471718));
#57429=CARTESIAN_POINT('Ctrl Pts',(19.1311554848484,71.6299045933452,11.7645996823912));
#57430=CARTESIAN_POINT('Ctrl Pts',(19.1357488249864,71.6920470637278,11.7651712377844));
#57431=CARTESIAN_POINT('Ctrl Pts',(19.1403421651244,71.7539069697206,11.769117560464));
#57432=CARTESIAN_POINT('Ctrl Pts',(19.1449898494017,71.8164987447354,11.7731105723726));
#57433=CARTESIAN_POINT('Ctrl Pts',(19.149637533679,71.8788006939132,11.780558684302));
#57434=CARTESIAN_POINT('Ctrl Pts',(19.1542852179564,71.9404105001401,11.791386393357));
#57435=CARTESIAN_POINT('Ctrl Pts',(19.1589329022337,72.0020203063669,11.802214102412));
#57436=CARTESIAN_POINT('Ctrl Pts',(19.1635805865111,72.0629374665644,11.8164212268768));
#57437=CARTESIAN_POINT('Ctrl Pts',(19.1682282707884,72.1227758668436,11.8338804697225));
#57438=CARTESIAN_POINT('Ctrl Pts',(19.1728331735793,72.1820634604063,11.851179001918));
#57439=CARTESIAN_POINT('Ctrl Pts',(19.1774380763701,72.240526620572,11.8717384059336));
#57440=CARTESIAN_POINT('Ctrl Pts',(19.1820429791609,72.2977822570827,11.8954612655626));
#57441=CARTESIAN_POINT('Ctrl Pts',(19.1866550927712,72.3551275502217,11.9192212728288));
#57442=CARTESIAN_POINT('Ctrl Pts',(19.1912672063814,72.4112610313227,11.9461545520894));
#57443=CARTESIAN_POINT('Ctrl Pts',(19.1958793199917,72.465811495844,11.9761125165907));
#57444=CARTESIAN_POINT('Ctrl Pts',(19.2004719605371,72.5201316397738,12.0059439938812));
#57445=CARTESIAN_POINT('Ctrl Pts',(19.2050646010825,72.5728816480386,12.0387744470168));
#57446=CARTESIAN_POINT('Ctrl Pts',(19.2096572416279,72.6237157481518,12.0744093965212));
#57447=CARTESIAN_POINT('Ctrl Pts',(19.2142471631464,72.6745197524455,12.110023248711));
#57448=CARTESIAN_POINT('Ctrl Pts',(19.218837084665,72.7234096838212,12.1484380138804));
#57449=CARTESIAN_POINT('Ctrl Pts',(19.2234270061836,72.7700678497869,12.1894153431906));
#57450=CARTESIAN_POINT('Ctrl Pts',(19.2280158794259,72.8167153596549,12.2303833138297));
#57451=CARTESIAN_POINT('Ctrl Pts',(19.2326047526681,72.8611317355008,12.2739123520018));
#57452=CARTESIAN_POINT('Ctrl Pts',(19.2371936259103,72.9030331290775,12.3197244902865));
#57453=CARTESIAN_POINT('Ctrl Pts',(19.2418219659017,72.9452948969125,12.3659306373128));
#57454=CARTESIAN_POINT('Ctrl Pts',(19.2464503058931,72.9849978358667,12.414458981884));
#57455=CARTESIAN_POINT('Ctrl Pts',(19.2510786458845,73.0218909603376,12.4649888201075));
#57456=CARTESIAN_POINT('Ctrl Pts',(19.2556732038974,73.0585148040855,12.5151498440448));
#57457=CARTESIAN_POINT('Ctrl Pts',(19.2602677619103,73.0923694824295,12.5672827792031));
#57458=CARTESIAN_POINT('Ctrl Pts',(19.2648623199231,73.1232534334683,12.6210453105224));
#57459=CARTESIAN_POINT('Ctrl Pts',(19.2695075509038,73.1544780008302,12.6754007839727));
#57460=CARTESIAN_POINT('Ctrl Pts',(19.2741527818845,73.1826656578134,12.7314215526223));
#57461=CARTESIAN_POINT('Ctrl Pts',(19.2787980128652,73.2076572814218,12.7887313142051));
#57462=CARTESIAN_POINT('Ctrl Pts',(19.2834432438458,73.2326489050301,12.846041075788));
#57463=CARTESIAN_POINT('Ctrl Pts',(19.2880884748265,73.254444369023,12.9046393130213));
#57464=CARTESIAN_POINT('Ctrl Pts',(19.2927337058072,73.2729365026424,12.9641346343478));
#57465=CARTESIAN_POINT('Ctrl Pts',(19.297338464396,73.2912675202953,13.0231115922232));
#57466=CARTESIAN_POINT('Ctrl Pts',(19.3019432229847,73.3064248298589,13.0832024627714));
#57467=CARTESIAN_POINT('Ctrl Pts',(19.3065479815735,73.3182780745141,13.1440340763056));
#57468=CARTESIAN_POINT('Ctrl Pts',(19.311160113209,73.330150298346,13.2049630921949));
#57469=CARTESIAN_POINT('Ctrl Pts',(19.3157722448445,73.3387076718679,13.2666347506746));
#57470=CARTESIAN_POINT('Ctrl Pts',(19.32038437648,73.343869055285,13.328657494577));
#57471=CARTESIAN_POINT('Ctrl Pts',(19.3249769086041,73.3490085051144,13.3904166693586));
#57472=CARTESIAN_POINT('Ctrl Pts',(19.3295694407281,73.3507806986223,13.4525234472179));
#57473=CARTESIAN_POINT('Ctrl Pts',(19.3341619728522,73.3491568095592,13.5145821655008));
#57474=CARTESIAN_POINT('Ctrl Pts',(19.3387517995581,73.3475338771141,13.5766043255676));
#57475=CARTESIAN_POINT('Ctrl Pts',(19.343341626264,73.3425188430167,13.6385779763424));
#57476=CARTESIAN_POINT('Ctrl Pts',(19.3479314529699,73.3341349614926,13.7001066392624));
#57477=CARTESIAN_POINT('Ctrl Pts',(19.3525202450466,73.3257529698456,13.7616214325192));
#57478=CARTESIAN_POINT('Ctrl Pts',(19.3571090371233,73.3140037072191,13.8226909349592));
#57479=CARTESIAN_POINT('Ctrl Pts',(19.3616978292,73.2989621474886,13.882925005289));
#57480=CARTESIAN_POINT('Ctrl Pts',(19.3663262718355,73.2837906175528,13.9436795425534));
#57481=CARTESIAN_POINT('Ctrl Pts',(19.370954714471,73.2652697138045,14.0035836244977));
#57482=CARTESIAN_POINT('Ctrl Pts',(19.3755831571065,73.243528201611,14.0622508647656));
#57483=CARTESIAN_POINT('Ctrl Pts',(19.3801776678416,73.2219460801423,14.120488005514));
#57484=CARTESIAN_POINT('Ctrl Pts',(19.3847721785767,73.1971906715339,14.1775059306295));
#57485=CARTESIAN_POINT('Ctrl Pts',(19.3893666893118,73.1694360388153,14.2329475656899));
#57486=CARTESIAN_POINT('Ctrl Pts',(19.3940120978975,73.1413739411171,14.2890033815022));
#57487=CARTESIAN_POINT('Ctrl Pts',(19.3986575064832,73.110246008635,14.3434472988074));
#57488=CARTESIAN_POINT('Ctrl Pts',(19.4033029150688,73.076278106149,14.3959388105827));
#57489=CARTESIAN_POINT('Ctrl Pts',(19.4079483236545,73.0423102036631,14.4484303223581));
#57490=CARTESIAN_POINT('Ctrl Pts',(19.4125937322402,73.0055026928797,14.4989690376699));
#57491=CARTESIAN_POINT('Ctrl Pts',(19.4172391408259,72.9661227118731,14.5472494390542));
#57492=CARTESIAN_POINT('Ctrl Pts',(19.4219058397656,72.9265622486294,14.5957511141574));
#57493=CARTESIAN_POINT('Ctrl Pts',(19.4265725387052,72.8842352513501,14.6421822266909));
#57494=CARTESIAN_POINT('Ctrl Pts',(19.4312392376448,72.8393915776516,14.6862067867337));
#57495=CARTESIAN_POINT('Ctrl Pts',(19.4357752167816,72.7958040287347,14.7289981663452));
#57496=CARTESIAN_POINT('Ctrl Pts',(19.4403111959183,72.7498393319997,14.7695156363342));
#57497=CARTESIAN_POINT('Ctrl Pts',(19.4448471750551,72.7017686549099,14.8074827477481));
#57498=CARTESIAN_POINT('Ctrl Pts',(19.4493789194439,72.6537428561569,14.8454144134201));
#57499=CARTESIAN_POINT('Ctrl Pts',(19.4539106638327,72.6036153791354,14.8808001147534));
#57500=CARTESIAN_POINT('Ctrl Pts',(19.4584424082216,72.5516925959545,14.9134017341399));
#57501=CARTESIAN_POINT('Ctrl Pts',(19.4629716795609,72.4997981479139,14.9459855622717));
#57502=CARTESIAN_POINT('Ctrl Pts',(19.4675009509002,72.4461107770265,14.9757880429932));
#57503=CARTESIAN_POINT('Ctrl Pts',(19.4720302222396,72.3909663220636,15.0026140071801));
#57504=CARTESIAN_POINT('Ctrl Pts',(19.4765587783873,72.33583057465,15.0294357354305));
#57505=CARTESIAN_POINT('Ctrl Pts',(19.481087334535,72.2792386699189,15.0532816536205));
#57506=CARTESIAN_POINT('Ctrl Pts',(19.4856158906827,72.221549564604,15.0740032776795));
#57507=CARTESIAN_POINT('Ctrl Pts',(19.4901480107099,72.1638150591632,15.0947412092257));
#57508=CARTESIAN_POINT('Ctrl Pts',(19.4946801307371,72.1049821223312,15.1123497644502));
#57509=CARTESIAN_POINT('Ctrl Pts',(19.4992122507643,72.0454266369115,15.1267297683573));
#57510=CARTESIAN_POINT('Ctrl Pts',(19.5037465866609,71.9858420332909,15.1411168030164));
#57511=CARTESIAN_POINT('Ctrl Pts',(19.5082809225576,71.9255346914762,15.1522720511605));
#57512=CARTESIAN_POINT('Ctrl Pts',(19.5128152584543,71.8648895078128,15.1601476833579));
#57513=CARTESIAN_POINT('Ctrl Pts',(19.5173562582881,71.8041551962814,15.1680348900657));
#57514=CARTESIAN_POINT('Ctrl Pts',(19.5218972581218,71.7430825723748,15.1726328329929));
#57515=CARTESIAN_POINT('Ctrl Pts',(19.5264382579556,71.6820588908945,15.1739457037472));
#57516=CARTESIAN_POINT('Ctrl Pts',(19.5273721437628,71.6695089785131,15.1742157040574));
#57517=CARTESIAN_POINT('Ctrl Pts',(19.5283060295701,71.6569611230376,15.174346939252));
#57518=CARTESIAN_POINT('Ctrl Pts',(19.5292399153773,71.6444186650849,15.1743397174806));
#57519=CARTESIAN_POINT('Origin',(21.26284859951,71.6454,13.47));
#57520=CARTESIAN_POINT('',(13.939,70.3906268762381,13.2739275442987));
#57521=CARTESIAN_POINT('Ctrl Pts',(13.939,70.3906268762381,13.2739275442987));
#57522=CARTESIAN_POINT('Ctrl Pts',(13.939476998378,70.3913557976579,13.2692627840007));
#57523=CARTESIAN_POINT('Ctrl Pts',(13.9399552893779,70.3921107122386,13.2646022132722));
#57524=CARTESIAN_POINT('Ctrl Pts',(13.9417487187488,70.3950313405543,13.2471871084459));
#57525=CARTESIAN_POINT('Ctrl Pts',(13.9430715863859,70.3973657981373,13.2344624073896));
#57526=CARTESIAN_POINT('Ctrl Pts',(13.950929094055,70.4123016062837,13.1595193368332));
#57527=CARTESIAN_POINT('Ctrl Pts',(13.9576152221227,70.4293582572828,13.0982868263952));
#57528=CARTESIAN_POINT('Ctrl Pts',(13.9724334320229,70.477206094675,12.9658055514468));
#57529=CARTESIAN_POINT('Ctrl Pts',(13.9805257607193,70.5100971774642,12.8955603370341));
#57530=CARTESIAN_POINT('Ctrl Pts',(13.9915151991299,70.5644934030398,12.8025722603859));
#57531=CARTESIAN_POINT('Ctrl Pts',(13.9945760543604,70.5807325852423,12.7769613699378));
#57532=CARTESIAN_POINT('Ctrl Pts',(13.9999561130953,70.6111811584152,12.7325413362383));
#57533=CARTESIAN_POINT('Ctrl Pts',(14.0022870448487,70.6250256515042,12.7135013133656));
#57534=CARTESIAN_POINT('Ctrl Pts',(14.0074424274966,70.6570574216567,12.6719294521042));
#57535=CARTESIAN_POINT('Ctrl Pts',(14.0102556756569,70.6755022934806,12.6496120495138));
#57536=CARTESIAN_POINT('Ctrl Pts',(14.0192439504941,70.7373428187729,12.5797925150066));
#57537=CARTESIAN_POINT('Ctrl Pts',(14.0253074478497,70.7835894852584,12.5349484414327));
#57538=CARTESIAN_POINT('Ctrl Pts',(14.0364660638293,70.8747173866202,12.4591151619936));
#57539=CARTESIAN_POINT('Ctrl Pts',(14.0415533847315,70.9185697641717,12.4271400924489));
#57540=CARTESIAN_POINT('Ctrl Pts',(14.0489162665172,70.9835928044448,12.3858264743385));
#57541=CARTESIAN_POINT('Ctrl Pts',(14.0511133230423,71.0031832515459,12.3741083681617));
#57542=CARTESIAN_POINT('Ctrl Pts',(14.0551429109317,71.0392651346352,12.3538255569822));
#57543=CARTESIAN_POINT('Ctrl Pts',(14.0569665926813,71.0556493201144,12.3450827300574));
#57544=CARTESIAN_POINT('Ctrl Pts',(14.060168130926,71.0844074382759,12.3305378698528));
#57545=CARTESIAN_POINT('Ctrl Pts',(14.0615366605854,71.09669384579,12.3245707853382));
#57546=CARTESIAN_POINT('Ctrl Pts',(14.0646364920111,71.1245061322962,12.3116134381408));
#57547=CARTESIAN_POINT('Ctrl Pts',(14.0663729254254,71.1400801522094,12.3047353950554));
#57548=CARTESIAN_POINT('Ctrl Pts',(14.0744847022017,71.2129275096061,12.2742982535752));
#57549=CARTESIAN_POINT('Ctrl Pts',(14.0809988379883,71.2717322723212,12.2546375391324));
#57550=CARTESIAN_POINT('Ctrl Pts',(14.094817689829,71.3991004994873,12.2221737653857));
#57551=CARTESIAN_POINT('Ctrl Pts',(14.1020964281858,71.4677780606284,12.2105608141454));
#57552=CARTESIAN_POINT('Ctrl Pts',(14.1127095020675,71.5708939392687,12.2017329677886));
#57553=CARTESIAN_POINT('Ctrl Pts',(14.1161534156613,71.6048236442353,12.2001943015546));
#57554=CARTESIAN_POINT('Ctrl Pts',(14.1219322244582,71.6624682015945,12.199893744023));
#57555=CARTESIAN_POINT('Ctrl Pts',(14.1242866410912,71.6861587520721,12.2004330910749));
#57556=CARTESIAN_POINT('Ctrl Pts',(14.129233621627,71.7362907908017,12.2029793813775));
#57557=CARTESIAN_POINT('Ctrl Pts',(14.1318200410207,71.7627127605111,12.2051520480678));
#57558=CARTESIAN_POINT('Ctrl Pts',(14.1394804903234,71.8413684315128,12.2141062568121));
#57559=CARTESIAN_POINT('Ctrl Pts',(14.1444814921371,71.8932710306063,12.2233108213533));
#57560=CARTESIAN_POINT('Ctrl Pts',(14.1561100063329,72.0131234493128,12.2523501508562));
#57561=CARTESIAN_POINT('Ctrl Pts',(14.1626863094704,72.080276432895,12.2746870134236));
#57562=CARTESIAN_POINT('Ctrl Pts',(14.1718438106433,72.1687837321241,12.3125776534399));
#57563=CARTESIAN_POINT('Ctrl Pts',(14.1742991986238,72.1920346943366,12.3233756953006));
#57564=CARTESIAN_POINT('Ctrl Pts',(14.1787329944899,72.2328957851856,12.343877344785));
#57565=CARTESIAN_POINT('Ctrl Pts',(14.1806991170041,72.2506325212958,12.353309818221));
#57566=CARTESIAN_POINT('Ctrl Pts',(14.1840219139556,72.2798553649482,12.3697513011343));
#57567=CARTESIAN_POINT('Ctrl Pts',(14.1853652962686,72.2914670310747,12.3765293086549));
#57568=CARTESIAN_POINT('Ctrl Pts',(14.1885093415771,72.3181556937138,12.3926816262207));
#57569=CARTESIAN_POINT('Ctrl Pts',(14.1903170640238,72.3331463424182,12.4021891777416));
#57570=CARTESIAN_POINT('Ctrl Pts',(14.1999026649965,72.4109359804507,12.4538432557881));
#57571=CARTESIAN_POINT('Ctrl Pts',(14.2078959440174,72.4700710441466,12.5012196510443));
#57572=CARTESIAN_POINT('Ctrl Pts',(14.2231252894692,72.5746573522342,12.6015610383273));
#57573=CARTESIAN_POINT('Ctrl Pts',(14.2303453761543,72.6206749140444,12.6535762450275));
#57574=CARTESIAN_POINT('Ctrl Pts',(14.2403516348131,72.6795543263118,12.7322590956993));
#57575=CARTESIAN_POINT('Ctrl Pts',(14.2432679300762,72.6960912186791,12.7560076203112));
#57576=CARTESIAN_POINT('Ctrl Pts',(14.2484630925337,72.7243694762793,12.7997312344215));
#57577=CARTESIAN_POINT('Ctrl Pts',(14.250751702894,72.7364024727295,12.8195008625732));
#57578=CARTESIAN_POINT('Ctrl Pts',(14.2558792756512,72.7623467479083,12.8648733801021));
#57579=CARTESIAN_POINT('Ctrl Pts',(14.258705844717,72.7759311862742,12.8906488022976));
#57580=CARTESIAN_POINT('Ctrl Pts',(14.2686398840895,72.8209087482662,12.9836093670273));
#57581=CARTESIAN_POINT('Ctrl Pts',(14.2755845575386,72.8472953411638,13.0530512168687));
#57582=CARTESIAN_POINT('Ctrl Pts',(14.28715814635,72.8808496167928,13.1717043784891));
#57583=CARTESIAN_POINT('Ctrl Pts',(14.2917711345339,72.8914669442238,13.2197353572991));
#57584=CARTESIAN_POINT('Ctrl Pts',(14.2978697489013,72.9016036510804,13.2827368088897));
#57585=CARTESIAN_POINT('Ctrl Pts',(14.299278560386,72.9036823773703,13.2972558893892));
#57586=CARTESIAN_POINT('Ctrl Pts',(14.3027574150405,72.9081629635459,13.3329466215874));
#57587=CARTESIAN_POINT('Ctrl Pts',(14.3048374149227,72.9102841614885,13.3541475287875));
#57588=CARTESIAN_POINT('Ctrl Pts',(14.3082685839507,72.9128682565807,13.3887386111822));
#57589=CARTESIAN_POINT('Ctrl Pts',(14.3096033497845,72.9136542410914,13.4021005592649));
#57590=CARTESIAN_POINT('Ctrl Pts',(14.3126726160277,72.9149641551614,13.4325819493954));
#57591=CARTESIAN_POINT('Ctrl Pts',(14.3144130745964,72.9153532090717,13.4497023981396));
#57592=CARTESIAN_POINT('Ctrl Pts',(14.3248101507675,72.9156070120017,13.5511864250937));
#57593=CARTESIAN_POINT('Ctrl Pts',(14.3337446112976,72.9074116815241,13.6353516107536));
#57594=CARTESIAN_POINT('Ctrl Pts',(14.3475118905944,72.8817789309105,13.7640485312999));
#57595=CARTESIAN_POINT('Ctrl Pts',(14.3523974580923,72.8700830549755,13.8094845992648));
#57596=CARTESIAN_POINT('Ctrl Pts',(14.3609273465335,72.8449901256348,13.88855013499));
#57597=CARTESIAN_POINT('Ctrl Pts',(14.3645946079188,72.8326199289611,13.9224490717668));
#57598=CARTESIAN_POINT('Ctrl Pts',(14.3706134829778,72.8096907104379,13.9778355819002));
#57599=CARTESIAN_POINT('Ctrl Pts',(14.37298948397,72.7999391051427,13.9996314606053));
#57600=CARTESIAN_POINT('Ctrl Pts',(14.3778780368709,72.7784425396652,14.0442586614366));
#57601=CARTESIAN_POINT('Ctrl Pts',(14.3803863398905,72.7666081996359,14.0670350094066));
#57602=CARTESIAN_POINT('Ctrl Pts',(14.3877972090109,72.7293203403296,14.1337739436212));
#57603=CARTESIAN_POINT('Ctrl Pts',(14.3926311014853,72.7019105305642,14.176587453146));
#57604=CARTESIAN_POINT('Ctrl Pts',(14.4043910868289,72.6285931422274,14.2772604595145));
#57605=CARTESIAN_POINT('Ctrl Pts',(14.4112487358363,72.5800728314809,14.3329738710421));
#57606=CARTESIAN_POINT('Ctrl Pts',(14.4207331854241,72.5082585172442,14.4022300067908));
#57607=CARTESIAN_POINT('Ctrl Pts',(14.4232252252988,72.4889717219042,14.4197179130659));
#57608=CARTESIAN_POINT('Ctrl Pts',(14.4277150060949,72.4537204885764,14.4497600036826));
#57609=CARTESIAN_POINT('Ctrl Pts',(14.42969994994,72.4379662802958,14.4625473282464));
#57610=CARTESIAN_POINT('Ctrl Pts',(14.4330455211469,72.4112423228979,14.4831966366446));
#57611=CARTESIAN_POINT('Ctrl Pts',(14.4343924570854,72.4004415118038,14.4912708527554));
#57612=CARTESIAN_POINT('Ctrl Pts',(14.4375382312067,72.3751393129469,14.5095648985649));
#57613=CARTESIAN_POINT('Ctrl Pts',(14.4393440192259,72.3605499510892,14.5196547398217));
#57614=CARTESIAN_POINT('Ctrl Pts',(14.4450144134697,72.314454345255,14.550126941652));
#57615=CARTESIAN_POINT('Ctrl Pts',(14.4489252220712,72.2822548807986,14.5694194668465));
#57616=CARTESIAN_POINT('Ctrl Pts',(14.4606935507246,72.183510131956,14.6227888442584));
#57617=CARTESIAN_POINT('Ctrl Pts',(14.4685870075198,72.1147529250637,14.6524526405009));
#57618=CARTESIAN_POINT('Ctrl Pts',(14.4786179771461,72.0229660970368,14.6827755300108));
#57619=CARTESIAN_POINT('Ctrl Pts',(14.4808805828867,72.0019732119006,14.6891129198592));
#57620=CARTESIAN_POINT('Ctrl Pts',(14.4865726092809,71.9484246744597,14.7037765500435));
#57621=CARTESIAN_POINT('Ctrl Pts',(14.4899797250469,71.9156811933941,14.7113609980156));
#57622=CARTESIAN_POINT('Ctrl Pts',(14.4957087608353,71.8595260038556,14.7220403916426));
#57623=CARTESIAN_POINT('Ctrl Pts',(14.4980497315057,71.8362607082174,14.7257975405665));
#57624=CARTESIAN_POINT('Ctrl Pts',(14.5029753891358,71.78670588571,14.732391005023));
#57625=CARTESIAN_POINT('Ctrl Pts',(14.505553845302,71.7604049151202,14.735058304044));
#57626=CARTESIAN_POINT('Ctrl Pts',(14.5132157729235,71.6813994141478,14.7405858389996));
#57627=CARTESIAN_POINT('Ctrl Pts',(14.5182254565731,71.6285779875919,14.7409848913599));
#57628=CARTESIAN_POINT('Ctrl Pts',(14.529824973741,71.5057116099575,14.7342489296445));
#57629=CARTESIAN_POINT('Ctrl Pts',(14.5363650344652,71.4359891878249,14.724585298081));
#57630=CARTESIAN_POINT('Ctrl Pts',(14.5454766825696,71.3425039421267,14.703615192929));
#57631=CARTESIAN_POINT('Ctrl Pts',(14.5479232462942,71.3177564210438,14.6972741822677));
#57632=CARTESIAN_POINT('Ctrl Pts',(14.5523417557301,71.2739797623426,14.6846390401184));
#57633=CARTESIAN_POINT('Ctrl Pts',(14.554301469331,71.2548763502391,14.6786323284445));
#57634=CARTESIAN_POINT('Ctrl Pts',(14.5576174455032,71.2231984630154,14.6678424829587));
#57635=CARTESIAN_POINT('Ctrl Pts',(14.5589605428977,71.2105438049429,14.6633066625323));
#57636=CARTESIAN_POINT('Ctrl Pts',(14.5621121806618,71.181275133035,14.6522884864969));
#57637=CARTESIAN_POINT('Ctrl Pts',(14.5639279465121,71.1647227730529,14.6456560898091));
#57638=CARTESIAN_POINT('Ctrl Pts',(14.5747662048084,71.0675590798907,14.6043287054158));
#57639=CARTESIAN_POINT('Ctrl Pts',(14.5840732617276,70.9905855644922,14.5617040993972));
#57640=CARTESIAN_POINT('Ctrl Pts',(14.5985102655584,70.8775755894171,14.482843207685));
#57641=CARTESIAN_POINT('Ctrl Pts',(14.6037099770511,70.8382498734026,14.4517920767621));
#57642=CARTESIAN_POINT('Ctrl Pts',(14.6120892722629,70.777065610681,14.3973133377009));
#57643=CARTESIAN_POINT('Ctrl Pts',(14.6153132949853,70.7540788900329,14.3752412753103));
#57644=CARTESIAN_POINT('Ctrl Pts',(14.6208409854466,70.7157045775444,14.335513026184));
#57645=CARTESIAN_POINT('Ctrl Pts',(14.6231601180174,70.6999311093351,14.3182541683687));
#57646=CARTESIAN_POINT('Ctrl Pts',(14.6254746131335,70.6845474582352,14.3004591583989));
#57647=CARTESIAN_POINT('Ctrl Pts',(14.6254887977793,70.6844531914697,14.3003500779552));
#57648=CARTESIAN_POINT('Ctrl Pts',(14.625502981677,70.6843589433682,14.3002409815638));
#57649=CARTESIAN_POINT('',(13.939,71.5396994937916,12.2044063041452));
#57650=CARTESIAN_POINT('Origin',(13.939,71.6454,13.47));
#57651=CARTESIAN_POINT('Ctrl Pts',(13.939,71.5396994937916,12.2044063041452));
#57652=CARTESIAN_POINT('Ctrl Pts',(13.9400008803869,71.5497265306615,12.2035688609149));
#57653=CARTESIAN_POINT('Ctrl Pts',(13.9409965869167,71.5597636455021,12.2028505703803));
#57654=CARTESIAN_POINT('Ctrl Pts',(13.9432202349612,71.5822983601624,12.2015069062696));
#57655=CARTESIAN_POINT('Ctrl Pts',(13.9444455907093,71.5947989547552,12.2009467657048));
#57656=CARTESIAN_POINT('Ctrl Pts',(13.9506098604098,71.6580160501178,12.1990497182328));
#57657=CARTESIAN_POINT('Ctrl Pts',(13.9554545208499,71.7087770568631,12.200567738032));
#57658=CARTESIAN_POINT('Ctrl Pts',(13.9662009801399,71.8212239847597,12.2106947988583));
#57659=CARTESIAN_POINT('Ctrl Pts',(13.9720824475883,71.882636162236,12.2208074072765));
#57660=CARTESIAN_POINT('Ctrl Pts',(13.9817260512219,71.9802087958434,12.2443314486371));
#57661=CARTESIAN_POINT('Ctrl Pts',(13.9854258910078,72.0169316314597,12.2549592481323));
#57662=CARTESIAN_POINT('Ctrl Pts',(13.9917230728597,72.077750086069,12.2755754712658));
#57663=CARTESIAN_POINT('Ctrl Pts',(13.9942936017168,72.1021193940872,12.284679905866));
#57664=CARTESIAN_POINT('Ctrl Pts',(13.9998426320644,72.1536153711263,12.305742678006));
#57665=CARTESIAN_POINT('Ctrl Pts',(14.0028263940625,72.1806367620649,12.3179152654874));
#57666=CARTESIAN_POINT('Ctrl Pts',(14.0137538928216,72.2769737338574,12.3654337747251));
#57667=CARTESIAN_POINT('Ctrl Pts',(14.021863947909,72.3434172847856,12.406177269604));
#57668=CARTESIAN_POINT('Ctrl Pts',(14.036212249074,72.4523557827846,12.4875976380237));
#57669=CARTESIAN_POINT('Ctrl Pts',(14.0423891403232,72.4965542068884,12.5256330654351));
#57670=CARTESIAN_POINT('Ctrl Pts',(14.0510067894361,72.5550641423249,12.5834406702947));
#57671=CARTESIAN_POINT('Ctrl Pts',(14.053507207594,72.5716609151176,12.600795071267));
#57672=CARTESIAN_POINT('Ctrl Pts',(14.0579761760335,72.6007134927342,12.6329518170708));
#57673=CARTESIAN_POINT('Ctrl Pts',(14.0599528001752,72.6133422534691,12.6475880141916));
#57674=CARTESIAN_POINT('Ctrl Pts',(14.0631257389503,72.6332926317608,12.6718062465998));
#57675=CARTESIAN_POINT('Ctrl Pts',(14.0643351086155,72.6408199704038,12.6812134225529));
#57676=CARTESIAN_POINT('Ctrl Pts',(14.0672300116217,72.6586585761863,12.7041691858446));
#57677=CARTESIAN_POINT('Ctrl Pts',(14.0689063732077,72.6688335190671,12.7178206847786));
#57678=CARTESIAN_POINT('Ctrl Pts',(14.078504766024,72.7260097741151,12.7978423042603));
#57679=CARTESIAN_POINT('Ctrl Pts',(14.0860899837725,72.7668322900115,12.8684119441173));
#57680=CARTESIAN_POINT('Ctrl Pts',(14.0997941559012,72.8274880950476,13.0012270457913));
#57681=CARTESIAN_POINT('Ctrl Pts',(14.105872946104,72.8498137862941,13.0619974288209));
#57682=CARTESIAN_POINT('Ctrl Pts',(14.1147712391621,72.8749865554666,13.1509543112505));
#57683=CARTESIAN_POINT('Ctrl Pts',(14.1174706324221,72.8816765490075,13.1779498911137));
#57684=CARTESIAN_POINT('Ctrl Pts',(14.1223875197292,72.892126759165,13.2269568674093));
#57685=CARTESIAN_POINT('Ctrl Pts',(14.1245938427866,72.8962028054639,13.2488897171881));
#57686=CARTESIAN_POINT('Ctrl Pts',(14.1296011449077,72.9040695909924,13.2984534208844));
#57687=CARTESIAN_POINT('Ctrl Pts',(14.1324115332915,72.9075317672287,13.3261234877943));
#57688=CARTESIAN_POINT('Ctrl Pts',(14.1444616756825,72.9183506254904,13.4439556617656));
#57689=CARTESIAN_POINT('Ctrl Pts',(14.1539650803249,72.9169724666146,13.5346343529476));
#57690=CARTESIAN_POINT('Ctrl Pts',(14.1696416569437,72.8989361470008,13.6819139638364));
#57691=CARTESIAN_POINT('Ctrl Pts',(14.1757614372814,72.8879576214181,13.7389098685731));
#57692=CARTESIAN_POINT('Ctrl Pts',(14.1836996253696,72.868263149876,13.8133164786309));
#57693=CARTESIAN_POINT('Ctrl Pts',(14.185641568696,72.8629934675486,13.8315615894252));
#57694=CARTESIAN_POINT('Ctrl Pts',(14.1888797281759,72.853418461148,13.8621241638884));
#57695=CARTESIAN_POINT('Ctrl Pts',(14.190186696673,72.8493296742341,13.8745038336191));
#57696=CARTESIAN_POINT('Ctrl Pts',(14.193207982358,72.8393558708374,13.9032094224017));
#57697=CARTESIAN_POINT('Ctrl Pts',(14.1949142433418,72.8333257001578,13.9194815566024));
#57698=CARTESIAN_POINT('Ctrl Pts',(14.2044541483894,72.7974459037967,14.0105293213565));
#57699=CARTESIAN_POINT('Ctrl Pts',(14.2119715930869,72.7608672484061,14.0824698321661));
#57700=CARTESIAN_POINT('Ctrl Pts',(14.2258300667714,72.6817886474242,14.207084965997));
#57701=CARTESIAN_POINT('Ctrl Pts',(14.2321347133448,72.6414408122528,14.2607569624196));
#57702=CARTESIAN_POINT('Ctrl Pts',(14.2413760835527,72.5778898376136,14.3326701905974));
#57703=CARTESIAN_POINT('Ctrl Pts',(14.2441863162849,72.5579966393668,14.3536878558472));
#57704=CARTESIAN_POINT('Ctrl Pts',(14.2491069800615,72.5223217491232,14.3888891395435));
#57705=CARTESIAN_POINT('Ctrl Pts',(14.2512026364407,72.5068696091555,14.4033911213357));
#57706=CARTESIAN_POINT('Ctrl Pts',(14.2561982192381,72.4694811707387,14.436761107742));
#57707=CARTESIAN_POINT('Ctrl Pts',(14.2591108893377,72.4472497530191,14.4552783632821));
#57708=CARTESIAN_POINT('Ctrl Pts',(14.2685636822047,72.3738376899391,14.5122948091277));
#57709=CARTESIAN_POINT('Ctrl Pts',(14.2752077046584,72.320378634547,14.5476831949409));
#57710=CARTESIAN_POINT('Ctrl Pts',(14.2876182528634,72.216925635022,14.6054408468038));
#57711=CARTESIAN_POINT('Ctrl Pts',(14.2933541963639,72.1677019373563,14.6289082780757));
#57712=CARTESIAN_POINT('Ctrl Pts',(14.3014093983787,72.0958859899463,14.6576386417937));
#57713=CARTESIAN_POINT('Ctrl Pts',(14.3037785183152,72.0744220921676,14.6655598591436));
#57714=CARTESIAN_POINT('Ctrl Pts',(14.3080342100415,72.0351404441845,14.6788623640315));
#57715=CARTESIAN_POINT('Ctrl Pts',(14.3099276650795,72.0173959500412,14.6844401891772));
#57716=CARTESIAN_POINT('Ctrl Pts',(14.3131770104863,71.9864162551457,14.6934355267851));
#57717=CARTESIAN_POINT('Ctrl Pts',(14.3145411934125,71.9732384615798,14.6970324255393));
#57718=CARTESIAN_POINT('Ctrl Pts',(14.3175782115732,71.9435299424688,14.7046285430537));
#57719=CARTESIAN_POINT('Ctrl Pts',(14.3192451068933,71.926972523221,14.7085096355793));
#57720=CARTESIAN_POINT('Ctrl Pts',(14.3271482062558,71.8474837798943,14.7254652170998));
#57721=CARTESIAN_POINT('Ctrl Pts',(14.3331979919213,71.7836893620083,14.7340844309566));
#57722=CARTESIAN_POINT('Ctrl Pts',(14.3444979591608,71.6636846004003,14.7410989367819));
#57723=CARTESIAN_POINT('Ctrl Pts',(14.3497369986247,71.6077103466657,14.740671386377));
#57724=CARTESIAN_POINT('Ctrl Pts',(14.3568506587739,71.5331155157879,14.7351675053485));
#57725=CARTESIAN_POINT('Ctrl Pts',(14.3586543682143,71.5143165029657,14.7333580941724));
#57726=CARTESIAN_POINT('Ctrl Pts',(14.3634092330661,71.4651675094903,14.7275187235973));
#57727=CARTESIAN_POINT('Ctrl Pts',(14.3663757765885,71.4349129264901,14.7228096161121));
#57728=CARTESIAN_POINT('Ctrl Pts',(14.3716716545472,71.3818618108209,14.7125764566566));
#57729=CARTESIAN_POINT('Ctrl Pts',(14.373985987621,71.3589920675168,14.7075051295526));
#57730=CARTESIAN_POINT('Ctrl Pts',(14.3791448312527,71.3087960301523,14.6949083860453));
#57731=CARTESIAN_POINT('Ctrl Pts',(14.3819972942167,71.2815560669788,14.6870949260919));
#57732=CARTESIAN_POINT('Ctrl Pts',(14.3938257027312,71.1708725190663,14.6512991507506));
#57733=CARTESIAN_POINT('Ctrl Pts',(14.4030355071996,71.0902009327151,14.6155965882369));
#57734=CARTESIAN_POINT('Ctrl Pts',(14.4167055282893,70.9774699565543,14.5509861125811));
#57735=CARTESIAN_POINT('Ctrl Pts',(14.4211189102001,70.9421110317391,14.5283225226393));
#57736=CARTESIAN_POINT('Ctrl Pts',(14.4283525036214,70.8854675647898,14.4879216300232));
#57737=CARTESIAN_POINT('Ctrl Pts',(14.431198690521,70.8635233793001,14.4711648481963));
#57738=CARTESIAN_POINT('Ctrl Pts',(14.4354711688423,70.8309739097779,14.4445860537232));
#57739=CARTESIAN_POINT('Ctrl Pts',(14.4369258536208,70.8199623305819,14.4352774579565));
#57740=CARTESIAN_POINT('Ctrl Pts',(14.4398774101789,70.7977382021212,14.4158318144448));
#57741=CARTESIAN_POINT('Ctrl Pts',(14.4413729012027,70.78654333058,14.405678174897));
#57742=CARTESIAN_POINT('Ctrl Pts',(14.4460738804801,70.7516443729712,14.3728708181603));
#57743=CARTESIAN_POINT('Ctrl Pts',(14.4492324740128,70.7286325727925,14.3494958189013));
#57744=CARTESIAN_POINT('Ctrl Pts',(14.4534224657446,70.6990405148412,14.3170112305496));
#57745=CARTESIAN_POINT('Ctrl Pts',(14.4544813502127,70.6916433897297,14.3086730545474));
#57746=CARTESIAN_POINT('Ctrl Pts',(14.4555370852546,70.6843589127286,14.3002409460971));
#57747=CARTESIAN_POINT('Origin',(13.939,71.6454,13.47));
#57748=CARTESIAN_POINT('',(13.939,73.264582312878,14.0019995049462));
#57749=CARTESIAN_POINT('',(13.939,71.6454,15.17434));
#57750=CARTESIAN_POINT('Origin',(13.939,71.6454,13.47));
#57751=CARTESIAN_POINT('Ctrl Pts',(13.939,73.264582312878,14.0019995049462));
#57752=CARTESIAN_POINT('Ctrl Pts',(13.939,73.2646272474247,14.001763711796));
#57753=CARTESIAN_POINT('Ctrl Pts',(13.939,73.2646721268292,14.0015279088845));
#57754=CARTESIAN_POINT('Ctrl Pts',(13.939,73.2647169510781,14.0012920962225));
#57755=CARTESIAN_POINT('Ctrl Pts',(13.939,73.2768225083756,13.9376068419289));
#57756=CARTESIAN_POINT('Ctrl Pts',(13.939,73.2849096414707,13.8732097073678));
#57757=CARTESIAN_POINT('Ctrl Pts',(13.939,73.2890848141171,13.8084486550991));
#57758=CARTESIAN_POINT('Ctrl Pts',(13.939,73.2919053719335,13.7646990170269));
#57759=CARTESIAN_POINT('Ctrl Pts',(13.939,73.2929394569106,13.7207833483898));
#57760=CARTESIAN_POINT('Ctrl Pts',(13.939,73.2922072227446,13.6768133865707));
#57761=CARTESIAN_POINT('Ctrl Pts',(13.939,73.2919437584807,13.6609926093361));
#57762=CARTESIAN_POINT('Ctrl Pts',(13.939,73.2914514204789,13.6451624680941));
#57763=CARTESIAN_POINT('Ctrl Pts',(13.939,73.2907312164348,13.6293359597415));
#57764=CARTESIAN_POINT('Ctrl Pts',(13.939,73.2878331555803,13.5656509739393));
#57765=CARTESIAN_POINT('Ctrl Pts',(13.939,73.2812563477203,13.5021534078011));
#57766=CARTESIAN_POINT('Ctrl Pts',(13.939,73.2710875752043,13.4391836479786));
#57767=CARTESIAN_POINT('Ctrl Pts',(13.939,73.2642723599941,13.3969806717347));
#57768=CARTESIAN_POINT('Ctrl Pts',(13.939,73.2558426578812,13.3550150867301));
#57769=CARTESIAN_POINT('Ctrl Pts',(13.939,73.2458136086189,13.3133965701029));
#57770=CARTESIAN_POINT('Ctrl Pts',(13.939,73.2421720474416,13.298284831149));
#57771=CARTESIAN_POINT('Ctrl Pts',(13.939,73.2383195470336,13.2832189194597));
#57772=CARTESIAN_POINT('Ctrl Pts',(13.939,73.2342565785196,13.2682043412823));
#57773=CARTESIAN_POINT('Ctrl Pts',(13.939,73.2311876368406,13.2568631594338));
#57774=CARTESIAN_POINT('Ctrl Pts',(13.939,73.2279985968259,13.2455515851929));
#57775=CARTESIAN_POINT('Ctrl Pts',(13.939,73.2246937617167,13.2342850968275));
#57776=CARTESIAN_POINT('Ctrl Pts',(13.939,73.2073554594815,13.1751772218635));
#57777=CARTESIAN_POINT('Ctrl Pts',(13.939,73.1868086540449,13.1172137677125));
#57778=CARTESIAN_POINT('Ctrl Pts',(13.939,73.1631328660133,13.0607036923316));
#57779=CARTESIAN_POINT('Ctrl Pts',(13.939,73.1400618824897,13.0056371823474));
#57780=CARTESIAN_POINT('Ctrl Pts',(13.939,73.1140190789678,12.9519500056349));
#57781=CARTESIAN_POINT('Ctrl Pts',(13.939,73.0850424472804,12.8999613856181));
#57782=CARTESIAN_POINT('Ctrl Pts',(13.939,73.0669043859958,12.867418860105));
#57783=CARTESIAN_POINT('Ctrl Pts',(13.939,73.0476161236673,12.8355425667648));
#57784=CARTESIAN_POINT('Ctrl Pts',(13.939,73.027181258192,12.804419590393));
#57785=CARTESIAN_POINT('Ctrl Pts',(13.939,73.0087993152631,12.776423282997));
#57786=CARTESIAN_POINT('Ctrl Pts',(13.939,72.989489497977,12.7490365884417));
#57787=CARTESIAN_POINT('Ctrl Pts',(13.939,72.9692519295121,12.7223284864005));
#57788=CARTESIAN_POINT('Ctrl Pts',(13.939,72.9625477153461,12.7134807418526));
#57789=CARTESIAN_POINT('Ctrl Pts',(13.939,72.9557464912283,12.7047139507404));
#57790=CARTESIAN_POINT('Ctrl Pts',(13.939,72.9488522064473,12.6960346929813));
#57791=CARTESIAN_POINT('Ctrl Pts',(13.939,72.9134703517828,12.6514922572707));
#57792=CARTESIAN_POINT('Ctrl Pts',(13.939,72.8756104083326,12.6092130013336));
#57793=CARTESIAN_POINT('Ctrl Pts',(13.939,72.8353120313341,12.5694808059632));
#57794=CARTESIAN_POINT('Ctrl Pts',(13.939,72.827878568635,12.5621517814655));
#57795=CARTESIAN_POINT('Ctrl Pts',(13.939,72.8203620597672,12.5549095428167));
#57796=CARTESIAN_POINT('Ctrl Pts',(13.939,72.8127626542197,12.547756041847));
#57797=CARTESIAN_POINT('Ctrl Pts',(13.939,72.7704332554513,12.5079103732296));
#57798=CARTESIAN_POINT('Ctrl Pts',(13.939,72.7255327909401,12.4708137762423));
#57799=CARTESIAN_POINT('Ctrl Pts',(13.939,72.6783705863321,12.4365867468974));
#57800=CARTESIAN_POINT('Ctrl Pts',(13.939,72.6372143500213,12.4067184292553));
#57801=CARTESIAN_POINT('Ctrl Pts',(13.939,72.5943349481246,12.3790360565908));
#57802=CARTESIAN_POINT('Ctrl Pts',(13.939,72.5499374525507,12.3536521712294));
#57803=CARTESIAN_POINT('Ctrl Pts',(13.939,72.5412850963492,12.3487052611597));
#57804=CARTESIAN_POINT('Ctrl Pts',(13.939,72.5325771207947,12.3438469827975));
#57805=CARTESIAN_POINT('Ctrl Pts',(13.939,72.5238247169746,12.3390831285424));
#57806=CARTESIAN_POINT('Ctrl Pts',(13.939,72.4744815389255,12.3122260829191));
#57807=CARTESIAN_POINT('Ctrl Pts',(13.939,72.4236416082651,12.2883166978516));
#57808=CARTESIAN_POINT('Ctrl Pts',(13.939,72.3715973046636,12.2674409134596));
#57809=CARTESIAN_POINT('Ctrl Pts',(13.939,72.3205033306167,12.2469463211196));
#57810=CARTESIAN_POINT('Ctrl Pts',(13.939,72.2682474285401,12.2293756434533));
#57811=CARTESIAN_POINT('Ctrl Pts',(13.939,72.2151072058468,12.2148592018594));
#57812=CARTESIAN_POINT('Ctrl Pts',(13.939,72.1624130772386,12.2004646208525));
#57813=CARTESIAN_POINT('Ctrl Pts',(13.939,72.1088484048521,12.1890732539501));
#57814=CARTESIAN_POINT('Ctrl Pts',(13.939,72.054700628375,12.1808599598466));
#57815=CARTESIAN_POINT('Ctrl Pts',(13.939,72.0424424009615,12.1790005958342));
#57816=CARTESIAN_POINT('Ctrl Pts',(13.939,72.0301516559131,12.1773041064647));
#57817=CARTESIAN_POINT('Ctrl Pts',(13.939,72.0178560360339,12.1757754217218));
#57818=CARTESIAN_POINT('Ctrl Pts',(13.939,71.964717139225,12.1691687909376));
#57819=CARTESIAN_POINT('Ctrl Pts',(13.939,71.9113917654875,12.1656763501367));
#57820=CARTESIAN_POINT('Ctrl Pts',(13.939,71.8581433977227,12.1654083282307));
#57821=CARTESIAN_POINT('Ctrl Pts',(13.939,71.8048950299579,12.1651403063247));
#57822=CARTESIAN_POINT('Ctrl Pts',(13.939,71.7517225988644,12.1680967638079));
#57823=CARTESIAN_POINT('Ctrl Pts',(13.939,71.6989120037461,12.1744397176796));
#57824=CARTESIAN_POINT('Ctrl Pts',(13.939,71.649362220586,12.1803910232506));
#57825=CARTESIAN_POINT('Ctrl Pts',(13.939,71.6001304926346,12.1893240715038));
#57826=CARTESIAN_POINT('Ctrl Pts',(13.939,71.5514831449858,12.2014131145448));
#57827=CARTESIAN_POINT('Ctrl Pts',(13.939,71.5475513741415,12.2023901739172));
#57828=CARTESIAN_POINT('Ctrl Pts',(13.939,71.5436234399984,12.2033878695024));
#57829=CARTESIAN_POINT('Ctrl Pts',(13.939,71.5396994937916,12.2044063041452));
#57830=CARTESIAN_POINT('',(13.9383731125779,70.3876696333693,13.2861333242433));
#57831=CARTESIAN_POINT('Ctrl Pts',(13.939,70.3906268762381,13.2739275442987));
#57832=CARTESIAN_POINT('Ctrl Pts',(13.938791037526,70.3899833170529,13.2780460257359));
#57833=CARTESIAN_POINT('Ctrl Pts',(13.9385820750519,70.3893600348717,13.282167675683));
#57834=CARTESIAN_POINT('Ctrl Pts',(13.9383731125779,70.3887570599105,13.2862922943282));
#57835=CARTESIAN_POINT('Ctrl Pts',(13.939,70.3865728200509,13.2860385524592));
#57836=CARTESIAN_POINT('Ctrl Pts',(13.939,70.3847141156884,13.2916947947257));
#57837=CARTESIAN_POINT('Ctrl Pts',(13.939,70.3828997146351,13.2973636743118));
#57838=CARTESIAN_POINT('Ctrl Pts',(13.939,70.3811298896707,13.3030447680062));
#57839=CARTESIAN_POINT('Ctrl Pts',(13.939,70.3662097964106,13.3509378927181));
#57840=CARTESIAN_POINT('Ctrl Pts',(13.939,70.3544544690838,13.3996961009194));
#57841=CARTESIAN_POINT('Ctrl Pts',(13.939,70.3457112817141,13.449041204321));
#57842=CARTESIAN_POINT('Ctrl Pts',(13.939,70.3408256769823,13.4766147493539));
#57843=CARTESIAN_POINT('Ctrl Pts',(13.939,70.3368812979427,13.5043722152326));
#57844=CARTESIAN_POINT('Ctrl Pts',(13.939,70.333856942926,13.5322692423113));
#57845=CARTESIAN_POINT('Ctrl Pts',(13.939,70.3322585732646,13.5470128029982));
#57846=CARTESIAN_POINT('Ctrl Pts',(13.939,70.3309172432249,13.5617953885959));
#57847=CARTESIAN_POINT('Ctrl Pts',(13.939,70.3298302731433,13.5766107087285));
#57848=CARTESIAN_POINT('Ctrl Pts',(13.939,70.3288771678923,13.5896014613277));
#57849=CARTESIAN_POINT('Ctrl Pts',(13.939,70.3281203298447,13.6026083266247));
#57850=CARTESIAN_POINT('Ctrl Pts',(13.939,70.3275573847283,13.6156237951177));
#57851=CARTESIAN_POINT('Ctrl Pts',(13.939,70.3252516912663,13.6689321545626));
#57852=CARTESIAN_POINT('Ctrl Pts',(13.939,70.3261938157966,13.7223984126338));
#57853=CARTESIAN_POINT('Ctrl Pts',(13.939,70.3302344908111,13.7757255847281));
#57854=CARTESIAN_POINT('Ctrl Pts',(13.939,70.3325695397501,13.8065426032142));
#57855=CARTESIAN_POINT('Ctrl Pts',(13.939,70.3359402122064,13.8373137478591));
#57856=CARTESIAN_POINT('Ctrl Pts',(13.939,70.3403248092368,13.8679850719421));
#57857=CARTESIAN_POINT('Ctrl Pts',(13.939,70.3424557006452,13.8828911763162));
#57858=CARTESIAN_POINT('Ctrl Pts',(13.939,70.3448269839794,13.897777514839));
#57859=CARTESIAN_POINT('Ctrl Pts',(13.939,70.3474313892361,13.9126111345666));
#57860=CARTESIAN_POINT('Ctrl Pts',(13.939,70.3570334545961,13.9673005442813));
#57861=CARTESIAN_POINT('Ctrl Pts',(13.939,70.3698086876566,14.0213395656395));
#57862=CARTESIAN_POINT('Ctrl Pts',(13.939,70.3855940774027,14.0744222844327));
#57863=CARTESIAN_POINT('Ctrl Pts',(13.939,70.4017665627473,14.1288067187448));
#57864=CARTESIAN_POINT('Ctrl Pts',(13.939,70.42109845679,14.1821884755046));
#57865=CARTESIAN_POINT('Ctrl Pts',(13.939,70.4434662797082,14.2342555993515));
#57866=CARTESIAN_POINT('Ctrl Pts',(13.939,70.4574328955107,14.2667666540649));
#57867=CARTESIAN_POINT('Ctrl Pts',(13.939,70.4725842111556,14.2987654365004));
#57868=CARTESIAN_POINT('Ctrl Pts',(13.939,70.4889004546343,14.3301761874657));
#57869=CARTESIAN_POINT('Ctrl Pts',(13.939,70.4970056681847,14.3457797082568));
#57870=CARTESIAN_POINT('Ctrl Pts',(13.939,70.5053984703826,14.3612381077738));
#57871=CARTESIAN_POINT('Ctrl Pts',(13.939,70.5140771559869,14.3765419403879));
#57872=CARTESIAN_POINT('Ctrl Pts',(13.939,70.519061925058,14.385331989361));
#57873=CARTESIAN_POINT('Ctrl Pts',(13.939,70.5241422137917,14.3940730469123));
#57874=CARTESIAN_POINT('Ctrl Pts',(13.939,70.5293138507803,14.4027567437645));
#57875=CARTESIAN_POINT('Ctrl Pts',(13.939,70.5595344952892,14.4535002348824));
#57876=CARTESIAN_POINT('Ctrl Pts',(13.939,70.5927791867216,14.5021351404274));
#57877=CARTESIAN_POINT('Ctrl Pts',(13.939,70.6288939100955,14.5483354328417));
#57878=CARTESIAN_POINT('Ctrl Pts',(13.939,70.6410781382509,14.5639222863749));
#57879=CARTESIAN_POINT('Ctrl Pts',(13.939,70.6535894795825,14.5792320742092));
#57880=CARTESIAN_POINT('Ctrl Pts',(13.939,70.6664233505904,14.5942522878267));
#57881=CARTESIAN_POINT('Ctrl Pts',(13.939,70.7032143579353,14.6373109089695));
#57882=CARTESIAN_POINT('Ctrl Pts',(13.939,70.7426523252183,14.6779915147634));
#57883=CARTESIAN_POINT('Ctrl Pts',(13.939,70.7844391127293,14.7162612897989));
#57884=CARTESIAN_POINT('Ctrl Pts',(13.939,70.8065815217405,14.7365400683813));
#57885=CARTESIAN_POINT('Ctrl Pts',(13.939,70.8293842670646,14.7561415704296));
#57886=CARTESIAN_POINT('Ctrl Pts',(13.939,70.8528080216974,14.7750580958749));
#57887=CARTESIAN_POINT('Ctrl Pts',(13.939,70.8661058911497,14.7857971720737));
#57888=CARTESIAN_POINT('Ctrl Pts',(13.939,70.8796039668997,14.7963154462813));
#57889=CARTESIAN_POINT('Ctrl Pts',(13.939,70.8932954851338,14.8066111791164));
#57890=CARTESIAN_POINT('Ctrl Pts',(13.939,70.9051906076058,14.8155560602405));
#57891=CARTESIAN_POINT('Ctrl Pts',(13.939,70.9172363806852,14.8243360470071));
#57892=CARTESIAN_POINT('Ctrl Pts',(13.939,70.9294017561649,14.8329314829181));
#57893=CARTESIAN_POINT('Ctrl Pts',(13.939,70.9781285705973,14.8673593730641));
#57894=CARTESIAN_POINT('Ctrl Pts',(13.939,71.0288346774935,14.898879998854));
#57895=CARTESIAN_POINT('Ctrl Pts',(13.939,71.0811731191553,14.9274712503634));
#57896=CARTESIAN_POINT('Ctrl Pts',(13.939,71.1349695972786,14.9568589926711));
#57897=CARTESIAN_POINT('Ctrl Pts',(13.939,71.1904912389686,14.9831525457031));
#57898=CARTESIAN_POINT('Ctrl Pts',(13.939,71.2474094103809,15.0062985260324));
#57899=CARTESIAN_POINT('Ctrl Pts',(13.939,71.3043094664642,15.0294371396975));
#57900=CARTESIAN_POINT('Ctrl Pts',(13.939,71.362606078278,15.0494307474303));
#57901=CARTESIAN_POINT('Ctrl Pts',(13.939,71.4220064371697,15.0661879181898));
#57902=CARTESIAN_POINT('Ctrl Pts',(13.939,71.4337420948756,15.0694986123307));
#57903=CARTESIAN_POINT('Ctrl Pts',(13.939,71.4455209214723,15.0726828426826));
#57904=CARTESIAN_POINT('Ctrl Pts',(13.939,71.4573407739189,15.0757396982053));
#57905=CARTESIAN_POINT('Ctrl Pts',(13.939,71.4688100974538,15.0787058997842));
#57906=CARTESIAN_POINT('Ctrl Pts',(13.939,71.480309797296,15.0815499878697));
#57907=CARTESIAN_POINT('Ctrl Pts',(13.939,71.4918315190228,15.0842702463551));
#57908=CARTESIAN_POINT('Ctrl Pts',(13.939,71.5542915564786,15.0990169526999));
#57909=CARTESIAN_POINT('Ctrl Pts',(13.939,71.6174513748119,15.1101419723292));
#57910=CARTESIAN_POINT('Ctrl Pts',(13.939,71.6809583817784,15.1175988679018));
#57911=CARTESIAN_POINT('Ctrl Pts',(13.939,71.7446039751982,15.1250720360836));
#57912=CARTESIAN_POINT('Ctrl Pts',(13.939,71.8085992672762,15.1288616146105));
#57913=CARTESIAN_POINT('Ctrl Pts',(13.939,71.8726203928869,15.1288794736354));
#57914=CARTESIAN_POINT('Ctrl Pts',(13.939,71.936077962909,15.1288971754536));
#57915=CARTESIAN_POINT('Ctrl Pts',(13.939,71.9995619530363,15.1252097402554));
#57916=CARTESIAN_POINT('Ctrl Pts',(13.939,72.0627722128131,15.1176831531631));
#57917=CARTESIAN_POINT('Ctrl Pts',(13.939,72.0746764434834,15.1162656897763));
#57918=CARTESIAN_POINT('Ctrl Pts',(13.939,72.0865709835791,15.1147119119096));
#57919=CARTESIAN_POINT('Ctrl Pts',(13.939,72.0984538423728,15.1130207093982));
#57920=CARTESIAN_POINT('Origin',(13.939,71.6454,13.47));
#57921=CARTESIAN_POINT('Ctrl Pts',(20.0410482168728,70.5240746963012,14.0615191344664));
#57922=CARTESIAN_POINT('Ctrl Pts',(19.9995464051999,70.7184011759149,14.4298980863427));
#57923=CARTESIAN_POINT('Ctrl Pts',(19.9165427818541,71.4952528988591,14.9541982817824));
#57924=CARTESIAN_POINT('Ctrl Pts',(19.7920373468353,72.80183948703,14.4146995872025));
#57925=CARTESIAN_POINT('Ctrl Pts',(19.6675319118165,73.0706439666114,13.0280142869573));
#57926=CARTESIAN_POINT('Ctrl Pts',(19.5430264767976,72.0647777602789,12.0377159341111));
#57927=CARTESIAN_POINT('Ctrl Pts',(19.418521041779,70.6828821695164,12.3292652371603));
#57928=CARTESIAN_POINT('Ctrl Pts',(19.2940156067602,70.1629367914403,13.6421861630661));
#57929=CARTESIAN_POINT('Ctrl Pts',(19.1695101717414,70.969967751209,14.8008798288961));
#57930=CARTESIAN_POINT('Ctrl Pts',(19.0450047367226,72.3817240944507,14.7681945331265));
#57931=CARTESIAN_POINT('Ctrl Pts',(18.9204993017039,73.1342796795863,13.5733292463045));
#57932=CARTESIAN_POINT('Ctrl Pts',(18.7959938666851,72.5539885107806,12.2859722028927));
#57933=CARTESIAN_POINT('Ctrl Pts',(18.6714884316663,71.1603094218454,12.0585666918175));
#57934=CARTESIAN_POINT('Ctrl Pts',(18.5469829966475,70.2008934572389,13.094696140498));
#57935=CARTESIAN_POINT('Ctrl Pts',(18.4224775616288,70.5346156866825,14.4668010991402));
#57936=CARTESIAN_POINT('Ctrl Pts',(18.29797212661,71.8627267685966,14.9465579232634));
#57937=CARTESIAN_POINT('Ctrl Pts',(18.1734666915911,72.996283760724,14.1044815120698));
#57938=CARTESIAN_POINT('Ctrl Pts',(18.0489612565725,72.9205130945634,12.6944095214458));
#57939=CARTESIAN_POINT('Ctrl Pts',(17.9244558215537,71.7032452653328,11.9786556757229));
#57940=CARTESIAN_POINT('Ctrl Pts',(17.7999503865349,70.4341936928937,12.5979717898819));
#57941=CARTESIAN_POINT('Ctrl Pts',(17.6754449515162,70.249428994792,13.9979383523494));
#57942=CARTESIAN_POINT('Ctrl Pts',(17.5509395164974,71.3143548597143,14.9252879647334));
#57943=CARTESIAN_POINT('Ctrl Pts',(17.4264340814786,72.6756364317002,14.5498457460373));
#57944=CARTESIAN_POINT('Ctrl Pts',(17.3019286464598,73.114637581328,13.207712230478));
#57945=CARTESIAN_POINT('Ctrl Pts',(17.177423211441,72.2383590324684,12.1003819768889));
#57946=CARTESIAN_POINT('Ctrl Pts',(17.0529177764223,70.8312562074884,12.2191507571731));
#57947=CARTESIAN_POINT('Ctrl Pts',(16.9284123414035,70.1529849983377,13.4576952863166));
#57948=CARTESIAN_POINT('Ctrl Pts',(16.8039069063848,70.8107421999714,14.7072551476021));
#57949=CARTESIAN_POINT('Ctrl Pts',(16.6794014713659,72.2156954121601,14.8492088628255));
#57950=CARTESIAN_POINT('Ctrl Pts',(16.5548960363472,73.1101130998516,13.756477705172));
#57951=CARTESIAN_POINT('Ctrl Pts',(16.4303906013284,72.6933014657471,12.4072881560414));
#57952=CARTESIAN_POINT('Ctrl Pts',(16.3058851663097,71.3383954419374,12.0094514206671));
#57953=CARTESIAN_POINT('Ctrl Pts',(16.1813797312908,70.2583237181736,12.9191158869499));
#57954=CARTESIAN_POINT('Ctrl Pts',(16.0568742962721,70.4199798494693,14.3219386262802));
#57955=CARTESIAN_POINT('Ctrl Pts',(15.9323688612533,71.6786473483666,14.9620953750271));
#57956=CARTESIAN_POINT('Ctrl Pts',(15.8078634262346,72.9075512918229,14.2665097869431));
#57957=CARTESIAN_POINT('Ctrl Pts',(15.6833579912158,73.006561990935,12.857878884914));
#57958=CARTESIAN_POINT('Ctrl Pts',(15.558852556197,71.8870431132129,11.9972261450596));
#57959=CARTESIAN_POINT('Ctrl Pts',(15.4343471211782,70.5512033220584,12.4550193257908));
#57960=CARTESIAN_POINT('Ctrl Pts',(15.3098416861595,70.1948999249935,13.8214347519347));
#57961=CARTESIAN_POINT('Ctrl Pts',(15.1853362511407,71.1371063372083,14.8732435492854));
#57962=CARTESIAN_POINT('Ctrl Pts',(15.060830816122,72.5343350401052,14.6688469993707));
#57963=CARTESIAN_POINT('Ctrl Pts',(14.9363253811032,73.1357954317769,13.3912365894174));
#57964=CARTESIAN_POINT('Ctrl Pts',(14.8118199460844,72.4029999040765,12.1841181131174));
#57965=CARTESIAN_POINT('Ctrl Pts',(14.6873145110655,70.992063963973,12.1281739071278));
#57966=CARTESIAN_POINT('Ctrl Pts',(14.5628090760468,70.1658546328295,13.2733737564971));
#57967=CARTESIAN_POINT('Ctrl Pts',(14.4383036410281,70.6644547802432,14.5947496730614));
#57968=CARTESIAN_POINT('Ctrl Pts',(14.3137982060093,72.0405920319688,14.9089214685884));
#57969=CARTESIAN_POINT('Ctrl Pts',(14.1892927709905,73.064211602503,13.9355998645035));
#57970=CARTESIAN_POINT('Ctrl Pts',(14.0647765398672,72.8150660685469,12.5440178827245));
#57971=CARTESIAN_POINT('Ctrl Pts',(13.9817621204168,71.954707782371,12.1718579782255));
#57972=CARTESIAN_POINT('Ctrl Pts',(13.9402495126393,71.5395603852097,12.2066460152216));
#57973=CARTESIAN_POINT('Ctrl Pts',(19.9566236618974,70.3947393463692,14.1297458426261));
#57974=CARTESIAN_POINT('Ctrl Pts',(19.9151218502245,70.6114797349164,14.5406141778164));
#57975=CARTESIAN_POINT('Ctrl Pts',(19.8321182268787,71.4779347059999,15.1253879477157));
#57976=CARTESIAN_POINT('Ctrl Pts',(19.7076127918599,72.935224959771,14.5236626608872));
#57977=CARTESIAN_POINT('Ctrl Pts',(19.5831073568411,73.2350337530116,12.9770349889135));
#57978=CARTESIAN_POINT('Ctrl Pts',(19.4586019218224,72.1131494229894,11.8725141320536));
#57979=CARTESIAN_POINT('Ctrl Pts',(19.3340964868036,70.5718639128065,12.1976911709685));
#57980=CARTESIAN_POINT('Ctrl Pts',(19.2095910517848,69.9919472514666,13.6620463745321));
#57981=CARTESIAN_POINT('Ctrl Pts',(19.085085616766,70.8920623780184,14.954385513482));
#57982=CARTESIAN_POINT('Ctrl Pts',(18.9605801817473,72.4666528248602,14.9179302464542));
#57983=CARTESIAN_POINT('Ctrl Pts',(18.8360747467285,73.3060093049954,13.5852473972504));
#57984=CARTESIAN_POINT('Ctrl Pts',(18.7115693117097,72.6587864785055,12.1494046529026));
#57985=CARTESIAN_POINT('Ctrl Pts',(18.587063876691,71.1043583437171,11.8957698475678));
#57986=CARTESIAN_POINT('Ctrl Pts',(18.4625584416722,70.0342818962844,13.0514080279053));
#57987=CARTESIAN_POINT('Ctrl Pts',(18.3380530066534,70.4064961504623,14.5817736397085));
#57988=CARTESIAN_POINT('Ctrl Pts',(18.2135475716346,71.8877935655138,15.1168663387342));
#57989=CARTESIAN_POINT('Ctrl Pts',(18.0890421366159,73.152096728945,14.1776635655901));
#57990=CARTESIAN_POINT('Ctrl Pts',(17.9645367015971,73.0675865599923,12.6049517471346));
#57991=CARTESIAN_POINT('Ctrl Pts',(17.8400312665783,71.7099172253868,11.8066417744819));
#57992=CARTESIAN_POINT('Ctrl Pts',(17.7155258315596,70.2944913326127,12.4973907423177));
#57993=CARTESIAN_POINT('Ctrl Pts',(17.5910203965408,70.0884155958631,14.0588315573082));
#57994=CARTESIAN_POINT('Ctrl Pts',(17.466514961522,71.2761716144768,15.0931430711416));
#57995=CARTESIAN_POINT('Ctrl Pts',(17.3420095265032,72.7944654539002,14.674396781295));
#57996=CARTESIAN_POINT('Ctrl Pts',(17.2175040914845,73.284101657531,13.1774595639752));
#57997=CARTESIAN_POINT('Ctrl Pts',(17.0929986564657,72.3067518206332,11.9424081706189));
#57998=CARTESIAN_POINT('Ctrl Pts',(16.9684932214469,70.7373516358605,12.0748759209596));
#57999=CARTESIAN_POINT('Ctrl Pts',(16.8439877864282,69.9808476035539,13.456276042102));
#58000=CARTESIAN_POINT('Ctrl Pts',(16.7194823514094,70.7144715118097,14.8499620203914));
#58001=CARTESIAN_POINT('Ctrl Pts',(16.5949769163906,72.2814741442132,15.0082888909979));
#58002=CARTESIAN_POINT('Ctrl Pts',(16.4704714813718,73.2790553155443,13.7895204752976));
#58003=CARTESIAN_POINT('Ctrl Pts',(16.3459660463531,72.8141679995884,12.2847133708637));
#58004=CARTESIAN_POINT('Ctrl Pts',(16.2214606113343,71.3029850736735,11.8409895470452));
#58005=CARTESIAN_POINT('Ctrl Pts',(16.0969551763155,70.0983362500405,12.8555760833815));
#58006=CARTESIAN_POINT('Ctrl Pts',(15.9724497412967,70.278638043073,14.4202025109772));
#58007=CARTESIAN_POINT('Ctrl Pts',(15.847944306278,71.682482147618,15.1341959035932));
#58008=CARTESIAN_POINT('Ctrl Pts',(15.7234388712592,73.0531297233953,14.3583804258011));
#58009=CARTESIAN_POINT('Ctrl Pts',(15.5989334362404,73.1635604657141,12.7872759132704));
#58010=CARTESIAN_POINT('Ctrl Pts',(15.4744280012216,71.9149145939534,11.8273541897304));
#58011=CARTESIAN_POINT('Ctrl Pts',(15.3499225662029,70.4249970286936,12.3379499256443));
#58012=CARTESIAN_POINT('Ctrl Pts',(15.2254171311841,70.0275970609997,13.8619697656991));
#58013=CARTESIAN_POINT('Ctrl Pts',(15.1009116961653,71.07847898034,15.0350957744051));
#58014=CARTESIAN_POINT('Ctrl Pts',(14.9764062611466,72.636866146912,14.8071238184768));
#58015=CARTESIAN_POINT('Ctrl Pts',(14.8519008261278,73.3076998863273,13.3821518989748));
#58016=CARTESIAN_POINT('Ctrl Pts',(14.727395391109,72.4903826184226,12.0358025589579));
#58017=CARTESIAN_POINT('Ctrl Pts',(14.6028899560903,70.9167072012529,11.9734056639631));
#58018=CARTESIAN_POINT('Ctrl Pts',(14.4783845210715,69.9952016410777,13.2506945893318));
#58019=CARTESIAN_POINT('Ctrl Pts',(14.3538790860527,70.5513110806915,14.7244799949148));
#58020=CARTESIAN_POINT('Ctrl Pts',(14.2293736510339,72.0861740763376,15.0748888386734));
#58021=CARTESIAN_POINT('Ctrl Pts',(14.1048682160152,73.2278594703359,13.9893028543541));
#58022=CARTESIAN_POINT('Ctrl Pts',(13.9803519848918,72.9499771151273,12.4372137102212));
#58023=CARTESIAN_POINT('Ctrl Pts',(13.8973375654414,71.9903838079969,12.0221283216363));
#58024=CARTESIAN_POINT('Ctrl Pts',(13.8558249576639,71.5273526845803,12.0609288632316));
#58025=CARTESIAN_POINT('Ctrl Pts',(19.8721991069221,70.2654039964372,14.1979725507859));
#58026=CARTESIAN_POINT('Ctrl Pts',(19.8306972952492,70.5045582939178,14.6513302692902));
#58027=CARTESIAN_POINT('Ctrl Pts',(19.7476936719033,71.4606165131408,15.296577613649));
#58028=CARTESIAN_POINT('Ctrl Pts',(19.6231882368845,73.0686104325118,14.6326257345719));
#58029=CARTESIAN_POINT('Ctrl Pts',(19.4986828018657,73.3994235394119,12.9260556908696));
#58030=CARTESIAN_POINT('Ctrl Pts',(19.374177366847,72.1615210857001,11.707312329996));
#58031=CARTESIAN_POINT('Ctrl Pts',(19.2496719318282,70.4608456560965,12.0661171047766));
#58032=CARTESIAN_POINT('Ctrl Pts',(19.1251664968095,69.8209577114928,13.681906585998));
#58033=CARTESIAN_POINT('Ctrl Pts',(19.0006610617907,70.8141570048277,15.1078911980679));
#58034=CARTESIAN_POINT('Ctrl Pts',(18.8761556267719,72.5515815552696,15.0676659597819));
#58035=CARTESIAN_POINT('Ctrl Pts',(18.7516501917531,73.4777389304046,13.5971655481964));
#58036=CARTESIAN_POINT('Ctrl Pts',(18.6271447567344,72.7635844462302,12.0128371029124));
#58037=CARTESIAN_POINT('Ctrl Pts',(18.5026393217156,71.048407265589,11.7329730033181));
#58038=CARTESIAN_POINT('Ctrl Pts',(18.3781338866968,69.8676703353299,13.0081199153126));
#58039=CARTESIAN_POINT('Ctrl Pts',(18.253628451678,70.278376614242,14.696746180277));
#58040=CARTESIAN_POINT('Ctrl Pts',(18.1291230166593,71.912860362431,15.2871747542049));
#58041=CARTESIAN_POINT('Ctrl Pts',(18.0046175816405,73.3079096971661,14.2508456191104));
#58042=CARTESIAN_POINT('Ctrl Pts',(17.8801121466217,73.2146600254213,12.5154939728233));
#58043=CARTESIAN_POINT('Ctrl Pts',(17.7556067116029,71.7165891854406,11.6346278732409));
#58044=CARTESIAN_POINT('Ctrl Pts',(17.6311012765842,70.1547889723317,12.3968096947535));
#58045=CARTESIAN_POINT('Ctrl Pts',(17.5065958415654,69.9274021969343,14.119724762267));
#58046=CARTESIAN_POINT('Ctrl Pts',(17.3820904065466,71.2379883692392,15.2609981775499));
#58047=CARTESIAN_POINT('Ctrl Pts',(17.2575849715279,72.9132944761003,14.7989478165527));
#58048=CARTESIAN_POINT('Ctrl Pts',(17.1330795365091,73.4535657337339,13.1472068974724));
#58049=CARTESIAN_POINT('Ctrl Pts',(17.0085741014903,72.375144608798,11.7844343643487));
#58050=CARTESIAN_POINT('Ctrl Pts',(16.8840686664715,70.6434470642325,11.9306010847461));
#58051=CARTESIAN_POINT('Ctrl Pts',(16.7595632314528,69.8087102087702,13.4548567978873));
#58052=CARTESIAN_POINT('Ctrl Pts',(16.635057796434,70.618200823648,14.9926688931807));
#58053=CARTESIAN_POINT('Ctrl Pts',(16.5105523614152,72.3472528762663,15.1673689191704));
#58054=CARTESIAN_POINT('Ctrl Pts',(16.3860469263965,73.4479975312372,13.8225632454232));
#58055=CARTESIAN_POINT('Ctrl Pts',(16.2615414913777,72.9350345334297,12.1621385856859));
#58056=CARTESIAN_POINT('Ctrl Pts',(16.1370360563589,71.2675747054093,11.6725276734234));
#58057=CARTESIAN_POINT('Ctrl Pts',(16.0125306213401,69.9383487819074,12.7920362798131));
#58058=CARTESIAN_POINT('Ctrl Pts',(15.8880251863214,70.1372962366768,14.5184663956743));
#58059=CARTESIAN_POINT('Ctrl Pts',(15.7635197513026,71.6863169468695,15.3062964321592));
#58060=CARTESIAN_POINT('Ctrl Pts',(15.6390143162838,73.1987081549679,14.4502510646592));
#58061=CARTESIAN_POINT('Ctrl Pts',(15.514508881265,73.3205589404931,12.7166729416266));
#58062=CARTESIAN_POINT('Ctrl Pts',(15.3900034462463,71.9427860746941,11.6574822344012));
#58063=CARTESIAN_POINT('Ctrl Pts',(15.2654980112275,70.2987907353288,12.2208805254978));
#58064=CARTESIAN_POINT('Ctrl Pts',(15.1409925762087,69.8602941970061,13.9025047794634));
#58065=CARTESIAN_POINT('Ctrl Pts',(15.01648714119,71.0198516234718,15.1969479995249));
#58066=CARTESIAN_POINT('Ctrl Pts',(14.8919817061712,72.7393972537189,14.9454006375828));
#58067=CARTESIAN_POINT('Ctrl Pts',(14.7674762711524,73.4796043408778,13.3730672085322));
#58068=CARTESIAN_POINT('Ctrl Pts',(14.6429708361336,72.5777653327687,11.8874870047984));
#58069=CARTESIAN_POINT('Ctrl Pts',(14.5184654011149,70.841350438533,11.8186374207984));
#58070=CARTESIAN_POINT('Ctrl Pts',(14.3939599660961,69.8245486493257,13.2280154221665));
#58071=CARTESIAN_POINT('Ctrl Pts',(14.2694545310773,70.4381673811397,14.8542103167684));
#58072=CARTESIAN_POINT('Ctrl Pts',(14.1449490960586,72.1317561207064,15.2408562087582));
#58073=CARTESIAN_POINT('Ctrl Pts',(14.0204436610398,73.3915073381686,14.0430058442048));
#58074=CARTESIAN_POINT('Ctrl Pts',(13.8959274299164,73.0848881617078,12.3304095377178));
#58075=CARTESIAN_POINT('Ctrl Pts',(13.8129130104661,72.0260598336227,11.872398665047));
#58076=CARTESIAN_POINT('Ctrl Pts',(13.7714004026886,71.5151449839512,11.9152117112416));
#58077=CARTESIAN_POINT('Ctrl Pts',(19.7877745519467,70.1360686465052,14.2661992589458));
#58078=CARTESIAN_POINT('Ctrl Pts',(19.7462727402738,70.3976368529192,14.762046360764));
#58079=CARTESIAN_POINT('Ctrl Pts',(19.6632691169279,71.4432983202816,15.4677672795824));
#58080=CARTESIAN_POINT('Ctrl Pts',(19.5387636819092,73.2019959052528,14.7415888082566));
#58081=CARTESIAN_POINT('Ctrl Pts',(19.4142582468904,73.5638133258121,12.8750763928258));
#58082=CARTESIAN_POINT('Ctrl Pts',(19.2897528118716,72.2098927484105,11.5421105279385));
#58083=CARTESIAN_POINT('Ctrl Pts',(19.1652473768528,70.3498273993866,11.9345430385847));
#58084=CARTESIAN_POINT('Ctrl Pts',(19.0407419418341,69.649968171519,13.701766797464));
#58085=CARTESIAN_POINT('Ctrl Pts',(18.9162365068153,70.7362516316372,15.2613968826537));
#58086=CARTESIAN_POINT('Ctrl Pts',(18.7917310717965,72.636510285679,15.2174016731096));
#58087=CARTESIAN_POINT('Ctrl Pts',(18.6672256367778,73.6494685558138,13.6090836991424));
#58088=CARTESIAN_POINT('Ctrl Pts',(18.542720201759,72.868382413955,11.8762695529223));
#58089=CARTESIAN_POINT('Ctrl Pts',(18.4182147667402,70.9924561874607,11.5701761590684));
#58090=CARTESIAN_POINT('Ctrl Pts',(18.2937093317214,69.7010587743754,12.9648318027199));
#58091=CARTESIAN_POINT('Ctrl Pts',(18.1692038967027,70.1502570780218,14.8117187208453));
#58092=CARTESIAN_POINT('Ctrl Pts',(18.0446984616839,71.9379271593483,15.4574831696756));
#58093=CARTESIAN_POINT('Ctrl Pts',(17.9201930266651,73.4637226653873,14.3240276726307));
#58094=CARTESIAN_POINT('Ctrl Pts',(17.7956875916463,73.3617334908503,12.4260361985122));
#58095=CARTESIAN_POINT('Ctrl Pts',(17.6711821566276,71.7232611454946,11.4626139719998));
#58096=CARTESIAN_POINT('Ctrl Pts',(17.5466767216088,70.0150866120508,12.2962286471894));
#58097=CARTESIAN_POINT('Ctrl Pts',(17.42217128659,69.7663887980055,14.1806179672258));
#58098=CARTESIAN_POINT('Ctrl Pts',(17.2976658515713,71.1998051240017,15.4288532839581));
#58099=CARTESIAN_POINT('Ctrl Pts',(17.1731604165525,73.0321234983004,14.9234988518104));
#58100=CARTESIAN_POINT('Ctrl Pts',(17.0486549815337,73.6230298099368,13.1169542309696));
#58101=CARTESIAN_POINT('Ctrl Pts',(16.9241495465149,72.4435373969628,11.6264605580787));
#58102=CARTESIAN_POINT('Ctrl Pts',(16.7996441114962,70.5495424926045,11.7863262485325));
#58103=CARTESIAN_POINT('Ctrl Pts',(16.6751386764774,69.6365728139866,13.4534375536726));
#58104=CARTESIAN_POINT('Ctrl Pts',(16.5506332414586,70.5219301354863,15.1353757659699));
#58105=CARTESIAN_POINT('Ctrl Pts',(16.4261278064399,72.4130316083195,15.3264489473428));
#58106=CARTESIAN_POINT('Ctrl Pts',(16.3016223714211,73.61693974693,13.8556060155489));
#58107=CARTESIAN_POINT('Ctrl Pts',(16.1771169364023,73.0559010672711,12.0395638005081));
#58108=CARTESIAN_POINT('Ctrl Pts',(16.0526115013835,71.2321643371453,11.5040657998015));
#58109=CARTESIAN_POINT('Ctrl Pts',(15.9281060663648,69.7783613137743,12.7284964762447));
#58110=CARTESIAN_POINT('Ctrl Pts',(15.803600631346,69.9959544302804,14.6167302803713));
#58111=CARTESIAN_POINT('Ctrl Pts',(15.6790951963272,71.690151746121,15.4783969607253));
#58112=CARTESIAN_POINT('Ctrl Pts',(15.5545897613085,73.3442865865404,14.5421217035174));
#58113=CARTESIAN_POINT('Ctrl Pts',(15.4300843262897,73.477557415272,12.646069969983));
#58114=CARTESIAN_POINT('Ctrl Pts',(15.3055788912709,71.9706575554347,11.487610279072));
#58115=CARTESIAN_POINT('Ctrl Pts',(15.1810734562521,70.172584441964,12.1038111253513));
#58116=CARTESIAN_POINT('Ctrl Pts',(15.0565680212334,69.6929913330123,13.9430397932278));
#58117=CARTESIAN_POINT('Ctrl Pts',(14.9320625862146,70.9612242666035,15.3588002246446));
#58118=CARTESIAN_POINT('Ctrl Pts',(14.8075571511958,72.8419283605258,15.0836774566888));
#58119=CARTESIAN_POINT('Ctrl Pts',(14.6830517161771,73.6515087954282,13.3639825180896));
#58120=CARTESIAN_POINT('Ctrl Pts',(14.5585462811583,72.6651480471149,11.7391714506388));
#58121=CARTESIAN_POINT('Ctrl Pts',(14.4340408461395,70.7659936758129,11.6638691776337));
#58122=CARTESIAN_POINT('Ctrl Pts',(14.3095354111207,69.6538956575739,13.2053362550011));
#58123=CARTESIAN_POINT('Ctrl Pts',(14.185029976102,70.3250236815881,14.9839406386219));
#58124=CARTESIAN_POINT('Ctrl Pts',(14.0605245410832,72.1773381650751,15.4068235788432));
#58125=CARTESIAN_POINT('Ctrl Pts',(13.9360191060644,73.5551552060015,14.0967088340556));
#58126=CARTESIAN_POINT('Ctrl Pts',(13.811502874941,73.2197992082883,12.2236053652145));
#58127=CARTESIAN_POINT('Ctrl Pts',(13.7284884554907,72.0617358592485,11.7226690084578));
#58128=CARTESIAN_POINT('Ctrl Pts',(13.6869758477133,71.5029372833219,11.7694945592516));
#58129=CARTESIAN_POINT('Ctrl Pts',(13.939,73.2573116306334,14.0236386281943));
#58130=CARTESIAN_POINT('Ctrl Pts',(13.939,73.2597351913816,14.0164255871116));
#58131=CARTESIAN_POINT('Ctrl Pts',(13.939,73.2621587521298,14.0092125460289));
#58132=CARTESIAN_POINT('Ctrl Pts',(13.939,73.264582312878,14.0019995049462));
#58133=CARTESIAN_POINT('',(19.7896276022603,72.6408167039313,14.2604548813054));
#58134=CARTESIAN_POINT('Ctrl Pts',(19.789,72.641620209933,14.2612225008607));
#58135=CARTESIAN_POINT('Ctrl Pts',(19.789,72.6387719444729,14.266450811799));
#58136=CARTESIAN_POINT('Ctrl Pts',(19.7890000000001,72.6358841274372,14.2716554974063));
#58137=CARTESIAN_POINT('Ctrl Pts',(19.789,72.6329568803625,14.2768360690663));
#58138=CARTESIAN_POINT('Ctrl Pts',(19.789,72.6082794067475,14.3205096699577));
#58139=CARTESIAN_POINT('Ctrl Pts',(19.789,72.5808040359192,14.3624698284424));
#58140=CARTESIAN_POINT('Ctrl Pts',(19.789,72.5508379984757,14.4026372192824));
#58141=CARTESIAN_POINT('Ctrl Pts',(19.789,72.5340932826451,14.4250823472557));
#58142=CARTESIAN_POINT('Ctrl Pts',(19.789,72.516569904339,14.4469676385987));
#58143=CARTESIAN_POINT('Ctrl Pts',(19.789,72.4983147064114,14.4682781592601));
#58144=CARTESIAN_POINT('Ctrl Pts',(19.789,72.4886668022326,14.4795408068717));
#58145=CARTESIAN_POINT('Ctrl Pts',(19.789,72.4788144131649,14.4906428946705));
#58146=CARTESIAN_POINT('Ctrl Pts',(19.789,72.4687639579593,14.5015820667859));
#58147=CARTESIAN_POINT('Ctrl Pts',(19.789,72.4599513410421,14.5111739440961));
#58148=CARTESIAN_POINT('Ctrl Pts',(19.789,72.4509925607107,14.5206338520356));
#58149=CARTESIAN_POINT('Ctrl Pts',(19.789,72.4418947144233,14.5299583775618));
#58150=CARTESIAN_POINT('Ctrl Pts',(19.789,72.4045912780145,14.5681912553245));
#58151=CARTESIAN_POINT('Ctrl Pts',(19.789,72.3649432494347,14.6041609037284));
#58152=CARTESIAN_POINT('Ctrl Pts',(19.789,72.3232702684491,14.637772358608));
#58153=CARTESIAN_POINT('Ctrl Pts',(19.789,72.2992595261045,14.657138287415));
#58154=CARTESIAN_POINT('Ctrl Pts',(19.789,72.274575549839,14.6757211293625));
#58155=CARTESIAN_POINT('Ctrl Pts',(19.789,72.2492721984787,14.6934998632628));
#58156=CARTESIAN_POINT('Ctrl Pts',(19.789,72.2369517511987,14.7021565012948));
#58157=CARTESIAN_POINT('Ctrl Pts',(19.789,72.2244810608313,14.7106244461823));
#58158=CARTESIAN_POINT('Ctrl Pts',(19.789,72.2118891168812,14.7188864255039));
#58159=CARTESIAN_POINT('Ctrl Pts',(19.789,72.1656012648316,14.7492573736266));
#58160=CARTESIAN_POINT('Ctrl Pts',(19.789,72.1176239693264,14.7768870422043));
#58161=CARTESIAN_POINT('Ctrl Pts',(19.789,72.0682888938632,14.801685512822));
#58162=CARTESIAN_POINT('Ctrl Pts',(19.789,72.0175949058287,14.8271670462132));
#58163=CARTESIAN_POINT('Ctrl Pts',(19.789,71.965466663248,14.8496601676798));
#58164=CARTESIAN_POINT('Ctrl Pts',(19.789,71.9122161490832,14.8690412852909));
#58165=CARTESIAN_POINT('Ctrl Pts',(19.789,71.878811941916,14.881199118468));
#58166=CARTESIAN_POINT('Ctrl Pts',(19.789,71.8449651868027,14.892131784855));
#58167=CARTESIAN_POINT('Ctrl Pts',(19.789,71.8107455960956,14.9018012949587));
#58168=CARTESIAN_POINT('Ctrl Pts',(19.789,71.7938250741778,14.9065825665714));
#58169=CARTESIAN_POINT('Ctrl Pts',(19.789,71.7768133199693,14.9110548975236));
#58170=CARTESIAN_POINT('Ctrl Pts',(19.789,71.7597183837639,14.9152130609202));
#58171=CARTESIAN_POINT('Ctrl Pts',(19.789,71.7498995878967,14.9176013797231));
#58172=CARTESIAN_POINT('Ctrl Pts',(19.789,71.7400510664113,14.9198865455108));
#58173=CARTESIAN_POINT('Ctrl Pts',(19.789,71.7301817745093,14.9220658655007));
#58174=CARTESIAN_POINT('Ctrl Pts',(19.789,71.6725102077602,14.9348008012503));
#58175=CARTESIAN_POINT('Ctrl Pts',(19.789,71.6143038238963,14.9438881407692));
#58176=CARTESIAN_POINT('Ctrl Pts',(19.789,71.5559056616475,14.9492168055038));
#58177=CARTESIAN_POINT('Ctrl Pts',(19.789,71.5362035607306,14.9510145656783));
#58178=CARTESIAN_POINT('Ctrl Pts',(19.789,71.5164792954917,14.9523842178932));
#58179=CARTESIAN_POINT('Ctrl Pts',(19.789,71.4967451192257,14.9533205346688));
#58180=CARTESIAN_POINT('Ctrl Pts',(19.789,71.4401728765432,14.9560046872345));
#58181=CARTESIAN_POINT('Ctrl Pts',(19.789,71.3835204002696,14.9551314660335));
#58182=CARTESIAN_POINT('Ctrl Pts',(19.789,71.3270157996704,14.9508956287317));
#58183=CARTESIAN_POINT('Ctrl Pts',(19.789,71.2970745678256,14.9486511002267));
#58184=CARTESIAN_POINT('Ctrl Pts',(19.789,71.2671745497408,14.945461559463));
#58185=CARTESIAN_POINT('Ctrl Pts',(19.789,71.2373482913903,14.9413503873858));
#58186=CARTESIAN_POINT('Ctrl Pts',(19.789,71.2204156653886,14.9390164392789));
#58187=CARTESIAN_POINT('Ctrl Pts',(19.789,71.2035067992762,14.9363853860378));
#58188=CARTESIAN_POINT('Ctrl Pts',(19.789,71.1866275930246,14.9334609646543));
#58189=CARTESIAN_POINT('Ctrl Pts',(19.789,71.1719630215258,14.9309202417179));
#58190=CARTESIAN_POINT('Ctrl Pts',(19.789,71.1573154150842,14.928156812882));
#58191=CARTESIAN_POINT('Ctrl Pts',(19.789,71.1427203611893,14.9251798379043));
#58192=CARTESIAN_POINT('Ctrl Pts',(19.789,71.084427289372,14.9132897128372));
#58193=CARTESIAN_POINT('Ctrl Pts',(19.789,71.0268925829723,14.8979855977678));
#58194=CARTESIAN_POINT('Ctrl Pts',(19.789,70.9703678600636,14.8795032122604));
#58195=CARTESIAN_POINT('Ctrl Pts',(19.789,70.9120325610004,14.8604288067527));
#58196=CARTESIAN_POINT('Ctrl Pts',(19.789,70.8547720822423,14.8379693077407));
#58197=CARTESIAN_POINT('Ctrl Pts',(19.789,70.7988513813129,14.812328463574));
#58198=CARTESIAN_POINT('Ctrl Pts',(19.789,70.7429306803836,14.7866876194072));
#58199=CARTESIAN_POINT('Ctrl Pts',(19.789,70.6883487124932,14.7578651502859));
#58200=CARTESIAN_POINT('Ctrl Pts',(19.789,70.6353738709878,14.7260125179742));
#58201=CARTESIAN_POINT('Ctrl Pts',(19.789,70.6249237878694,14.7197291078547));
#58202=CARTESIAN_POINT('Ctrl Pts',(19.789,70.614536282974,14.7133276283047));
#58203=CARTESIAN_POINT('Ctrl Pts',(19.789,70.6042134878844,14.7068090168181));
#58204=CARTESIAN_POINT('Ctrl Pts',(19.789,70.5941967736294,14.7004836884516));
#58205=CARTESIAN_POINT('Ctrl Pts',(19.789,70.5842482301542,14.6940525900351));
#58206=CARTESIAN_POINT('Ctrl Pts',(19.789,70.5743748300446,14.6875206335784));
#58207=CARTESIAN_POINT('Ctrl Pts',(19.789,70.5206424546419,14.6519728453245));
#58208=CARTESIAN_POINT('Ctrl Pts',(19.789,70.4690864887003,14.6134113895555));
#58209=CARTESIAN_POINT('Ctrl Pts',(19.789,70.419985490651,14.5720639021248));
#58210=CARTESIAN_POINT('Ctrl Pts',(19.789,70.3709118097536,14.5307394182099));
#58211=CARTESIAN_POINT('Ctrl Pts',(19.789,70.324289270061,14.4866316356991));
#58212=CARTESIAN_POINT('Ctrl Pts',(19.789,70.2804049653145,14.4399165596753));
#58213=CARTESIAN_POINT('Ctrl Pts',(19.789,70.2371769561625,14.3939001138058));
#58214=CARTESIAN_POINT('Ctrl Pts',(19.789,70.1966048791055,14.3453533038319));
#58215=CARTESIAN_POINT('Ctrl Pts',(19.789,70.1589874472662,14.294401015779));
#58216=CARTESIAN_POINT('Ctrl Pts',(19.789,70.1518669431078,14.2847563919645));
#58217=CARTESIAN_POINT('Ctrl Pts',(19.789,70.1448523993543,14.275025465843));
#58218=CARTESIAN_POINT('Ctrl Pts',(19.789,70.1379459883857,14.2652089275579));
#58219=CARTESIAN_POINT('Ctrl Pts',(19.7896276022603,72.6399620111973,14.2597761745477));
#58220=CARTESIAN_POINT('Ctrl Pts',(19.7894184015068,72.6425467167479,14.2565212650763));
#58221=CARTESIAN_POINT('Ctrl Pts',(19.7892092007534,72.6451154436252,14.2532536670299));
#58222=CARTESIAN_POINT('Ctrl Pts',(19.789,72.647668068024,14.249973537897));
#58223=CARTESIAN_POINT('Origin',(19.789,71.6454,13.47));
#58224=CARTESIAN_POINT('',(19.789,70.1487787364881,12.6545862220908));
#58225=CARTESIAN_POINT('',(19.789,71.6454,15.17434));
#58226=CARTESIAN_POINT('Origin',(19.789,71.6454,13.47));
#58227=CARTESIAN_POINT('Ctrl Pts',(19.789,70.1487787364881,12.6545862220908));
#58228=CARTESIAN_POINT('Ctrl Pts',(19.789,70.1489198244377,12.6543919049109));
#58229=CARTESIAN_POINT('Ctrl Pts',(19.789,70.1490609573038,12.6541976212514));
#58230=CARTESIAN_POINT('Ctrl Pts',(19.789,70.149202135088,12.6540033711292));
#58231=CARTESIAN_POINT('Ctrl Pts',(19.789,70.1879762118368,12.6006531277364));
#58232=CARTESIAN_POINT('Ctrl Pts',(19.789,70.2301358263451,12.5498286668655));
#58233=CARTESIAN_POINT('Ctrl Pts',(19.789,70.2753374488553,12.5016996841948));
#58234=CARTESIAN_POINT('Ctrl Pts',(19.789,70.3045799803949,12.4705633396221));
#58235=CARTESIAN_POINT('Ctrl Pts',(19.789,70.3350964259176,12.4405560547994));
#58236=CARTESIAN_POINT('Ctrl Pts',(19.789,70.3667987628524,12.4117351475176));
#58237=CARTESIAN_POINT('Ctrl Pts',(19.789,70.3785067074331,12.401091339589));
#58238=CARTESIAN_POINT('Ctrl Pts',(19.789,70.3903782324118,12.3906078824228));
#58239=CARTESIAN_POINT('Ctrl Pts',(19.789,70.4024031776679,12.3802929434665));
#58240=CARTESIAN_POINT('Ctrl Pts',(19.789,70.4508048825224,12.3387741988632));
#58241=CARTESIAN_POINT('Ctrl Pts',(19.789,70.5015910097002,12.3000658874002));
#58242=CARTESIAN_POINT('Ctrl Pts',(19.789,70.5544538397869,12.2643380655472));
#58243=CARTESIAN_POINT('Ctrl Pts',(19.789,70.5898575003643,12.2404101813234));
#58244=CARTESIAN_POINT('Ctrl Pts',(19.789,70.6261931205748,12.2178201212625));
#58245=CARTESIAN_POINT('Ctrl Pts',(19.789,70.6633705338864,12.1966318922625));
#58246=CARTESIAN_POINT('Ctrl Pts',(19.789,70.67687546201,12.1889351354356));
#58247=CARTESIAN_POINT('Ctrl Pts',(19.789,70.690491471705,12.1814234606844));
#58248=CARTESIAN_POINT('Ctrl Pts',(19.789,70.7042142283386,12.174100295955));
#58249=CARTESIAN_POINT('Ctrl Pts',(19.789,70.7145797303758,12.1685687339702));
#58250=CARTESIAN_POINT('Ctrl Pts',(19.789,70.7250059162256,12.1631449583535));
#58251=CARTESIAN_POINT('Ctrl Pts',(19.789,70.7354785604031,12.157836434949));
#58252=CARTESIAN_POINT('Ctrl Pts',(19.789,70.7903722896243,12.1300111177326));
#58253=CARTESIAN_POINT('Ctrl Pts',(19.789,70.8466272484881,12.1053018562078));
#58254=CARTESIAN_POINT('Ctrl Pts',(19.789,70.903964603326,12.0838618819254));
#58255=CARTESIAN_POINT('Ctrl Pts',(19.789,70.9598880709669,12.0629505979745));
#58256=CARTESIAN_POINT('Ctrl Pts',(19.789,71.0168421988663,12.0451493184059));
#58257=CARTESIAN_POINT('Ctrl Pts',(19.789,71.0745683658387,12.0306489624154));
#58258=CARTESIAN_POINT('Ctrl Pts',(19.789,71.1107541019409,12.0215593920736));
#58259=CARTESIAN_POINT('Ctrl Pts',(19.789,71.147243151667,12.0137678679056));
#58260=CARTESIAN_POINT('Ctrl Pts',(19.789,71.183969313623,12.0073316554369));
#58261=CARTESIAN_POINT('Ctrl Pts',(19.789,71.2169581642735,12.0015504019494));
#58262=CARTESIAN_POINT('Ctrl Pts',(19.789,71.2501383400913,11.9968627522112));
#58263=CARTESIAN_POINT('Ctrl Pts',(19.789,71.2834594960917,11.9933158611134));
#58264=CARTESIAN_POINT('Ctrl Pts',(19.789,71.2944980578517,11.9921408545669));
#58265=CARTESIAN_POINT('Ctrl Pts',(19.789,71.3055440776528,11.9910919794509));
#58266=CARTESIAN_POINT('Ctrl Pts',(19.789,71.3165900557996,11.9901708649002));
#58267=CARTESIAN_POINT('Ctrl Pts',(19.789,71.373278300547,11.9854436812687));
#58268=CARTESIAN_POINT('Ctrl Pts',(19.789,71.4300147845701,11.9840721766392));
#58269=CARTESIAN_POINT('Ctrl Pts',(19.789,71.4865655032522,11.9862218894224));
#58270=CARTESIAN_POINT('Ctrl Pts',(19.789,71.4969969079928,11.9866184276918));
#58271=CARTESIAN_POINT('Ctrl Pts',(19.789,71.5074219568044,11.9871349167772));
#58272=CARTESIAN_POINT('Ctrl Pts',(19.789,71.5178391251249,11.9877725845906));
#58273=CARTESIAN_POINT('Ctrl Pts',(19.789,71.5747021515476,11.9912533502463));
#58274=CARTESIAN_POINT('Ctrl Pts',(19.789,71.6313325553251,11.998341595826));
#58275=CARTESIAN_POINT('Ctrl Pts',(19.789,71.6874486199552,12.0089024886782));
#58276=CARTESIAN_POINT('Ctrl Pts',(19.789,71.7385648764786,12.0185224310549));
#58277=CARTESIAN_POINT('Ctrl Pts',(19.789,71.789254587842,12.0310247112241));
#58278=CARTESIAN_POINT('Ctrl Pts',(19.789,71.8392799419038,12.0463316703637));
#58279=CARTESIAN_POINT('Ctrl Pts',(19.789,71.8488104716665,12.0492478602117));
#58280=CARTESIAN_POINT('Ctrl Pts',(19.789,71.8583145157961,12.0522652805629));
#58281=CARTESIAN_POINT('Ctrl Pts',(19.789,71.8677801889141,12.055379744509));
#58282=CARTESIAN_POINT('Ctrl Pts',(19.789,71.9211107347488,12.0729269448148));
#58283=CARTESIAN_POINT('Ctrl Pts',(19.789,71.9733200814847,12.0935796656819));
#58284=CARTESIAN_POINT('Ctrl Pts',(19.789,72.024145868163,12.1171840112806));
#58285=CARTESIAN_POINT('Ctrl Pts',(19.789,72.0745282756665,12.1405824441733));
#58286=CARTESIAN_POINT('Ctrl Pts',(19.789,72.1235519535232,12.1668820916441));
#58287=CARTESIAN_POINT('Ctrl Pts',(19.789,72.1709238057524,12.1959669353727));
#58288=CARTESIAN_POINT('Ctrl Pts',(19.789,72.2170798876667,12.2243053339456));
#58289=CARTESIAN_POINT('Ctrl Pts',(19.789,72.2616683576994,12.2552886122479));
#58290=CARTESIAN_POINT('Ctrl Pts',(19.789,72.3043729294909,12.288829428407));
#58291=CARTESIAN_POINT('Ctrl Pts',(19.789,72.3141234565815,12.2964876397619));
#58292=CARTESIAN_POINT('Ctrl Pts',(19.789,72.3237775801607,12.304281098163));
#58293=CARTESIAN_POINT('Ctrl Pts',(19.789,72.3333127754152,12.3121930388631));
#58294=CARTESIAN_POINT('Ctrl Pts',(19.789,72.3739413221764,12.3459050546245));
#58295=CARTESIAN_POINT('Ctrl Pts',(19.789,72.4124882882934,12.3818224635262));
#58296=CARTESIAN_POINT('Ctrl Pts',(19.789,72.4487040921249,12.4198334708158));
#58297=CARTESIAN_POINT('Ctrl Pts',(19.789,72.4859547374258,12.4589306162682));
#58298=CARTESIAN_POINT('Ctrl Pts',(19.789,72.5207400586359,12.5002434669381));
#58299=CARTESIAN_POINT('Ctrl Pts',(19.789,72.5527331601959,12.5436703974697));
#58300=CARTESIAN_POINT('Ctrl Pts',(19.789,72.5823338904573,12.5838499610027));
#58301=CARTESIAN_POINT('Ctrl Pts',(19.789,72.6095441962068,12.6258399981718));
#58302=CARTESIAN_POINT('Ctrl Pts',(19.789,72.63405470443,12.6695658026545));
#58303=CARTESIAN_POINT('Ctrl Pts',(19.789,72.6360356770569,12.673099781672));
#58304=CARTESIAN_POINT('Ctrl Pts',(19.789,72.6379989859775,12.6766450988997));
#58305=CARTESIAN_POINT('Ctrl Pts',(19.789,72.6399444526778,12.6802017145829));
#58306=CARTESIAN_POINT('Origin',(19.789,71.6454,13.47));
#58307=CARTESIAN_POINT('Ctrl Pts',(20.040973809758,72.9819445553179,12.4091675667597));
#58308=CARTESIAN_POINT('Ctrl Pts',(19.999461202279,72.633355430368,11.9699615052754));
#58309=CARTESIAN_POINT('Ctrl Pts',(19.9164467831271,71.4752515269709,11.4692823470277));
#58310=CARTESIAN_POINT('Ctrl Pts',(19.7919305523022,69.8808452508188,12.5077823363638));
#58311=CARTESIAN_POINT('Ctrl Pts',(19.6674251172834,69.8699348774273,14.4089112278554));
#58312=CARTESIAN_POINT('Ctrl Pts',(19.5429196822646,71.4466435928667,15.4688729946812));
#58313=CARTESIAN_POINT('Ctrl Pts',(19.4184142472458,73.202158953221,14.7397343798463));
#58314=CARTESIAN_POINT('Ctrl Pts',(19.2939088122271,73.563614891359,12.8737593469291));
#58315=CARTESIAN_POINT('Ctrl Pts',(19.1694033772083,72.2080713563702,11.5416219660584));
#58316=CARTESIAN_POINT('Ctrl Pts',(19.0448979421895,70.3487144949671,11.9357554795025));
#58317=CARTESIAN_POINT('Ctrl Pts',(18.9203925071708,69.6502169789121,13.7033818367937));
#58318=CARTESIAN_POINT('Ctrl Pts',(18.795887072152,70.7378073584978,15.2620730044683));
#58319=CARTESIAN_POINT('Ctrl Pts',(18.6713816371332,72.6378980052588,15.2164825479556));
#58320=CARTESIAN_POINT('Ctrl Pts',(18.5468762021145,73.6494862177602,13.6074171356146));
#58321=CARTESIAN_POINT('Ctrl Pts',(18.4223707670957,72.8669944998988,11.8753352416511));
#58322=CARTESIAN_POINT('Ctrl Pts',(18.2978653320769,70.9909148234652,11.5708164984104));
#58323=CARTESIAN_POINT('Ctrl Pts',(18.1733598970581,69.7007390850565,12.9664706197299));
#58324=CARTESIAN_POINT('Ctrl Pts',(18.0488544620394,70.1514475657618,14.8128903622671));
#58325=CARTESIAN_POINT('Ctrl Pts',(17.9243490270206,71.9395609525946,15.4571380645241));
#58326=CARTESIAN_POINT('Ctrl Pts',(17.7998435920018,73.4643377264577,14.3224751075195));
#58327=CARTESIAN_POINT('Ctrl Pts',(17.675338156983,73.3607789380809,12.4246658804603));
#58328=CARTESIAN_POINT('Ctrl Pts',(17.5508327219643,71.7215916392195,11.4626527092184));
#58329=CARTESIAN_POINT('Ctrl Pts',(17.4263272869455,70.0141966499276,12.2976417212453));
#58330=CARTESIAN_POINT('Ctrl Pts',(17.3018218519267,69.7670751170318,14.1821403964886));
#58331=CARTESIAN_POINT('Ctrl Pts',(17.177316416908,71.2014533072286,15.4291221611814));
#58332=CARTESIAN_POINT('Ctrl Pts',(17.0528109818892,73.0332580794223,14.9222734795421));
#58333=CARTESIAN_POINT('Ctrl Pts',(16.9283055468704,73.6226350938871,13.1153315752696));
#58334=CARTESIAN_POINT('Ctrl Pts',(16.8038001118517,72.4419667407709,11.6258932417151));
#58335=CARTESIAN_POINT('Ctrl Pts',(16.6792946768329,70.5482019652493,11.7873221393186));
#58336=CARTESIAN_POINT('Ctrl Pts',(16.5547892418141,69.6366624746966,13.4551051186589));
#58337=CARTESIAN_POINT('Ctrl Pts',(16.4302838067953,70.5233697144127,15.1362221790386));
#58338=CARTESIAN_POINT('Ctrl Pts',(16.3057783717766,72.4145323853567,15.3257164914074));
#58339=CARTESIAN_POINT('Ctrl Pts',(16.1812729367578,73.6171581900668,13.853950389472));
#58340=CARTESIAN_POINT('Ctrl Pts',(16.056767501739,73.0546416597839,12.0384671509735));
#58341=CARTESIAN_POINT('Ctrl Pts',(15.9322620667202,71.2305544421676,11.5045098412908));
#58342=CARTESIAN_POINT('Ctrl Pts',(15.8077566317015,69.7778422804962,12.7300837376931));
#58343=CARTESIAN_POINT('Ctrl Pts',(15.6832511966827,69.9969905948197,14.6180397431827));
#58344=CARTESIAN_POINT('Ctrl Pts',(15.5587457616639,71.6918161520591,15.4782565459948));
#58345=CARTESIAN_POINT('Ctrl Pts',(15.4342403266452,73.345087948424,14.5406567682313));
#58346=CARTESIAN_POINT('Ctrl Pts',(15.3097348916264,73.476780975954,12.6445926450108));
#58347=CARTESIAN_POINT('Ctrl Pts',(15.1852294566076,71.9689930174075,11.4874416489449));
#58348=CARTESIAN_POINT('Ctrl Pts',(15.0607240215888,70.1715328997075,12.1051050809465));
#58349=CARTESIAN_POINT('Ctrl Pts',(14.9362185865701,69.6934717153363,13.9446319828763));
#58350=CARTESIAN_POINT('Ctrl Pts',(14.8117131515513,70.9628523308878,15.3592775276433));
#58351=CARTESIAN_POINT('Ctrl Pts',(14.6872077165325,72.8431530960336,15.0825876121152));
#58352=CARTESIAN_POINT('Ctrl Pts',(14.5627022815138,73.6514248701469,13.3623521753633));
#58353=CARTESIAN_POINT('Ctrl Pts',(14.438196846495,72.6634403331674,11.7383559146618));
#58354=CARTESIAN_POINT('Ctrl Pts',(14.3136914114762,70.7649881924949,11.6648114379736));
#58355=CARTESIAN_POINT('Ctrl Pts',(14.1891859764574,69.6528597290574,13.2067518969809));
#58356=CARTESIAN_POINT('Ctrl Pts',(14.0646805414387,70.3282556438409,14.9854666458723));
#58357=CARTESIAN_POINT('Ctrl Pts',(13.9816769180928,71.5585834209095,15.2639982872471));
#58358=CARTESIAN_POINT('Ctrl Pts',(13.9401751064199,72.0989948849057,15.1149828251624));
#58359=CARTESIAN_POINT('Ctrl Pts',(19.9565660471403,72.8674323206533,12.5000573856227));
#58360=CARTESIAN_POINT('Ctrl Pts',(19.9150534396612,72.5487095548299,12.0984815455766));
#58361=CARTESIAN_POINT('Ctrl Pts',(19.8320390205094,71.4898294785953,11.6406994901849));
#58362=CARTESIAN_POINT('Ctrl Pts',(19.7075227896845,70.0320284693002,12.5902230559481));
#58363=CARTESIAN_POINT('Ctrl Pts',(19.5830173546657,70.0220528730047,14.3284673530698));
#58364=CARTESIAN_POINT('Ctrl Pts',(19.458511919647,71.4636726101519,15.2976138978402));
#58365=CARTESIAN_POINT('Ctrl Pts',(19.3340064846282,73.0687792272267,14.6309462959114));
#58366=CARTESIAN_POINT('Ctrl Pts',(19.2095010496094,73.3992664056296,12.9248439511118));
#58367=CARTESIAN_POINT('Ctrl Pts',(19.0849956145907,72.1598628966198,11.706841207771));
#58368=CARTESIAN_POINT('Ctrl Pts',(18.9604901795719,70.459811692773,12.0672062178001));
#58369=CARTESIAN_POINT('Ctrl Pts',(18.8359847445531,69.82115992683,13.6833861878982));
#58370=CARTESIAN_POINT('Ctrl Pts',(18.7114793095343,70.8155679248255,15.1085320816407));
#58371=CARTESIAN_POINT('Ctrl Pts',(18.5869738745156,72.5528629317702,15.0668477164242));
#58372=CARTESIAN_POINT('Ctrl Pts',(18.4624684394968,73.4777804632882,13.5956435338909));
#58373=CARTESIAN_POINT('Ctrl Pts',(18.337963004478,72.7623309363231,12.0119626547013));
#58374=CARTESIAN_POINT('Ctrl Pts',(18.2134575694592,71.0469896919175,11.7335344159986));
#58375=CARTESIAN_POINT('Ctrl Pts',(18.0889521344405,69.8673534086486,13.0096119234183));
#58376=CARTESIAN_POINT('Ctrl Pts',(17.9644466994217,70.2794461656189,14.6978344326455));
#58377=CARTESIAN_POINT('Ctrl Pts',(17.8399412644029,71.9143578810632,15.2868843910119));
#58378=CARTESIAN_POINT('Ctrl Pts',(17.7154358293842,73.3084950925974,14.2494368917941));
#58379=CARTESIAN_POINT('Ctrl Pts',(17.5909303943654,73.2138089962899,12.5142278374661));
#58380=CARTESIAN_POINT('Ctrl Pts',(17.4664249593466,71.7150637050516,11.6346378653441));
#58381=CARTESIAN_POINT('Ctrl Pts',(17.3419195243278,70.1539546101586,12.3980868323294));
#58382=CARTESIAN_POINT('Ctrl Pts',(17.2174140893091,69.9280059134793,14.121125754012));
#58383=CARTESIAN_POINT('Ctrl Pts',(17.0929086542903,71.2394896956594,15.2612688294198));
#58384=CARTESIAN_POINT('Ctrl Pts',(16.9684032192715,72.9143494134601,14.7978458420012));
#58385=CARTESIAN_POINT('Ctrl Pts',(16.8438977842528,73.4532298853908,13.1457187955978));
#58386=CARTESIAN_POINT('Ctrl Pts',(16.719392349234,72.3737186324814,11.7838923035579));
#58387=CARTESIAN_POINT('Ctrl Pts',(16.5948869142152,70.6422075098673,11.9314903238213));
#58388=CARTESIAN_POINT('Ctrl Pts',(16.4703814791964,69.8087667430968,13.4563812797421));
#58389=CARTESIAN_POINT('Ctrl Pts',(16.3458760441777,70.6195028323494,14.9934638815989));
#58390=CARTESIAN_POINT('Ctrl Pts',(16.2213706091589,72.3486347930544,15.1667227328458));
#58391=CARTESIAN_POINT('Ctrl Pts',(16.0968651741401,73.4482222307946,13.8210543540021));
#58392=CARTESIAN_POINT('Ctrl Pts',(15.9723597391213,72.9339008950991,12.1611177763384));
#58393=CARTESIAN_POINT('Ctrl Pts',(15.8478543041026,71.2660975085615,11.6729087692499));
#58394=CARTESIAN_POINT('Ctrl Pts',(15.7233488690838,69.9378505697632,12.7934781560268));
#58395=CARTESIAN_POINT('Ctrl Pts',(15.598843434065,70.1382227324828,14.5196781914091));
#58396=CARTESIAN_POINT('Ctrl Pts',(15.4743379990463,71.6878393169617,15.3061934868572));
#58397=CARTESIAN_POINT('Ctrl Pts',(15.3498325640275,73.1994623765476,14.4489252216837));
#58398=CARTESIAN_POINT('Ctrl Pts',(15.2253271290087,73.3198722315023,12.7153117544878));
#58399=CARTESIAN_POINT('Ctrl Pts',(15.1008216939899,71.9412682704863,11.6573029425538));
#58400=CARTESIAN_POINT('Ctrl Pts',(14.9763162589712,70.2978106317753,12.222046313202));
#58401=CARTESIAN_POINT('Ctrl Pts',(14.8518108239524,69.8607086913822,13.9039665454345));
#58402=CARTESIAN_POINT('Ctrl Pts',(14.7273053889336,71.0213315327552,15.197408332388));
#58403=CARTESIAN_POINT('Ctrl Pts',(14.6027999539149,72.7405322121599,14.9444246078808));
#58404=CARTESIAN_POINT('Ctrl Pts',(14.4782945188961,73.4795530161492,13.3715752071784));
#58405=CARTESIAN_POINT('Ctrl Pts',(14.3537890838773,72.5762168484989,11.8867194189437));
#58406=CARTESIAN_POINT('Ctrl Pts',(14.2292836488585,70.8404199639996,11.8194760732872));
#58407=CARTESIAN_POINT('Ctrl Pts',(14.1047782138398,69.8235762518826,13.2293064227002));
#58408=CARTESIAN_POINT('Ctrl Pts',(13.980272778821,70.4411057115768,14.8556247550891));
#58409=CARTESIAN_POINT('Ctrl Pts',(13.8972691554751,71.5660216768494,15.1102924103725));
#58410=CARTESIAN_POINT('Ctrl Pts',(13.8557673438022,72.0601318603277,14.9740442694332));
#58411=CARTESIAN_POINT('Ctrl Pts',(19.8721582845226,72.7529200859888,12.5909472044855));
#58412=CARTESIAN_POINT('Ctrl Pts',(19.8306456770436,72.4640636792919,12.2270015858779));
#58413=CARTESIAN_POINT('Ctrl Pts',(19.7476312578916,71.5044074302198,11.812116633342));
#58414=CARTESIAN_POINT('Ctrl Pts',(19.6231150270668,70.1832116877817,12.6726637755322));
#58415=CARTESIAN_POINT('Ctrl Pts',(19.4986095920481,70.1741708685821,14.2480234782843));
#58416=CARTESIAN_POINT('Ctrl Pts',(19.3741041570293,71.4807016274368,15.126354800999));
#58417=CARTESIAN_POINT('Ctrl Pts',(19.2495987220105,72.9353995012324,14.5221582119765));
#58418=CARTESIAN_POINT('Ctrl Pts',(19.1250932869917,73.2349179199001,12.9759285552946));
#58419=CARTESIAN_POINT('Ctrl Pts',(19.000587851973,72.1116544368694,11.8720604494837));
#58420=CARTESIAN_POINT('Ctrl Pts',(18.8760824169542,70.5709088905788,12.1986569560976));
#58421=CARTESIAN_POINT('Ctrl Pts',(18.7515769819354,69.9921028747479,13.6633905390027));
#58422=CARTESIAN_POINT('Ctrl Pts',(18.6270715469167,70.8933284911529,14.9549911588131));
#58423=CARTESIAN_POINT('Ctrl Pts',(18.5025661118979,72.4678278582817,14.917212884893));
#58424=CARTESIAN_POINT('Ctrl Pts',(18.3780606768791,73.3060747088162,13.583869932167));
#58425=CARTESIAN_POINT('Ctrl Pts',(18.2535552418603,72.6576673727473,12.1485900677515));
#58426=CARTESIAN_POINT('Ctrl Pts',(18.1290498068416,71.1030645603695,11.8962523335869));
#58427=CARTESIAN_POINT('Ctrl Pts',(18.0045443718228,70.0339677322408,13.0527532271067));
#58428=CARTESIAN_POINT('Ctrl Pts',(17.880038936804,70.407444765476,14.5827785030239));
#58429=CARTESIAN_POINT('Ctrl Pts',(17.7555335017852,71.8891548095317,15.1166307174996));
#58430=CARTESIAN_POINT('Ctrl Pts',(17.6310280667665,73.1526524587371,14.1763986760686));
#58431=CARTESIAN_POINT('Ctrl Pts',(17.5065226317477,73.0668390544988,12.6037897944718));
#58432=CARTESIAN_POINT('Ctrl Pts',(17.382017196729,71.7085357708834,11.8066230214698));
#58433=CARTESIAN_POINT('Ctrl Pts',(17.2575117617102,70.2937125703898,12.4985319434135));
#58434=CARTESIAN_POINT('Ctrl Pts',(17.1330063266914,70.0889367099268,14.0601111115353));
#58435=CARTESIAN_POINT('Ctrl Pts',(17.0085008916726,71.2775260840903,15.0934154976583));
#58436=CARTESIAN_POINT('Ctrl Pts',(16.8839954566538,72.795440747498,14.6734182044602));
#58437=CARTESIAN_POINT('Ctrl Pts',(16.7594900216351,73.2838246768945,13.1761060159259));
#58438=CARTESIAN_POINT('Ctrl Pts',(16.6349845866163,72.3054705241918,11.9418913654007));
#58439=CARTESIAN_POINT('Ctrl Pts',(16.5104791515975,70.7362130544855,12.0756585083241));
#58440=CARTESIAN_POINT('Ctrl Pts',(16.3859737165788,69.9808710114968,13.4576574408253));
#58441=CARTESIAN_POINT('Ctrl Pts',(16.26146828156,70.715635950286,14.8507055841594));
#58442=CARTESIAN_POINT('Ctrl Pts',(16.1369628465412,72.2827372007522,15.0077289742842));
#58443=CARTESIAN_POINT('Ctrl Pts',(16.0124574115224,73.2792862715224,13.7881583185323));
#58444=CARTESIAN_POINT('Ctrl Pts',(15.8879519765037,72.8131601304144,12.2837684017033));
#58445=CARTESIAN_POINT('Ctrl Pts',(15.7634465414849,71.3016405749555,11.8413076972089));
#58446=CARTESIAN_POINT('Ctrl Pts',(15.6389411064661,70.0978588590303,12.8568725743605));
#58447=CARTESIAN_POINT('Ctrl Pts',(15.5144356714473,70.2794548701458,14.4213166396355));
#58448=CARTESIAN_POINT('Ctrl Pts',(15.3899302364286,71.6838624818643,15.1341304277197));
#58449=CARTESIAN_POINT('Ctrl Pts',(15.2654248014098,73.0538368046712,14.3571936751363));
#58450=CARTESIAN_POINT('Ctrl Pts',(15.140919366391,73.1629634870506,12.7860308639648));
#58451=CARTESIAN_POINT('Ctrl Pts',(15.0164139313723,71.913543523565,11.8271642361628));
#58452=CARTESIAN_POINT('Ctrl Pts',(14.8919084963535,70.4240883638431,12.3389875454574));
#58453=CARTESIAN_POINT('Ctrl Pts',(14.7674030613347,70.0279456674279,13.8633011079927));
#58454=CARTESIAN_POINT('Ctrl Pts',(14.6428976263159,71.0798107346226,15.0355391371328));
#58455=CARTESIAN_POINT('Ctrl Pts',(14.5183921912972,72.6379113282863,14.8062616036466));
#58456=CARTESIAN_POINT('Ctrl Pts',(14.3938867562784,73.3076811621513,13.3807982389934));
#58457=CARTESIAN_POINT('Ctrl Pts',(14.2693813212596,72.4889933638302,12.0350829232256));
#58458=CARTESIAN_POINT('Ctrl Pts',(14.1448758862409,70.9158517355042,11.9741407086008));
#58459=CARTESIAN_POINT('Ctrl Pts',(14.0203704512221,69.9942927747077,13.2518609484195));
#58460=CARTESIAN_POINT('Ctrl Pts',(13.8958650162033,70.5539557793127,14.7257828643058));
#58461=CARTESIAN_POINT('Ctrl Pts',(13.8128613928575,71.5734599327894,14.956586533498));
#58462=CARTESIAN_POINT('Ctrl Pts',(13.7713595811846,72.0212688357496,14.833105713704));
#58463=CARTESIAN_POINT('Ctrl Pts',(19.7877505219048,72.6384078513241,12.6818370233485));
#58464=CARTESIAN_POINT('Ctrl Pts',(19.7462379144259,72.3794178037539,12.3555216261791));
#58465=CARTESIAN_POINT('Ctrl Pts',(19.6632234952739,71.5189853818442,11.983533776499));
#58466=CARTESIAN_POINT('Ctrl Pts',(19.5387072644491,70.3343949062631,12.7551044951164));
#58467=CARTESIAN_POINT('Ctrl Pts',(19.4142018294303,70.3262888641596,14.1675796034986));
#58468=CARTESIAN_POINT('Ctrl Pts',(19.2896963944115,71.4977306447218,14.9550957041578));
#58469=CARTESIAN_POINT('Ctrl Pts',(19.1651909593927,72.8020197752382,14.4133701280415));
#58470=CARTESIAN_POINT('Ctrl Pts',(19.040685524374,73.0705694341706,13.0270131594774));
#58471=CARTESIAN_POINT('Ctrl Pts',(18.9161800893552,72.063445977119,12.0372796911963));
#58472=CARTESIAN_POINT('Ctrl Pts',(18.7916746543364,70.6820060883847,12.3301076943952));
#58473=CARTESIAN_POINT('Ctrl Pts',(18.6671692193177,70.1630458226657,13.6433948901071));
#58474=CARTESIAN_POINT('Ctrl Pts',(18.5426637842989,70.9710890574806,14.8014502359854));
#58475=CARTESIAN_POINT('Ctrl Pts',(18.4181583492801,72.3827927847929,14.7675780533616));
#58476=CARTESIAN_POINT('Ctrl Pts',(18.2936529142613,73.1343689543444,13.5720963304433));
#58477=CARTESIAN_POINT('Ctrl Pts',(18.1691474792426,72.5530038091715,12.2852174808017));
#58478=CARTESIAN_POINT('Ctrl Pts',(18.0446420442238,71.1591394288216,12.058970251175));
#58479=CARTESIAN_POINT('Ctrl Pts',(17.920136609205,70.200582055833,13.0958945307951));
#58480=CARTESIAN_POINT('Ctrl Pts',(17.7956311741862,70.535443365333,14.4677225734024));
#58481=CARTESIAN_POINT('Ctrl Pts',(17.6711257391675,71.8639517380003,14.9463770439872));
#58482=CARTESIAN_POINT('Ctrl Pts',(17.5466203041487,72.9968098248767,14.1033604603431));
#58483=CARTESIAN_POINT('Ctrl Pts',(17.4221148691299,72.9198691127078,12.6933517514775));
#58484=CARTESIAN_POINT('Ctrl Pts',(17.2976094341112,71.7020078367154,11.9786081775955));
#58485=CARTESIAN_POINT('Ctrl Pts',(17.1731039990924,70.4334705306209,12.5989770544976));
#58486=CARTESIAN_POINT('Ctrl Pts',(17.0485985640736,70.2498675063742,13.9990964690587));
#58487=CARTESIAN_POINT('Ctrl Pts',(16.9240931290549,71.3155624725212,14.9255621658968));
#58488=CARTESIAN_POINT('Ctrl Pts',(16.7995876940361,72.6765320815356,14.5489905669191));
#58489=CARTESIAN_POINT('Ctrl Pts',(16.6750822590173,73.1144194683981,13.2064932362542));
#58490=CARTESIAN_POINT('Ctrl Pts',(16.5505768239985,72.2372224159023,12.0998904272434));
#58491=CARTESIAN_POINT('Ctrl Pts',(16.4260713889798,70.8302185991034,12.219826692827));
#58492=CARTESIAN_POINT('Ctrl Pts',(16.301565953961,70.152975279897,13.4589336019084));
#58493=CARTESIAN_POINT('Ctrl Pts',(16.1770605189422,70.8117690682227,14.7079472867197));
#58494=CARTESIAN_POINT('Ctrl Pts',(16.0525550839235,72.21683960845,14.8487352157226));
#58495=CARTESIAN_POINT('Ctrl Pts',(15.9280496489047,73.11035031225,13.7552622830624));
#58496=CARTESIAN_POINT('Ctrl Pts',(15.8035442138859,72.6924193657298,12.4064190270683));
#58497=CARTESIAN_POINT('Ctrl Pts',(15.6790387788671,71.3371836413492,12.009706625168));
#58498=CARTESIAN_POINT('Ctrl Pts',(15.5545333438484,70.2578671482972,12.9202669926942));
#58499=CARTESIAN_POINT('Ctrl Pts',(15.4300279088296,70.4206870078087,14.322955087862));
#58500=CARTESIAN_POINT('Ctrl Pts',(15.3055224738108,71.679885646767,14.962067368582));
#58501=CARTESIAN_POINT('Ctrl Pts',(15.181017038792,72.9082112327946,14.2654621285887));
#58502=CARTESIAN_POINT('Ctrl Pts',(15.0565116037733,73.0060547425988,12.8567499734418));
#58503=CARTESIAN_POINT('Ctrl Pts',(14.9320061687545,71.8858187766437,11.9970255297717));
#58504=CARTESIAN_POINT('Ctrl Pts',(14.8075007337357,70.5503660959109,12.4559287777128));
#58505=CARTESIAN_POINT('Ctrl Pts',(14.6829952987169,70.1951826434738,13.8226356705509));
#58506=CARTESIAN_POINT('Ctrl Pts',(14.5584898636982,71.1382899364899,14.8736699418776));
#58507=CARTESIAN_POINT('Ctrl Pts',(14.4339844286794,72.5352904444127,14.6680985994122));
#58508=CARTESIAN_POINT('Ctrl Pts',(14.3094789936606,73.1358093081533,13.3900212708084));
#58509=CARTESIAN_POINT('Ctrl Pts',(14.1849735586419,72.4017698791616,12.1834464275074));
#58510=CARTESIAN_POINT('Ctrl Pts',(14.0604681236231,70.9912835070088,12.1288053439144));
#58511=CARTESIAN_POINT('Ctrl Pts',(13.9359626886043,70.165009297533,13.2744154741389));
#58512=CARTESIAN_POINT('Ctrl Pts',(13.8114572535856,70.6668058470485,14.5959409735227));
#58513=CARTESIAN_POINT('Ctrl Pts',(13.7284536302397,71.5808981887293,14.8028806566234));
#58514=CARTESIAN_POINT('Ctrl Pts',(13.6869518185668,71.9824058111716,14.6921671579748));
#58515=CARTESIAN_POINT('Ctrl Pts',(19.789,70.1379689624582,12.6747475226976));
#58516=CARTESIAN_POINT('Ctrl Pts',(19.789,70.1415722204682,12.668027089162));
#58517=CARTESIAN_POINT('Ctrl Pts',(19.789,70.1451754784782,12.6613066556264));
#58518=CARTESIAN_POINT('Ctrl Pts',(19.789,70.1487787364881,12.6545862220908));
#58519=CARTESIAN_POINT('Origin',(19.789,71.6454,13.47));
#58520=CARTESIAN_POINT('',(19.939,71.6454,15.32434));
#58521=CARTESIAN_POINT('Origin',(19.939,71.6454,13.47));
#58522=CARTESIAN_POINT('Origin',(19.789,71.6454,15.32434));
#58523=CARTESIAN_POINT('Origin',(19.939,71.6454,13.47));
#58524=CARTESIAN_POINT('',(19.939,71.6454,16.3402));
#58525=CARTESIAN_POINT('Origin',(19.939,71.6454,13.47));
#58526=CARTESIAN_POINT('Origin',(13.764,71.6454,13.47));
#58527=CARTESIAN_POINT('',(13.589,71.6454,14.82434));
#58528=CARTESIAN_POINT('',(13.764,71.6454,14.99934));
#58529=CARTESIAN_POINT('Origin',(13.589,71.6454,13.47));
#58530=CARTESIAN_POINT('Origin',(13.589,71.6454,13.47));
#58531=CARTESIAN_POINT('Origin',(23.4442,74.795221247026,13.8629302123578));
#58532=CARTESIAN_POINT('',(20.539,74.4795530928687,13.9234581415991));
#58533=CARTESIAN_POINT('',(23.1442,74.4795530928687,13.9234581415991));
#58534=CARTESIAN_POINT('',(19.939,74.4795530928687,13.9234581415991));
#58535=CARTESIAN_POINT('',(20.539,74.3538182823342,13.9475672182196));
#58536=CARTESIAN_POINT('',(20.539,74.3538182823342,13.9475672182196));
#58537=CARTESIAN_POINT('',(23.2642,74.3538182823342,13.9475672182196));
#58538=CARTESIAN_POINT('',(23.4442,74.3538182823342,13.9475672182196));
#58539=CARTESIAN_POINT('Ctrl Pts',(23.1442,74.4795530928687,13.9234581415991));
#58540=CARTESIAN_POINT('Ctrl Pts',(23.2056581248801,74.4153434186117,13.935770053868));
#58541=CARTESIAN_POINT('Ctrl Pts',(23.2642,74.3538182823342,13.9475672182196));
#58542=CARTESIAN_POINT('Origin',(23.4442,74.3538182823342,13.9475672182196));
#58543=CARTESIAN_POINT('',(23.1442,74.4637245661282,14.0132261775339));
#58544=CARTESIAN_POINT('',(20.539,74.4637245661282,14.0132261775339));
#58545=CARTESIAN_POINT('',(19.939,74.4637245661282,14.0132261775339));
#58546=CARTESIAN_POINT('Ctrl Pts',(23.2642,74.3538182823342,13.9475672182196));
#58547=CARTESIAN_POINT('Ctrl Pts',(23.2056581248809,74.4075981310439,13.9796957624344));
#58548=CARTESIAN_POINT('Ctrl Pts',(23.1442,74.4637245661282,14.0132261775339));
#58549=CARTESIAN_POINT('',(20.539,74.7396538301726,14.1780686933217));
#58550=CARTESIAN_POINT('Origin',(20.539,74.5606279104667,13.9840333355296));
#58551=CARTESIAN_POINT('Origin',(20.539,71.6454,13.47));
#58552=CARTESIAN_POINT('Origin',(23.2942,71.6454,13.47));
#58553=CARTESIAN_POINT('',(23.2642,71.6454,16.2202));
#58554=CARTESIAN_POINT('',(23.1442,71.5998235737076,16.3398381190176));
#58555=CARTESIAN_POINT('Ctrl Pts',(23.2642,71.6454,16.2202));
#58556=CARTESIAN_POINT('Ctrl Pts',(23.2056581248805,71.6230983332878,16.2787418751195));
#58557=CARTESIAN_POINT('Ctrl Pts',(23.1442,71.5998235737076,16.3398381190176));
#58558=CARTESIAN_POINT('',(23.1442,71.1919418584009,16.3041530928687));
#58559=CARTESIAN_POINT('Origin',(23.1442,71.6454,13.47));
#58560=CARTESIAN_POINT('',(23.2642,71.1678327817804,16.1784182823342));
#58561=CARTESIAN_POINT('Ctrl Pts',(23.1442,71.1919418584009,16.3041530928687));
#58562=CARTESIAN_POINT('Ctrl Pts',(23.2056581248803,71.179629946132,16.2399434186114));
#58563=CARTESIAN_POINT('Ctrl Pts',(23.2642,71.1678327817804,16.1784182823342));
#58564=CARTESIAN_POINT('',(23.1442,71.1021738224661,16.2883245661282));
#58565=CARTESIAN_POINT('Ctrl Pts',(23.2642,71.1678327817804,16.1784182823342));
#58566=CARTESIAN_POINT('Ctrl Pts',(23.2056581248806,71.1357042375654,16.2321981310442));
#58567=CARTESIAN_POINT('Ctrl Pts',(23.1442,71.1021738224661,16.2883245661282));
#58568=CARTESIAN_POINT('',(23.1442,70.7066853866809,16.1823537591437));
#58569=CARTESIAN_POINT('Origin',(23.1442,71.6454,13.47));
#58570=CARTESIAN_POINT('',(23.2642,70.7047762018258,16.0543426456854));
#58571=CARTESIAN_POINT('Ctrl Pts',(23.1442,70.7066853866809,16.1823537591438));
#58572=CARTESIAN_POINT('Ctrl Pts',(23.2056581248804,70.7057104129475,16.1169816329876));
#58573=CARTESIAN_POINT('Ctrl Pts',(23.2642,70.7047762018258,16.0543426456854));
#58574=CARTESIAN_POINT('',(23.1442,70.6210297237434,16.1511776474381));
#58575=CARTESIAN_POINT('Ctrl Pts',(23.2642,70.7047762018258,16.0543426456854));
#58576=CARTESIAN_POINT('Ctrl Pts',(23.2056581248808,70.6637969896664,16.1017263944966));
#58577=CARTESIAN_POINT('Ctrl Pts',(23.1442,70.6210297237434,16.1511776474381));
#58578=CARTESIAN_POINT('',(23.1442,70.2499512834741,15.9781409289644));
#58579=CARTESIAN_POINT('Origin',(23.1442,71.6454,13.47));
#58580=CARTESIAN_POINT('',(23.2642,70.2703,15.851743065488));
#58581=CARTESIAN_POINT('Ctrl Pts',(23.1442,70.2499512834741,15.9781409289644));
#58582=CARTESIAN_POINT('Ctrl Pts',(23.2056581248808,70.2603428723598,15.9135926498824));
#58583=CARTESIAN_POINT('Ctrl Pts',(23.2642,70.2703,15.851743065488));
#58584=CARTESIAN_POINT('',(23.1442,70.1710105975083,15.932564502672));
#58585=CARTESIAN_POINT('Ctrl Pts',(23.2642,70.2703,15.851743065488));
#58586=CARTESIAN_POINT('Ctrl Pts',(23.2056581248807,70.2217152525209,15.8912909831704));
#58587=CARTESIAN_POINT('Ctrl Pts',(23.1442,70.1710105975083,15.932564502672));
#58588=CARTESIAN_POINT('',(23.1442,69.8356171833879,15.697719505839));
#58589=CARTESIAN_POINT('Origin',(23.1442,71.6454,13.47));
#58590=CARTESIAN_POINT('',(23.2642,69.8776055158401,15.5767754274658));
#58591=CARTESIAN_POINT('Ctrl Pts',(23.1442,69.8356171833879,15.697719505839));
#58592=CARTESIAN_POINT('Ctrl Pts',(23.2056581248802,69.8570595917225,15.6359563406292));
#58593=CARTESIAN_POINT('Ctrl Pts',(23.2642,69.8776055158401,15.5767754274658));
#58594=CARTESIAN_POINT('',(23.1442,69.7657900471908,15.6391275816099));
#58595=CARTESIAN_POINT('Ctrl Pts',(23.2642,69.8776055158401,15.5767754274658));
#58596=CARTESIAN_POINT('Ctrl Pts',(23.2056581248808,69.8228914560086,15.6072858705527));
#58597=CARTESIAN_POINT('Ctrl Pts',(23.1442,69.7657900471908,15.6391275816099));
#58598=CARTESIAN_POINT('',(23.1442,69.4762724183901,15.3496099528092));
#58599=CARTESIAN_POINT('Origin',(23.1442,71.6454,13.47));
#58600=CARTESIAN_POINT('',(23.2642,69.5386245725342,15.2377944841599));
#58601=CARTESIAN_POINT('Ctrl Pts',(23.1442,69.4762724183901,15.3496099528092));
#58602=CARTESIAN_POINT('Ctrl Pts',(23.20565812488,69.5081141294468,15.2925085439922));
#58603=CARTESIAN_POINT('Ctrl Pts',(23.2642,69.5386245725342,15.2377944841599));
#58604=CARTESIAN_POINT('',(23.1442,69.417680494161,15.2797828166121));
#58605=CARTESIAN_POINT('Ctrl Pts',(23.2642,69.5386245725342,15.2377944841599));
#58606=CARTESIAN_POINT('Ctrl Pts',(23.2056581248812,69.4794436593718,15.2583404082771));
#58607=CARTESIAN_POINT('Ctrl Pts',(23.1442,69.417680494161,15.2797828166121));
#58608=CARTESIAN_POINT('',(23.1442,69.182835497328,14.9443894024917));
#58609=CARTESIAN_POINT('Origin',(23.1442,71.6454,13.47));
#58610=CARTESIAN_POINT('',(23.2642,69.263656934512,14.8451));
#58611=CARTESIAN_POINT('Ctrl Pts',(23.1442,69.182835497328,14.9443894024917));
#58612=CARTESIAN_POINT('Ctrl Pts',(23.2056581248801,69.2241090168292,14.8936847474796));
#58613=CARTESIAN_POINT('Ctrl Pts',(23.2642,69.263656934512,14.8451));
#58614=CARTESIAN_POINT('',(23.1442,69.1372590710356,14.8654487165258));
#58615=CARTESIAN_POINT('Ctrl Pts',(23.2642,69.263656934512,14.8451));
#58616=CARTESIAN_POINT('Ctrl Pts',(23.2056581248811,69.2018073501179,14.8550571276402));
#58617=CARTESIAN_POINT('Ctrl Pts',(23.1442,69.1372590710356,14.8654487165258));
#58618=CARTESIAN_POINT('',(23.1442,68.9642223525619,14.4943702762566));
#58619=CARTESIAN_POINT('Origin',(23.1442,71.6454,13.47));
#58620=CARTESIAN_POINT('',(23.2642,69.0610573543146,14.4106237981742));
#58621=CARTESIAN_POINT('Ctrl Pts',(23.1442,68.9642223525618,14.4943702762566));
#58622=CARTESIAN_POINT('Ctrl Pts',(23.2056581248796,69.0136736055024,14.4516030103345));
#58623=CARTESIAN_POINT('Ctrl Pts',(23.2642,69.0610573543146,14.4106237981742));
#58624=CARTESIAN_POINT('',(23.1442,68.9330462408563,14.4087146133191));
#58625=CARTESIAN_POINT('Ctrl Pts',(23.2642,69.0610573543146,14.4106237981742));
#58626=CARTESIAN_POINT('Ctrl Pts',(23.2056581248797,68.9984183670117,14.4096895870525));
#58627=CARTESIAN_POINT('Ctrl Pts',(23.1442,68.9330462408562,14.4087146133191));
#58628=CARTESIAN_POINT('',(23.1442,68.8270754338718,14.0132261775338));
#58629=CARTESIAN_POINT('Origin',(23.1442,71.6454,13.47));
#58630=CARTESIAN_POINT('',(23.2642,68.9369817176658,13.9475672182196));
#58631=CARTESIAN_POINT('Ctrl Pts',(23.1442,68.8270754338717,14.0132261775338));
#58632=CARTESIAN_POINT('Ctrl Pts',(23.2056581248802,68.8832018689555,13.9796957624347));
#58633=CARTESIAN_POINT('Ctrl Pts',(23.2642,68.9369817176658,13.9475672182196));
#58634=CARTESIAN_POINT('',(23.1442,68.8112469071312,13.9234581415991));
#58635=CARTESIAN_POINT('Ctrl Pts',(23.2642,68.9369817176658,13.9475672182196));
#58636=CARTESIAN_POINT('Ctrl Pts',(23.2056581248804,68.8754565813886,13.935770053868));
#58637=CARTESIAN_POINT('Ctrl Pts',(23.1442,68.8112469071312,13.9234581415991));
#58638=CARTESIAN_POINT('',(23.1442,68.7755618809824,13.5155764262924));
#58639=CARTESIAN_POINT('Origin',(23.1442,71.6454,13.47));
#58640=CARTESIAN_POINT('',(23.2642,68.8952,13.47));
#58641=CARTESIAN_POINT('Ctrl Pts',(23.1442,68.7755618809824,13.5155764262924));
#58642=CARTESIAN_POINT('Ctrl Pts',(23.2056581248812,68.8366581248812,13.4923016667119));
#58643=CARTESIAN_POINT('Ctrl Pts',(23.2642,68.8952,13.47));
#58644=CARTESIAN_POINT('',(23.1442,68.7755618809824,13.4244235737076));
#58645=CARTESIAN_POINT('Ctrl Pts',(23.2642,68.8952,13.47));
#58646=CARTESIAN_POINT('Ctrl Pts',(23.2056581248805,68.8366581248805,13.4476983332878));
#58647=CARTESIAN_POINT('Ctrl Pts',(23.1442,68.7755618809824,13.4244235737076));
#58648=CARTESIAN_POINT('',(23.1442,68.8112469071312,13.0165418584009));
#58649=CARTESIAN_POINT('Origin',(23.1442,71.6454,13.47));
#58650=CARTESIAN_POINT('',(23.2642,68.9369817176658,12.9924327817804));
#58651=CARTESIAN_POINT('Ctrl Pts',(23.1442,68.8112469071312,13.0165418584009));
#58652=CARTESIAN_POINT('Ctrl Pts',(23.20565812488,68.8754565813883,13.0042299461321));
#58653=CARTESIAN_POINT('Ctrl Pts',(23.2642,68.9369817176658,12.9924327817804));
#58654=CARTESIAN_POINT('',(23.1442,68.8270754338718,12.9267738224661));
#58655=CARTESIAN_POINT('Ctrl Pts',(23.2642,68.9369817176658,12.9924327817804));
#58656=CARTESIAN_POINT('Ctrl Pts',(23.2056581248801,68.8832018689554,12.9603042375652));
#58657=CARTESIAN_POINT('Ctrl Pts',(23.1442,68.8270754338718,12.9267738224661));
#58658=CARTESIAN_POINT('',(23.1442,68.9330462408563,12.5312853866809));
#58659=CARTESIAN_POINT('Origin',(23.1442,71.6454,13.47));
#58660=CARTESIAN_POINT('',(23.2642,69.0610573543146,12.5293762018258));
#58661=CARTESIAN_POINT('Ctrl Pts',(23.1442,68.9330462408562,12.5312853866809));
#58662=CARTESIAN_POINT('Ctrl Pts',(23.2056581248799,68.9984183670118,12.5303104129475));
#58663=CARTESIAN_POINT('Ctrl Pts',(23.2642,69.0610573543146,12.5293762018258));
#58664=CARTESIAN_POINT('',(23.1442,68.9642223525618,12.4456297237434));
#58665=CARTESIAN_POINT('Ctrl Pts',(23.2642,69.0610573543146,12.5293762018258));
#58666=CARTESIAN_POINT('Ctrl Pts',(23.2056581248799,69.0136736055026,12.4883969896657));
#58667=CARTESIAN_POINT('Ctrl Pts',(23.1442,68.9642223525618,12.4456297237434));
#58668=CARTESIAN_POINT('',(23.1442,69.1372590710356,12.0745512834741));
#58669=CARTESIAN_POINT('Origin',(23.1442,71.6454,13.47));
#58670=CARTESIAN_POINT('',(23.2642,69.263656934512,12.0949));
#58671=CARTESIAN_POINT('Ctrl Pts',(23.1442,69.1372590710356,12.0745512834741));
#58672=CARTESIAN_POINT('Ctrl Pts',(23.2056581248798,69.2018073501165,12.0849428723596));
#58673=CARTESIAN_POINT('Ctrl Pts',(23.2642,69.263656934512,12.0949));
#58674=CARTESIAN_POINT('',(23.1442,69.182835497328,11.9956105975083));
#58675=CARTESIAN_POINT('Ctrl Pts',(23.2642,69.263656934512,12.0949));
#58676=CARTESIAN_POINT('Ctrl Pts',(23.2056581248803,69.2241090168293,12.0463152525206));
#58677=CARTESIAN_POINT('Ctrl Pts',(23.1442,69.182835497328,11.9956105975083));
#58678=CARTESIAN_POINT('',(23.1442,69.417680494161,11.6602171833879));
#58679=CARTESIAN_POINT('Origin',(23.1442,71.6454,13.47));
#58680=CARTESIAN_POINT('',(23.2642,69.5386245725342,11.7022055158401));
#58681=CARTESIAN_POINT('Ctrl Pts',(23.1442,69.417680494161,11.6602171833879));
#58682=CARTESIAN_POINT('Ctrl Pts',(23.2056581248803,69.479443659371,11.6816595917226));
#58683=CARTESIAN_POINT('Ctrl Pts',(23.2642,69.5386245725342,11.7022055158401));
#58684=CARTESIAN_POINT('',(23.1442,69.4762724183901,11.5903900471908));
#58685=CARTESIAN_POINT('Ctrl Pts',(23.2642,69.5386245725342,11.7022055158401));
#58686=CARTESIAN_POINT('Ctrl Pts',(23.2056581248804,69.508114129447,11.6474914560082));
#58687=CARTESIAN_POINT('Ctrl Pts',(23.1442,69.4762724183901,11.5903900471908));
#58688=CARTESIAN_POINT('',(23.1442,69.7657900471908,11.3008724183901));
#58689=CARTESIAN_POINT('Origin',(23.1442,71.6454,13.47));
#58690=CARTESIAN_POINT('',(23.2642,69.8776055158401,11.3632245725342));
#58691=CARTESIAN_POINT('Ctrl Pts',(23.1442,69.7657900471908,11.3008724183901));
#58692=CARTESIAN_POINT('Ctrl Pts',(23.2056581248811,69.8228914560089,11.3327141294474));
#58693=CARTESIAN_POINT('Ctrl Pts',(23.2642,69.8776055158401,11.3632245725342));
#58694=CARTESIAN_POINT('',(23.1442,69.8356171833879,11.242280494161));
#58695=CARTESIAN_POINT('Ctrl Pts',(23.2642,69.8776055158401,11.3632245725342));
#58696=CARTESIAN_POINT('Ctrl Pts',(23.2056581248796,69.8570595917223,11.3040436593702));
#58697=CARTESIAN_POINT('Ctrl Pts',(23.1442,69.8356171833879,11.242280494161));
#58698=CARTESIAN_POINT('',(23.1442,70.1710105975083,11.007435497328));
#58699=CARTESIAN_POINT('Origin',(23.1442,71.6454,13.47));
#58700=CARTESIAN_POINT('',(23.2642,70.2703,11.0882569345121));
#58701=CARTESIAN_POINT('Ctrl Pts',(23.1442,70.1710105975083,11.007435497328));
#58702=CARTESIAN_POINT('Ctrl Pts',(23.2056581248807,70.2217152525209,11.0487090168296));
#58703=CARTESIAN_POINT('Ctrl Pts',(23.2642,70.2703,11.0882569345121));
#58704=CARTESIAN_POINT('',(23.1442,70.2499512834741,10.9618590710356));
#58705=CARTESIAN_POINT('Ctrl Pts',(23.2642,70.2703,11.0882569345121));
#58706=CARTESIAN_POINT('Ctrl Pts',(23.205658124881,70.2603428723598,11.0264073501178));
#58707=CARTESIAN_POINT('Ctrl Pts',(23.1442,70.2499512834741,10.9618590710356));
#58708=CARTESIAN_POINT('',(23.1442,70.6210297237434,10.7888223525619));
#58709=CARTESIAN_POINT('Origin',(23.1442,71.6454,13.47));
#58710=CARTESIAN_POINT('',(23.2642,70.7047762018258,10.8856573543146));
#58711=CARTESIAN_POINT('Ctrl Pts',(23.1442,70.6210297237434,10.7888223525619));
#58712=CARTESIAN_POINT('Ctrl Pts',(23.2056581248802,70.6637969896659,10.8382736055029));
#58713=CARTESIAN_POINT('Ctrl Pts',(23.2642,70.7047762018258,10.8856573543146));
#58714=CARTESIAN_POINT('',(23.1442,70.7066853866809,10.7576462408563));
#58715=CARTESIAN_POINT('Ctrl Pts',(23.2642,70.7047762018258,10.8856573543146));
#58716=CARTESIAN_POINT('Ctrl Pts',(23.2056581248805,70.7057104129475,10.8230183670125));
#58717=CARTESIAN_POINT('Ctrl Pts',(23.1442,70.7066853866809,10.7576462408562));
#58718=CARTESIAN_POINT('',(23.1442,71.1021738224661,10.6516754338718));
#58719=CARTESIAN_POINT('Origin',(23.1442,71.6454,13.47));
#58720=CARTESIAN_POINT('',(23.2642,71.1678327817804,10.7615817176658));
#58721=CARTESIAN_POINT('Ctrl Pts',(23.1442,71.1021738224662,10.6516754338718));
#58722=CARTESIAN_POINT('Ctrl Pts',(23.2056581248805,71.1357042375654,10.7078018689558));
#58723=CARTESIAN_POINT('Ctrl Pts',(23.2642,71.1678327817804,10.7615817176658));
#58724=CARTESIAN_POINT('',(23.1442,71.1919418584009,10.6358469071313));
#58725=CARTESIAN_POINT('Ctrl Pts',(23.2642,71.1678327817804,10.7615817176658));
#58726=CARTESIAN_POINT('Ctrl Pts',(23.2056581248808,71.1796299461319,10.7000565813891));
#58727=CARTESIAN_POINT('Ctrl Pts',(23.1442,71.1919418584009,10.6358469071313));
#58728=CARTESIAN_POINT('',(23.1442,71.5998235737076,10.6001618809824));
#58729=CARTESIAN_POINT('Origin',(23.1442,71.6454,13.47));
#58730=CARTESIAN_POINT('',(23.2642,71.6454,10.7198));
#58731=CARTESIAN_POINT('Ctrl Pts',(23.1442,71.5998235737076,10.6001618809824));
#58732=CARTESIAN_POINT('Ctrl Pts',(23.2056581248805,71.6230983332878,10.6612581248805));
#58733=CARTESIAN_POINT('Ctrl Pts',(23.2642,71.6454,10.7198));
#58734=CARTESIAN_POINT('',(23.1442,71.6909764262924,10.6001618809824));
#58735=CARTESIAN_POINT('Ctrl Pts',(23.2642,71.6454,10.7198));
#58736=CARTESIAN_POINT('Ctrl Pts',(23.2056581248811,71.667701666712,10.6612581248811));
#58737=CARTESIAN_POINT('Ctrl Pts',(23.1442,71.6909764262924,10.6001618809824));
#58738=CARTESIAN_POINT('',(23.1442,72.0988581415992,10.6358469071313));
#58739=CARTESIAN_POINT('Origin',(23.1442,71.6454,13.47));
#58740=CARTESIAN_POINT('',(23.2642,72.1229672182196,10.7615817176658));
#58741=CARTESIAN_POINT('Ctrl Pts',(23.1442,72.0988581415992,10.6358469071313));
#58742=CARTESIAN_POINT('Ctrl Pts',(23.2056581248808,72.1111700538681,10.7000565813891));
#58743=CARTESIAN_POINT('Ctrl Pts',(23.2642,72.1229672182196,10.7615817176658));
#58744=CARTESIAN_POINT('',(23.1442,72.1886261775339,10.6516754338718));
#58745=CARTESIAN_POINT('Ctrl Pts',(23.2642,72.1229672182196,10.7615817176658));
#58746=CARTESIAN_POINT('Ctrl Pts',(23.2056581248801,72.1550957624348,10.7078018689554));
#58747=CARTESIAN_POINT('Ctrl Pts',(23.1442,72.1886261775339,10.6516754338718));
#58748=CARTESIAN_POINT('',(23.1442,72.5841146133191,10.7576462408563));
#58749=CARTESIAN_POINT('Origin',(23.1442,71.6454,13.47));
#58750=CARTESIAN_POINT('',(23.2642,72.5860237981743,10.8856573543146));
#58751=CARTESIAN_POINT('Ctrl Pts',(23.1442,72.5841146133191,10.7576462408563));
#58752=CARTESIAN_POINT('Ctrl Pts',(23.2056581248803,72.5850895870525,10.8230183670123));
#58753=CARTESIAN_POINT('Ctrl Pts',(23.2642,72.5860237981742,10.8856573543146));
#58754=CARTESIAN_POINT('',(23.1442,72.6697702762566,10.7888223525619));
#58755=CARTESIAN_POINT('Ctrl Pts',(23.2642,72.5860237981743,10.8856573543146));
#58756=CARTESIAN_POINT('Ctrl Pts',(23.2056581248806,72.6270030103338,10.8382736055032));
#58757=CARTESIAN_POINT('Ctrl Pts',(23.1442,72.6697702762566,10.7888223525619));
#58758=CARTESIAN_POINT('',(23.1442,73.0408487165258,10.9618590710356));
#58759=CARTESIAN_POINT('Origin',(23.1442,71.6454,13.47));
#58760=CARTESIAN_POINT('',(23.2642,73.0205,11.088256934512));
#58761=CARTESIAN_POINT('Ctrl Pts',(23.1442,73.0408487165258,10.9618590710356));
#58762=CARTESIAN_POINT('Ctrl Pts',(23.2056581248806,73.0304571276402,11.0264073501174));
#58763=CARTESIAN_POINT('Ctrl Pts',(23.2642,73.0205,11.088256934512));
#58764=CARTESIAN_POINT('',(23.1442,73.1197894024917,11.007435497328));
#58765=CARTESIAN_POINT('Ctrl Pts',(23.2642,73.0205,11.088256934512));
#58766=CARTESIAN_POINT('Ctrl Pts',(23.2056581248807,73.0690847474791,11.0487090168296));
#58767=CARTESIAN_POINT('Ctrl Pts',(23.1442,73.1197894024917,11.007435497328));
#58768=CARTESIAN_POINT('',(23.1442,73.4551828166121,11.242280494161));
#58769=CARTESIAN_POINT('Origin',(23.1442,71.6454,13.47));
#58770=CARTESIAN_POINT('',(23.2642,73.4131944841599,11.3632245725342));
#58771=CARTESIAN_POINT('Ctrl Pts',(23.1442,73.4551828166121,11.242280494161));
#58772=CARTESIAN_POINT('Ctrl Pts',(23.2056581248799,73.4337404082776,11.3040436593706));
#58773=CARTESIAN_POINT('Ctrl Pts',(23.2642,73.4131944841599,11.3632245725342));
#58774=CARTESIAN_POINT('',(23.1442,73.5250099528092,11.3008724183901));
#58775=CARTESIAN_POINT('Ctrl Pts',(23.2642,73.4131944841599,11.3632245725342));
#58776=CARTESIAN_POINT('Ctrl Pts',(23.2056581248809,73.4679085439913,11.3327141294473));
#58777=CARTESIAN_POINT('Ctrl Pts',(23.1442,73.5250099528091,11.3008724183901));
#58778=CARTESIAN_POINT('',(23.1442,73.8145275816099,11.5903900471908));
#58779=CARTESIAN_POINT('Origin',(23.1442,71.6454,13.47));
#58780=CARTESIAN_POINT('',(23.2642,73.7521754274658,11.7022055158401));
#58781=CARTESIAN_POINT('Ctrl Pts',(23.1442,73.8145275816099,11.5903900471908));
#58782=CARTESIAN_POINT('Ctrl Pts',(23.2056581248799,73.7826858705532,11.6474914560077));
#58783=CARTESIAN_POINT('Ctrl Pts',(23.2642,73.7521754274658,11.7022055158401));
#58784=CARTESIAN_POINT('',(23.1442,73.873119505839,11.6602171833879));
#58785=CARTESIAN_POINT('Ctrl Pts',(23.2642,73.7521754274658,11.7022055158401));
#58786=CARTESIAN_POINT('Ctrl Pts',(23.2056581248803,73.811356340629,11.6816595917226));
#58787=CARTESIAN_POINT('Ctrl Pts',(23.1442,73.873119505839,11.6602171833879));
#58788=CARTESIAN_POINT('',(23.1442,74.107964502672,11.9956105975083));
#58789=CARTESIAN_POINT('Origin',(23.1442,71.6454,13.47));
#58790=CARTESIAN_POINT('',(23.2642,74.027143065488,12.0949));
#58791=CARTESIAN_POINT('Ctrl Pts',(23.1442,74.107964502672,11.9956105975083));
#58792=CARTESIAN_POINT('Ctrl Pts',(23.20565812488,74.0666909831708,12.0463152525204));
#58793=CARTESIAN_POINT('Ctrl Pts',(23.2642,74.027143065488,12.0949));
#58794=CARTESIAN_POINT('',(23.1442,74.1535409289644,12.0745512834741));
#58795=CARTESIAN_POINT('Ctrl Pts',(23.2642,74.0271430654879,12.0949));
#58796=CARTESIAN_POINT('Ctrl Pts',(23.2056581248806,74.0889926498826,12.0849428723598));
#58797=CARTESIAN_POINT('Ctrl Pts',(23.1442,74.1535409289644,12.0745512834741));
#58798=CARTESIAN_POINT('',(23.1442,74.3265776474381,12.4456297237434));
#58799=CARTESIAN_POINT('Origin',(23.1442,71.6454,13.47));
#58800=CARTESIAN_POINT('',(23.2642,74.2297426456854,12.5293762018257));
#58801=CARTESIAN_POINT('Ctrl Pts',(23.1442,74.3265776474381,12.4456297237434));
#58802=CARTESIAN_POINT('Ctrl Pts',(23.2056581248805,74.2771263944969,12.4883969896661));
#58803=CARTESIAN_POINT('Ctrl Pts',(23.2642,74.2297426456854,12.5293762018257));
#58804=CARTESIAN_POINT('',(23.1442,74.3577537591437,12.5312853866809));
#58805=CARTESIAN_POINT('Ctrl Pts',(23.2642,74.2297426456854,12.5293762018257));
#58806=CARTESIAN_POINT('Ctrl Pts',(23.2056581248808,74.2923816329872,12.5303104129475));
#58807=CARTESIAN_POINT('Ctrl Pts',(23.1442,74.3577537591437,12.5312853866809));
#58808=CARTESIAN_POINT('',(23.1442,74.4637245661282,12.9267738224661));
#58809=CARTESIAN_POINT('Origin',(23.1442,71.6454,13.47));
#58810=CARTESIAN_POINT('',(23.2642,74.3538182823342,12.9924327817804));
#58811=CARTESIAN_POINT('Ctrl Pts',(23.1442,74.4637245661282,12.9267738224661));
#58812=CARTESIAN_POINT('Ctrl Pts',(23.2056581248812,74.4075981310436,12.9603042375658));
#58813=CARTESIAN_POINT('Ctrl Pts',(23.2642,74.3538182823342,12.9924327817804));
#58814=CARTESIAN_POINT('',(23.1442,74.4795530928687,13.0165418584009));
#58815=CARTESIAN_POINT('Ctrl Pts',(23.2642,74.3538182823342,12.9924327817804));
#58816=CARTESIAN_POINT('Ctrl Pts',(23.2056581248806,74.4153434186111,13.0042299461319));
#58817=CARTESIAN_POINT('Ctrl Pts',(23.1442,74.4795530928687,13.0165418584009));
#58818=CARTESIAN_POINT('',(23.1442,74.5152381190176,13.4244235737076));
#58819=CARTESIAN_POINT('Origin',(23.1442,71.6454,13.47));
#58820=CARTESIAN_POINT('',(23.2642,74.3956,13.47));
#58821=CARTESIAN_POINT('Ctrl Pts',(23.1442,74.5152381190176,13.4244235737076));
#58822=CARTESIAN_POINT('Ctrl Pts',(23.2056581248811,74.4541418751189,13.447698333288));
#58823=CARTESIAN_POINT('Ctrl Pts',(23.2642,74.3956,13.47));
#58824=CARTESIAN_POINT('',(23.1442,74.5152381190176,13.5155764262924));
#58825=CARTESIAN_POINT('Ctrl Pts',(23.2642,74.3956,13.47));
#58826=CARTESIAN_POINT('Ctrl Pts',(23.2056581248807,74.4541418751193,13.4923016667121));
#58827=CARTESIAN_POINT('Ctrl Pts',(23.1442,74.5152381190176,13.5155764262924));
#58828=CARTESIAN_POINT('Origin',(23.1442,71.6454,13.47));
#58829=CARTESIAN_POINT('',(23.1442,74.3577537591437,14.4087146133191));
#58830=CARTESIAN_POINT('Origin',(23.1442,71.6454,13.47));
#58831=CARTESIAN_POINT('',(23.2642,74.2297426456854,14.4106237981743));
#58832=CARTESIAN_POINT('Ctrl Pts',(23.1442,74.3577537591437,14.4087146133191));
#58833=CARTESIAN_POINT('Ctrl Pts',(23.2056581248805,74.2923816329875,14.4096895870525));
#58834=CARTESIAN_POINT('Ctrl Pts',(23.2642,74.2297426456854,14.4106237981743));
#58835=CARTESIAN_POINT('',(23.1442,74.3265776474381,14.4943702762566));
#58836=CARTESIAN_POINT('Ctrl Pts',(23.2642,74.2297426456854,14.4106237981743));
#58837=CARTESIAN_POINT('Ctrl Pts',(23.20565812488,74.2771263944972,14.4516030103342));
#58838=CARTESIAN_POINT('Ctrl Pts',(23.1442,74.3265776474381,14.4943702762567));
#58839=CARTESIAN_POINT('',(23.1442,74.1535409289644,14.8654487165258));
#58840=CARTESIAN_POINT('Origin',(23.1442,71.6454,13.47));
#58841=CARTESIAN_POINT('',(23.2642,74.0271430654879,14.8451));
#58842=CARTESIAN_POINT('Ctrl Pts',(23.1442,74.1535409289644,14.8654487165259));
#58843=CARTESIAN_POINT('Ctrl Pts',(23.2056581248803,74.0889926498829,14.8550571276403));
#58844=CARTESIAN_POINT('Ctrl Pts',(23.2642,74.0271430654879,14.8451));
#58845=CARTESIAN_POINT('',(23.1442,74.107964502672,14.9443894024917));
#58846=CARTESIAN_POINT('Ctrl Pts',(23.2642,74.0271430654879,14.8451));
#58847=CARTESIAN_POINT('Ctrl Pts',(23.2056581248802,74.0666909831707,14.8936847474795));
#58848=CARTESIAN_POINT('Ctrl Pts',(23.1442,74.107964502672,14.9443894024917));
#58849=CARTESIAN_POINT('',(23.1442,73.873119505839,15.2797828166121));
#58850=CARTESIAN_POINT('Origin',(23.1442,71.6454,13.47));
#58851=CARTESIAN_POINT('',(23.2642,73.7521754274658,15.2377944841599));
#58852=CARTESIAN_POINT('Ctrl Pts',(23.1442,73.873119505839,15.2797828166121));
#58853=CARTESIAN_POINT('Ctrl Pts',(23.2056581248798,73.8113563406296,15.2583404082776));
#58854=CARTESIAN_POINT('Ctrl Pts',(23.2642,73.7521754274658,15.2377944841599));
#58855=CARTESIAN_POINT('',(23.1442,73.8145275816099,15.3496099528092));
#58856=CARTESIAN_POINT('Ctrl Pts',(23.2642,73.7521754274658,15.2377944841599));
#58857=CARTESIAN_POINT('Ctrl Pts',(23.2056581248795,73.7826858705534,15.2925085439927));
#58858=CARTESIAN_POINT('Ctrl Pts',(23.1442,73.8145275816099,15.3496099528092));
#58859=CARTESIAN_POINT('',(23.1442,73.5250099528092,15.6391275816099));
#58860=CARTESIAN_POINT('Origin',(23.1442,71.6454,13.47));
#58861=CARTESIAN_POINT('',(23.2642,73.4131944841599,15.5767754274658));
#58862=CARTESIAN_POINT('Ctrl Pts',(23.1442,73.5250099528092,15.6391275816099));
#58863=CARTESIAN_POINT('Ctrl Pts',(23.2056581248799,73.4679085439923,15.6072858705533));
#58864=CARTESIAN_POINT('Ctrl Pts',(23.2642,73.4131944841599,15.5767754274658));
#58865=CARTESIAN_POINT('',(23.1442,73.4551828166121,15.697719505839));
#58866=CARTESIAN_POINT('Ctrl Pts',(23.2642,73.4131944841599,15.5767754274658));
#58867=CARTESIAN_POINT('Ctrl Pts',(23.2056581248798,73.4337404082776,15.6359563406295));
#58868=CARTESIAN_POINT('Ctrl Pts',(23.1442,73.4551828166121,15.697719505839));
#58869=CARTESIAN_POINT('',(23.1442,73.1197894024917,15.932564502672));
#58870=CARTESIAN_POINT('Origin',(23.1442,71.6454,13.47));
#58871=CARTESIAN_POINT('',(23.2642,73.0205,15.8517430654879));
#58872=CARTESIAN_POINT('Ctrl Pts',(23.1442,73.1197894024917,15.932564502672));
#58873=CARTESIAN_POINT('Ctrl Pts',(23.2056581248807,73.0690847474791,15.8912909831704));
#58874=CARTESIAN_POINT('Ctrl Pts',(23.2642,73.0205,15.8517430654879));
#58875=CARTESIAN_POINT('',(23.1442,73.0408487165259,15.9781409289644));
#58876=CARTESIAN_POINT('Ctrl Pts',(23.2642,73.0205,15.8517430654879));
#58877=CARTESIAN_POINT('Ctrl Pts',(23.2056581248811,73.0304571276402,15.9135926498821));
#58878=CARTESIAN_POINT('Ctrl Pts',(23.1442,73.0408487165259,15.9781409289644));
#58879=CARTESIAN_POINT('',(23.1442,72.6697702762566,16.1511776474381));
#58880=CARTESIAN_POINT('Origin',(23.1442,71.6454,13.47));
#58881=CARTESIAN_POINT('',(23.2642,72.5860237981742,16.0543426456854));
#58882=CARTESIAN_POINT('Ctrl Pts',(23.1442,72.6697702762566,16.1511776474381));
#58883=CARTESIAN_POINT('Ctrl Pts',(23.2056581248799,72.6270030103342,16.1017263944973));
#58884=CARTESIAN_POINT('Ctrl Pts',(23.2642,72.5860237981742,16.0543426456854));
#58885=CARTESIAN_POINT('',(23.1442,72.5841146133191,16.1823537591437));
#58886=CARTESIAN_POINT('Ctrl Pts',(23.2642,72.5860237981742,16.0543426456854));
#58887=CARTESIAN_POINT('Ctrl Pts',(23.2056581248803,72.5850895870525,16.1169816329877));
#58888=CARTESIAN_POINT('Ctrl Pts',(23.1442,72.5841146133191,16.1823537591438));
#58889=CARTESIAN_POINT('',(23.1442,72.1886261775338,16.2883245661282));
#58890=CARTESIAN_POINT('Origin',(23.1442,71.6454,13.47));
#58891=CARTESIAN_POINT('',(23.2642,72.1229672182196,16.1784182823342));
#58892=CARTESIAN_POINT('Ctrl Pts',(23.1442,72.1886261775338,16.2883245661282));
#58893=CARTESIAN_POINT('Ctrl Pts',(23.2056581248799,72.1550957624349,16.2321981310448));
#58894=CARTESIAN_POINT('Ctrl Pts',(23.2642,72.1229672182196,16.1784182823342));
#58895=CARTESIAN_POINT('',(23.1442,72.0988581415991,16.3041530928687));
#58896=CARTESIAN_POINT('Ctrl Pts',(23.2642,72.1229672182196,16.1784182823342));
#58897=CARTESIAN_POINT('Ctrl Pts',(23.2056581248806,72.1111700538681,16.2399434186111));
#58898=CARTESIAN_POINT('Ctrl Pts',(23.1442,72.0988581415991,16.3041530928687));
#58899=CARTESIAN_POINT('',(23.1442,71.6909764262924,16.3398381190176));
#58900=CARTESIAN_POINT('Origin',(23.1442,71.6454,13.47));
#58901=CARTESIAN_POINT('Ctrl Pts',(23.1442,71.6909764262924,16.3398381190176));
#58902=CARTESIAN_POINT('Ctrl Pts',(23.2056581248802,71.6677016667123,16.2787418751198));
#58903=CARTESIAN_POINT('Ctrl Pts',(23.2642,71.6454,16.2202));
#58904=CARTESIAN_POINT('',(23.4442,71.6454,16.0402));
#58905=CARTESIAN_POINT('',(23.2942,71.6454,16.1902));
#58906=CARTESIAN_POINT('Origin',(23.4442,71.6454,13.47));
#58907=CARTESIAN_POINT('Origin',(23.4442,74.6791367693476,14.4039214390453));
#58908=CARTESIAN_POINT('',(20.539,74.3577537591437,14.4087146133191));
#58909=CARTESIAN_POINT('',(19.939,74.3577537591437,14.4087146133191));
#58910=CARTESIAN_POINT('',(20.539,74.2297426456854,14.4106237981743));
#58911=CARTESIAN_POINT('',(20.539,74.2297426456854,14.4106237981743));
#58912=CARTESIAN_POINT('',(23.4442,74.2297426456854,14.4106237981743));
#58913=CARTESIAN_POINT('Origin',(23.4442,74.2297426456854,14.4106237981743));
#58914=CARTESIAN_POINT('',(20.539,74.3265776474381,14.4943702762566));
#58915=CARTESIAN_POINT('',(19.939,74.3265776474381,14.4943702762566));
#58916=CARTESIAN_POINT('',(20.539,74.5696903234834,14.7046230776968));
#58917=CARTESIAN_POINT('Origin',(20.539,74.4270780960504,14.4824480282726));
#58918=CARTESIAN_POINT('Origin',(20.539,71.6454,13.47));
#58919=CARTESIAN_POINT('Origin',(23.4442,74.4708737350774,14.9165359353945));
#58920=CARTESIAN_POINT('',(20.539,74.1535409289644,14.8654487165258));
#58921=CARTESIAN_POINT('',(19.939,74.1535409289644,14.8654487165258));
#58922=CARTESIAN_POINT('',(20.539,74.0271430654879,14.8451));
#58923=CARTESIAN_POINT('',(20.539,74.0271430654879,14.8451));
#58924=CARTESIAN_POINT('',(23.4442,74.0271430654879,14.8451));
#58925=CARTESIAN_POINT('Origin',(23.4442,74.0271430654879,14.8451));
#58926=CARTESIAN_POINT('',(20.539,74.107964502672,14.9443894024917));
#58927=CARTESIAN_POINT('',(19.939,74.107964502672,14.9443894024917));
#58928=CARTESIAN_POINT('',(20.539,74.3108737350774,15.1936640646055));
#58929=CARTESIAN_POINT('Origin',(20.539,74.2090084002827,14.9501));
#58930=CARTESIAN_POINT('Origin',(20.539,71.6454,13.47));
#58931=CARTESIAN_POINT('Origin',(23.4442,74.1767601111256,15.3851981693292));
#58932=CARTESIAN_POINT('',(20.539,73.873119505839,15.2797828166121));
#58933=CARTESIAN_POINT('',(19.939,73.873119505839,15.2797828166121));
#58934=CARTESIAN_POINT('',(20.539,73.7521754274658,15.2377944841599));
#58935=CARTESIAN_POINT('',(20.539,73.7521754274658,15.2377944841599));
#58936=CARTESIAN_POINT('',(23.4442,73.7521754274658,15.2377944841599));
#58937=CARTESIAN_POINT('Origin',(23.4442,73.7521754274658,15.2377944841599));
#58938=CARTESIAN_POINT('',(20.539,73.8145275816099,15.3496099528092));
#58939=CARTESIAN_POINT('',(19.939,73.8145275816099,15.3496099528092));
#58940=CARTESIAN_POINT('',(20.539,73.9710680760259,15.6303323911273));
#58941=CARTESIAN_POINT('Origin',(20.539,73.9130447605208,15.3727798821941));
#58942=CARTESIAN_POINT('Origin',(20.539,71.6454,13.47));
#58943=CARTESIAN_POINT('Origin',(23.4442,73.8057323911273,15.7956680760259));
#58944=CARTESIAN_POINT('',(20.539,73.5250099528092,15.6391275816099));
#58945=CARTESIAN_POINT('',(19.939,73.5250099528092,15.6391275816099));
#58946=CARTESIAN_POINT('',(20.539,73.4131944841599,15.5767754274658));
#58947=CARTESIAN_POINT('',(20.539,73.4131944841599,15.5767754274658));
#58948=CARTESIAN_POINT('',(23.4442,73.4131944841599,15.5767754274658));
#58949=CARTESIAN_POINT('Origin',(23.4442,73.4131944841599,15.5767754274658));
#58950=CARTESIAN_POINT('',(20.539,73.4551828166121,15.697719505839));
#58951=CARTESIAN_POINT('',(19.939,73.4551828166121,15.697719505839));
#58952=CARTESIAN_POINT('',(20.539,73.5605981693292,16.0013601111256));
#58953=CARTESIAN_POINT('Origin',(20.539,73.5481798821941,15.7376447605208));
#58954=CARTESIAN_POINT('Origin',(20.539,71.6454,13.47));
#58955=CARTESIAN_POINT('Origin',(23.4442,73.3690640646055,16.1354737350774));
#58956=CARTESIAN_POINT('',(20.539,73.1197894024917,15.932564502672));
#58957=CARTESIAN_POINT('',(19.939,73.1197894024917,15.932564502672));
#58958=CARTESIAN_POINT('',(20.539,73.0205,15.8517430654879));
#58959=CARTESIAN_POINT('',(20.539,73.0205,15.8517430654879));
#58960=CARTESIAN_POINT('',(23.4442,73.0205,15.8517430654879));
#58961=CARTESIAN_POINT('Origin',(23.4442,73.0205,15.8517430654879));
#58962=CARTESIAN_POINT('',(20.539,73.0408487165258,15.9781409289644));
#58963=CARTESIAN_POINT('',(19.939,73.0408487165259,15.9781409289644));
#58964=CARTESIAN_POINT('',(20.539,73.0919359353945,16.2954737350774));
#58965=CARTESIAN_POINT('Origin',(20.539,73.1255,16.0336084002827));
#58966=CARTESIAN_POINT('Origin',(20.539,71.6454,13.47));
#58967=CARTESIAN_POINT('Origin',(23.4442,72.8800230776968,16.3942903234834));
#58968=CARTESIAN_POINT('',(20.539,72.6697702762566,16.1511776474381));
#58969=CARTESIAN_POINT('',(19.939,72.6697702762566,16.1511776474381));
#58970=CARTESIAN_POINT('',(20.539,72.5860237981742,16.0543426456854));
#58971=CARTESIAN_POINT('',(20.539,72.5860237981742,16.0543426456854));
#58972=CARTESIAN_POINT('',(23.4442,72.5860237981742,16.0543426456854));
#58973=CARTESIAN_POINT('Origin',(23.4442,72.5860237981742,16.0543426456854));
#58974=CARTESIAN_POINT('',(20.539,72.5841146133191,16.1823537591437));
#58975=CARTESIAN_POINT('',(19.939,72.5841146133191,16.1823537591437));
#58976=CARTESIAN_POINT('',(20.539,72.5793214390453,16.5037367693476));
#58977=CARTESIAN_POINT('Origin',(20.539,72.6578480282726,16.2516780960504));
#58978=CARTESIAN_POINT('Origin',(20.539,71.6454,13.47));
#58979=CARTESIAN_POINT('Origin',(23.4442,72.3534686933216,16.5642538301726));
#58980=CARTESIAN_POINT('',(20.539,72.1886261775338,16.2883245661282));
#58981=CARTESIAN_POINT('',(19.939,72.1886261775338,16.2883245661282));
#58982=CARTESIAN_POINT('',(20.539,72.1229672182196,16.1784182823342));
#58983=CARTESIAN_POINT('',(20.539,72.1229672182196,16.1784182823342));
#58984=CARTESIAN_POINT('',(23.4442,72.1229672182196,16.1784182823342));
#58985=CARTESIAN_POINT('Origin',(23.4442,72.1229672182196,16.1784182823342));
#58986=CARTESIAN_POINT('',(20.539,72.0988581415991,16.3041530928687));
#58987=CARTESIAN_POINT('',(19.939,72.0988581415991,16.3041530928687));
#58988=CARTESIAN_POINT('',(20.539,72.0383302123577,16.619821247026));
#58989=CARTESIAN_POINT('Origin',(20.539,72.1594333355296,16.3852279104667));
#58990=CARTESIAN_POINT('Origin',(20.539,71.6454,13.47));
#58991=CARTESIAN_POINT('Origin',(23.4442,71.8054,16.6402));
#58992=CARTESIAN_POINT('',(20.539,71.6909764262924,16.3398381190176));
#58993=CARTESIAN_POINT('',(19.939,71.6909764262924,16.3398381190176));
#58994=CARTESIAN_POINT('',(20.539,71.6454,16.2202));
#58995=CARTESIAN_POINT('',(20.539,71.6454,16.2202));
#58996=CARTESIAN_POINT('',(23.4442,71.6454,16.2202));
#58997=CARTESIAN_POINT('Origin',(23.4442,71.6454,16.2202));
#58998=CARTESIAN_POINT('',(20.539,71.5998235737076,16.3398381190176));
#58999=CARTESIAN_POINT('',(19.939,71.5998235737076,16.3398381190176));
#59000=CARTESIAN_POINT('',(20.539,71.4854,16.6402));
#59001=CARTESIAN_POINT('Origin',(20.539,71.6454,16.4302));
#59002=CARTESIAN_POINT('',(20.539,71.6454,16.3402));
#59003=CARTESIAN_POINT('Origin',(20.539,71.6454,13.47));
#59004=CARTESIAN_POINT('Origin',(20.539,71.6454,13.47));
#59005=CARTESIAN_POINT('Origin',(23.4442,71.2524697876423,16.619821247026));
#59006=CARTESIAN_POINT('',(20.539,71.1919418584009,16.3041530928687));
#59007=CARTESIAN_POINT('',(19.939,71.1919418584009,16.3041530928687));
#59008=CARTESIAN_POINT('',(20.539,71.1678327817804,16.1784182823342));
#59009=CARTESIAN_POINT('',(20.539,71.1678327817804,16.1784182823342));
#59010=CARTESIAN_POINT('',(23.4442,71.1678327817804,16.1784182823342));
#59011=CARTESIAN_POINT('Origin',(23.4442,71.1678327817804,16.1784182823342));
#59012=CARTESIAN_POINT('',(20.539,71.1021738224661,16.2883245661282));
#59013=CARTESIAN_POINT('',(19.939,71.1021738224661,16.2883245661282));
#59014=CARTESIAN_POINT('',(20.539,70.9373313066783,16.5642538301726));
#59015=CARTESIAN_POINT('Origin',(20.539,71.1313666644703,16.3852279104667));
#59016=CARTESIAN_POINT('Origin',(20.539,71.6454,13.47));
#59017=CARTESIAN_POINT('Origin',(23.4442,70.7114785609547,16.5037367693476));
#59018=CARTESIAN_POINT('',(20.539,70.7066853866809,16.1823537591438));
#59019=CARTESIAN_POINT('',(19.939,70.7066853866809,16.1823537591437));
#59020=CARTESIAN_POINT('',(20.539,70.7047762018258,16.0543426456854));
#59021=CARTESIAN_POINT('',(20.539,70.7047762018258,16.0543426456854));
#59022=CARTESIAN_POINT('',(23.4442,70.7047762018258,16.0543426456854));
#59023=CARTESIAN_POINT('Origin',(23.4442,70.7047762018258,16.0543426456854));
#59024=CARTESIAN_POINT('',(20.539,70.6210297237434,16.1511776474381));
#59025=CARTESIAN_POINT('',(19.939,70.6210297237434,16.1511776474381));
#59026=CARTESIAN_POINT('',(20.539,70.4107769223032,16.3942903234834));
#59027=CARTESIAN_POINT('Origin',(20.539,70.6329519717274,16.2516780960504));
#59028=CARTESIAN_POINT('Origin',(20.539,71.6454,13.47));
#59029=CARTESIAN_POINT('Origin',(23.4442,70.1988640646055,16.2954737350774));
#59030=CARTESIAN_POINT('',(20.539,70.2499512834741,15.9781409289644));
#59031=CARTESIAN_POINT('',(19.939,70.2499512834741,15.9781409289644));
#59032=CARTESIAN_POINT('',(20.539,70.2703,15.851743065488));
#59033=CARTESIAN_POINT('',(20.539,70.2703,15.851743065488));
#59034=CARTESIAN_POINT('',(23.4442,70.2703,15.851743065488));
#59035=CARTESIAN_POINT('Origin',(23.4442,70.2703,15.851743065488));
#59036=CARTESIAN_POINT('',(20.539,70.1710105975083,15.932564502672));
#59037=CARTESIAN_POINT('',(19.939,70.1710105975083,15.932564502672));
#59038=CARTESIAN_POINT('',(20.539,69.9217359353945,16.1354737350774));
#59039=CARTESIAN_POINT('Origin',(20.539,70.1653,16.0336084002827));
#59040=CARTESIAN_POINT('Origin',(20.539,71.6454,13.47));
#59041=CARTESIAN_POINT('Origin',(23.4442,69.7302018306708,16.0013601111256));
#59042=CARTESIAN_POINT('',(20.539,69.8356171833879,15.697719505839));
#59043=CARTESIAN_POINT('',(19.939,69.8356171833879,15.697719505839));
#59044=CARTESIAN_POINT('',(20.539,69.8776055158401,15.5767754274658));
#59045=CARTESIAN_POINT('',(20.539,69.8776055158401,15.5767754274658));
#59046=CARTESIAN_POINT('',(23.4442,69.8776055158401,15.5767754274658));
#59047=CARTESIAN_POINT('Origin',(23.4442,69.8776055158401,15.5767754274658));
#59048=CARTESIAN_POINT('',(20.539,69.7657900471908,15.6391275816099));
#59049=CARTESIAN_POINT('',(19.939,69.7657900471908,15.6391275816099));
#59050=CARTESIAN_POINT('',(20.539,69.4850676088727,15.7956680760259));
#59051=CARTESIAN_POINT('Origin',(20.539,69.7426201178059,15.7376447605208));
#59052=CARTESIAN_POINT('Origin',(20.539,71.6454,13.47));
#59053=CARTESIAN_POINT('Origin',(23.4442,69.3197319239741,15.6303323911273));
#59054=CARTESIAN_POINT('',(20.539,69.4762724183901,15.3496099528092));
#59055=CARTESIAN_POINT('',(19.939,69.4762724183901,15.3496099528092));
#59056=CARTESIAN_POINT('',(20.539,69.5386245725342,15.2377944841599));
#59057=CARTESIAN_POINT('',(20.539,69.5386245725342,15.2377944841599));
#59058=CARTESIAN_POINT('',(23.4442,69.5386245725342,15.2377944841599));
#59059=CARTESIAN_POINT('Origin',(23.4442,69.5386245725342,15.2377944841599));
#59060=CARTESIAN_POINT('',(20.539,69.417680494161,15.2797828166121));
#59061=CARTESIAN_POINT('',(19.939,69.417680494161,15.2797828166121));
#59062=CARTESIAN_POINT('',(20.539,69.1140398888744,15.3851981693292));
#59063=CARTESIAN_POINT('Origin',(20.539,69.3777552394792,15.3727798821941));
#59064=CARTESIAN_POINT('Origin',(20.539,71.6454,13.47));
#59065=CARTESIAN_POINT('Origin',(23.4442,68.9799262649226,15.1936640646055));
#59066=CARTESIAN_POINT('',(20.539,69.182835497328,14.9443894024917));
#59067=CARTESIAN_POINT('',(19.939,69.182835497328,14.9443894024917));
#59068=CARTESIAN_POINT('',(20.539,69.263656934512,14.8451));
#59069=CARTESIAN_POINT('',(20.539,69.263656934512,14.8451));
#59070=CARTESIAN_POINT('',(23.4442,69.263656934512,14.8451));
#59071=CARTESIAN_POINT('Origin',(23.4442,69.263656934512,14.8451));
#59072=CARTESIAN_POINT('',(20.539,69.1372590710356,14.8654487165258));
#59073=CARTESIAN_POINT('',(19.939,69.1372590710356,14.8654487165258));
#59074=CARTESIAN_POINT('',(20.539,68.8199262649226,14.9165359353945));
#59075=CARTESIAN_POINT('Origin',(20.539,69.0817915997173,14.9501));
#59076=CARTESIAN_POINT('Origin',(20.539,71.6454,13.47));
#59077=CARTESIAN_POINT('Origin',(23.4442,68.7211096765166,14.7046230776968));
#59078=CARTESIAN_POINT('',(20.539,68.9642223525619,14.4943702762566));
#59079=CARTESIAN_POINT('',(19.939,68.9642223525619,14.4943702762566));
#59080=CARTESIAN_POINT('',(20.539,69.0610573543146,14.4106237981742));
#59081=CARTESIAN_POINT('',(20.539,69.0610573543146,14.4106237981742));
#59082=CARTESIAN_POINT('',(23.4442,69.0610573543146,14.4106237981742));
#59083=CARTESIAN_POINT('Origin',(23.4442,69.0610573543146,14.4106237981742));
#59084=CARTESIAN_POINT('',(20.539,68.9330462408563,14.4087146133191));
#59085=CARTESIAN_POINT('',(19.939,68.9330462408563,14.4087146133191));
#59086=CARTESIAN_POINT('',(20.539,68.6116632306524,14.4039214390453));
#59087=CARTESIAN_POINT('Origin',(20.539,68.8637219039496,14.4824480282726));
#59088=CARTESIAN_POINT('Origin',(20.539,71.6454,13.47));
#59089=CARTESIAN_POINT('Origin',(23.4442,68.5511461698274,14.1780686933217));
#59090=CARTESIAN_POINT('',(20.539,68.8270754338718,14.0132261775339));
#59091=CARTESIAN_POINT('',(19.939,68.8270754338718,14.0132261775338));
#59092=CARTESIAN_POINT('',(20.539,68.9369817176658,13.9475672182196));
#59093=CARTESIAN_POINT('',(20.539,68.9369817176658,13.9475672182196));
#59094=CARTESIAN_POINT('',(23.4442,68.9369817176658,13.9475672182196));
#59095=CARTESIAN_POINT('Origin',(23.4442,68.9369817176658,13.9475672182196));
#59096=CARTESIAN_POINT('',(20.539,68.8112469071312,13.9234581415991));
#59097=CARTESIAN_POINT('',(19.939,68.8112469071312,13.9234581415991));
#59098=CARTESIAN_POINT('',(20.539,68.495578752974,13.8629302123577));
#59099=CARTESIAN_POINT('Origin',(20.539,68.7301720895333,13.9840333355296));
#59100=CARTESIAN_POINT('Origin',(20.539,71.6454,13.47));
#59101=CARTESIAN_POINT('Origin',(23.4442,68.4752,13.63));
#59102=CARTESIAN_POINT('',(20.539,68.7755618809824,13.5155764262924));
#59103=CARTESIAN_POINT('',(19.939,68.7755618809824,13.5155764262924));
#59104=CARTESIAN_POINT('',(20.539,68.8952,13.47));
#59105=CARTESIAN_POINT('',(20.539,68.8952,13.47));
#59106=CARTESIAN_POINT('',(23.4442,68.8952,13.47));
#59107=CARTESIAN_POINT('Origin',(23.4442,68.8952,13.47));
#59108=CARTESIAN_POINT('',(20.539,68.7755618809824,13.4244235737076));
#59109=CARTESIAN_POINT('',(19.939,68.7755618809824,13.4244235737076));
#59110=CARTESIAN_POINT('',(20.539,68.4752,13.31));
#59111=CARTESIAN_POINT('Origin',(20.539,68.6852,13.47));
#59112=CARTESIAN_POINT('Origin',(20.539,71.6454,13.47));
#59113=CARTESIAN_POINT('Origin',(23.4442,68.495578752974,13.0770697876423));
#59114=CARTESIAN_POINT('',(20.539,68.8112469071312,13.0165418584009));
#59115=CARTESIAN_POINT('',(19.939,68.8112469071312,13.0165418584009));
#59116=CARTESIAN_POINT('',(20.539,68.9369817176658,12.9924327817804));
#59117=CARTESIAN_POINT('',(20.539,68.9369817176658,12.9924327817804));
#59118=CARTESIAN_POINT('',(23.4442,68.9369817176658,12.9924327817804));
#59119=CARTESIAN_POINT('Origin',(23.4442,68.9369817176658,12.9924327817804));
#59120=CARTESIAN_POINT('',(20.539,68.8270754338718,12.9267738224661));
#59121=CARTESIAN_POINT('',(19.939,68.8270754338718,12.9267738224661));
#59122=CARTESIAN_POINT('',(20.539,68.5511461698274,12.7619313066783));
#59123=CARTESIAN_POINT('Origin',(20.539,68.7301720895333,12.9559666644704));
#59124=CARTESIAN_POINT('Origin',(20.539,71.6454,13.47));
#59125=CARTESIAN_POINT('Origin',(23.4442,68.6116632306524,12.5360785609547));
#59126=CARTESIAN_POINT('',(20.539,68.9330462408563,12.5312853866809));
#59127=CARTESIAN_POINT('',(19.939,68.9330462408563,12.5312853866809));
#59128=CARTESIAN_POINT('',(20.539,69.0610573543146,12.5293762018258));
#59129=CARTESIAN_POINT('',(20.539,69.0610573543146,12.5293762018258));
#59130=CARTESIAN_POINT('',(23.4442,69.0610573543146,12.5293762018258));
#59131=CARTESIAN_POINT('Origin',(23.4442,69.0610573543146,12.5293762018258));
#59132=CARTESIAN_POINT('',(20.539,68.9642223525618,12.4456297237434));
#59133=CARTESIAN_POINT('',(19.939,68.9642223525618,12.4456297237434));
#59134=CARTESIAN_POINT('',(20.539,68.7211096765166,12.2353769223032));
#59135=CARTESIAN_POINT('Origin',(20.539,68.8637219039495,12.4575519717274));
#59136=CARTESIAN_POINT('Origin',(20.539,71.6454,13.47));
#59137=CARTESIAN_POINT('Origin',(23.4442,68.8199262649226,12.0234640646055));
#59138=CARTESIAN_POINT('',(20.539,69.1372590710356,12.0745512834741));
#59139=CARTESIAN_POINT('',(19.939,69.1372590710356,12.0745512834741));
#59140=CARTESIAN_POINT('',(20.539,69.263656934512,12.0949));
#59141=CARTESIAN_POINT('',(20.539,69.263656934512,12.0949));
#59142=CARTESIAN_POINT('',(23.4442,69.263656934512,12.0949));
#59143=CARTESIAN_POINT('Origin',(23.4442,69.263656934512,12.0949));
#59144=CARTESIAN_POINT('',(20.539,69.182835497328,11.9956105975083));
#59145=CARTESIAN_POINT('',(19.939,69.182835497328,11.9956105975083));
#59146=CARTESIAN_POINT('',(20.539,68.9799262649226,11.7463359353945));
#59147=CARTESIAN_POINT('Origin',(20.539,69.0817915997173,11.9899));
#59148=CARTESIAN_POINT('Origin',(20.539,71.6454,13.47));
#59149=CARTESIAN_POINT('Origin',(23.4442,69.1140398888744,11.5548018306708));
#59150=CARTESIAN_POINT('',(20.539,69.417680494161,11.6602171833879));
#59151=CARTESIAN_POINT('',(19.939,69.417680494161,11.6602171833879));
#59152=CARTESIAN_POINT('',(20.539,69.5386245725342,11.7022055158401));
#59153=CARTESIAN_POINT('',(20.539,69.5386245725342,11.7022055158401));
#59154=CARTESIAN_POINT('',(23.4442,69.5386245725342,11.7022055158401));
#59155=CARTESIAN_POINT('Origin',(23.4442,69.5386245725342,11.7022055158401));
#59156=CARTESIAN_POINT('',(20.539,69.4762724183901,11.5903900471908));
#59157=CARTESIAN_POINT('',(19.939,69.4762724183901,11.5903900471908));
#59158=CARTESIAN_POINT('',(20.539,69.3197319239741,11.3096676088727));
#59159=CARTESIAN_POINT('Origin',(20.539,69.3777552394792,11.5672201178059));
#59160=CARTESIAN_POINT('Origin',(20.539,71.6454,13.47));
#59161=CARTESIAN_POINT('Origin',(23.4442,69.4850676088727,11.1443319239741));
#59162=CARTESIAN_POINT('',(20.539,69.7657900471908,11.3008724183901));
#59163=CARTESIAN_POINT('',(19.939,69.7657900471908,11.3008724183901));
#59164=CARTESIAN_POINT('',(20.539,69.8776055158401,11.3632245725342));
#59165=CARTESIAN_POINT('',(20.539,69.8776055158401,11.3632245725342));
#59166=CARTESIAN_POINT('',(23.4442,69.8776055158401,11.3632245725342));
#59167=CARTESIAN_POINT('Origin',(23.4442,69.8776055158401,11.3632245725342));
#59168=CARTESIAN_POINT('',(20.539,69.8356171833879,11.242280494161));
#59169=CARTESIAN_POINT('',(19.939,69.8356171833879,11.242280494161));
#59170=CARTESIAN_POINT('',(20.539,69.7302018306708,10.9386398888744));
#59171=CARTESIAN_POINT('Origin',(20.539,69.7426201178059,11.2023552394792));
#59172=CARTESIAN_POINT('Origin',(20.539,71.6454,13.47));
#59173=CARTESIAN_POINT('Origin',(23.4442,69.9217359353945,10.8045262649226));
#59174=CARTESIAN_POINT('',(20.539,70.1710105975083,11.007435497328));
#59175=CARTESIAN_POINT('',(19.939,70.1710105975083,11.007435497328));
#59176=CARTESIAN_POINT('',(20.539,70.2703,11.0882569345121));
#59177=CARTESIAN_POINT('',(20.539,70.2703,11.0882569345121));
#59178=CARTESIAN_POINT('',(23.4442,70.2703,11.0882569345121));
#59179=CARTESIAN_POINT('Origin',(23.4442,70.2703,11.0882569345121));
#59180=CARTESIAN_POINT('',(20.539,70.2499512834742,10.9618590710356));
#59181=CARTESIAN_POINT('',(19.939,70.2499512834741,10.9618590710356));
#59182=CARTESIAN_POINT('',(20.539,70.1988640646055,10.6445262649226));
#59183=CARTESIAN_POINT('Origin',(20.539,70.1653,10.9063915997173));
#59184=CARTESIAN_POINT('Origin',(20.539,71.6454,13.47));
#59185=CARTESIAN_POINT('Origin',(23.4442,70.4107769223032,10.5457096765166));
#59186=CARTESIAN_POINT('',(20.539,70.6210297237433,10.7888223525619));
#59187=CARTESIAN_POINT('',(19.939,70.6210297237434,10.7888223525619));
#59188=CARTESIAN_POINT('',(20.539,70.7047762018258,10.8856573543146));
#59189=CARTESIAN_POINT('',(20.539,70.7047762018258,10.8856573543146));
#59190=CARTESIAN_POINT('',(23.4442,70.7047762018258,10.8856573543146));
#59191=CARTESIAN_POINT('Origin',(23.4442,70.7047762018258,10.8856573543146));
#59192=CARTESIAN_POINT('',(20.539,70.7066853866809,10.7576462408563));
#59193=CARTESIAN_POINT('',(19.939,70.7066853866809,10.7576462408563));
#59194=CARTESIAN_POINT('',(20.539,70.7114785609547,10.4362632306524));
#59195=CARTESIAN_POINT('Origin',(20.539,70.6329519717274,10.6883219039496));
#59196=CARTESIAN_POINT('Origin',(20.539,71.6454,13.47));
#59197=CARTESIAN_POINT('Origin',(23.4442,70.9373313066783,10.3757461698274));
#59198=CARTESIAN_POINT('',(20.539,71.1021738224661,10.6516754338718));
#59199=CARTESIAN_POINT('',(19.939,71.1021738224661,10.6516754338718));
#59200=CARTESIAN_POINT('',(20.539,71.1678327817804,10.7615817176658));
#59201=CARTESIAN_POINT('',(20.539,71.1678327817804,10.7615817176658));
#59202=CARTESIAN_POINT('',(23.4442,71.1678327817804,10.7615817176658));
#59203=CARTESIAN_POINT('Origin',(23.4442,71.1678327817804,10.7615817176658));
#59204=CARTESIAN_POINT('',(20.539,71.1919418584009,10.6358469071313));
#59205=CARTESIAN_POINT('',(19.939,71.1919418584009,10.6358469071313));
#59206=CARTESIAN_POINT('',(20.539,71.2524697876422,10.320178752974));
#59207=CARTESIAN_POINT('Origin',(20.539,71.1313666644703,10.5547720895333));
#59208=CARTESIAN_POINT('Origin',(20.539,71.6454,13.47));
#59209=CARTESIAN_POINT('Origin',(23.4442,71.4854,10.2998));
#59210=CARTESIAN_POINT('',(20.539,71.5998235737076,10.6001618809824));
#59211=CARTESIAN_POINT('',(19.939,71.5998235737076,10.6001618809824));
#59212=CARTESIAN_POINT('',(20.539,71.6454,10.7198));
#59213=CARTESIAN_POINT('',(20.539,71.6454,10.7198));
#59214=CARTESIAN_POINT('',(23.4442,71.6454,10.7198));
#59215=CARTESIAN_POINT('Origin',(23.4442,71.6454,10.7198));
#59216=CARTESIAN_POINT('',(20.539,71.6909764262924,10.6001618809824));
#59217=CARTESIAN_POINT('',(19.939,71.6909764262924,10.6001618809824));
#59218=CARTESIAN_POINT('',(20.539,71.8054,10.2998));
#59219=CARTESIAN_POINT('Origin',(20.539,71.6454,10.5098));
#59220=CARTESIAN_POINT('Origin',(20.539,71.6454,13.47));
#59221=CARTESIAN_POINT('Origin',(23.4442,72.0383302123577,10.320178752974));
#59222=CARTESIAN_POINT('',(20.539,72.0988581415991,10.6358469071313));
#59223=CARTESIAN_POINT('',(19.939,72.0988581415992,10.6358469071313));
#59224=CARTESIAN_POINT('',(20.539,72.1229672182196,10.7615817176658));
#59225=CARTESIAN_POINT('',(20.539,72.1229672182196,10.7615817176658));
#59226=CARTESIAN_POINT('',(23.4442,72.1229672182196,10.7615817176658));
#59227=CARTESIAN_POINT('Origin',(23.4442,72.1229672182196,10.7615817176658));
#59228=CARTESIAN_POINT('',(20.539,72.1886261775339,10.6516754338718));
#59229=CARTESIAN_POINT('',(19.939,72.1886261775339,10.6516754338718));
#59230=CARTESIAN_POINT('',(20.539,72.3534686933216,10.3757461698274));
#59231=CARTESIAN_POINT('Origin',(20.539,72.1594333355297,10.5547720895333));
#59232=CARTESIAN_POINT('Origin',(20.539,71.6454,13.47));
#59233=CARTESIAN_POINT('Origin',(23.4442,72.5793214390453,10.4362632306524));
#59234=CARTESIAN_POINT('',(20.539,72.5841146133191,10.7576462408563));
#59235=CARTESIAN_POINT('',(19.939,72.5841146133191,10.7576462408563));
#59236=CARTESIAN_POINT('',(20.539,72.5860237981743,10.8856573543146));
#59237=CARTESIAN_POINT('',(20.539,72.5860237981743,10.8856573543146));
#59238=CARTESIAN_POINT('',(23.4442,72.5860237981743,10.8856573543146));
#59239=CARTESIAN_POINT('Origin',(23.4442,72.5860237981743,10.8856573543146));
#59240=CARTESIAN_POINT('',(20.539,72.6697702762566,10.7888223525619));
#59241=CARTESIAN_POINT('',(19.939,72.6697702762566,10.7888223525619));
#59242=CARTESIAN_POINT('',(20.539,72.8800230776968,10.5457096765166));
#59243=CARTESIAN_POINT('Origin',(20.539,72.6578480282726,10.6883219039496));
#59244=CARTESIAN_POINT('Origin',(20.539,71.6454,13.47));
#59245=CARTESIAN_POINT('Origin',(23.4442,73.0919359353945,10.6445262649226));
#59246=CARTESIAN_POINT('',(20.539,73.0408487165258,10.9618590710356));
#59247=CARTESIAN_POINT('',(19.939,73.0408487165258,10.9618590710356));
#59248=CARTESIAN_POINT('',(20.539,73.0205,11.088256934512));
#59249=CARTESIAN_POINT('',(20.539,73.0205,11.088256934512));
#59250=CARTESIAN_POINT('',(23.4442,73.0205,11.088256934512));
#59251=CARTESIAN_POINT('Origin',(23.4442,73.0205,11.088256934512));
#59252=CARTESIAN_POINT('',(20.539,73.1197894024917,11.007435497328));
#59253=CARTESIAN_POINT('',(19.939,73.1197894024917,11.007435497328));
#59254=CARTESIAN_POINT('',(20.539,73.3690640646055,10.8045262649226));
#59255=CARTESIAN_POINT('Origin',(20.539,73.1255,10.9063915997173));
#59256=CARTESIAN_POINT('Origin',(20.539,71.6454,13.47));
#59257=CARTESIAN_POINT('Origin',(23.4442,73.5605981693292,10.9386398888744));
#59258=CARTESIAN_POINT('',(20.539,73.4551828166121,11.242280494161));
#59259=CARTESIAN_POINT('',(19.939,73.4551828166121,11.242280494161));
#59260=CARTESIAN_POINT('',(20.539,73.4131944841599,11.3632245725342));
#59261=CARTESIAN_POINT('',(20.539,73.4131944841599,11.3632245725342));
#59262=CARTESIAN_POINT('',(23.4442,73.4131944841599,11.3632245725342));
#59263=CARTESIAN_POINT('Origin',(23.4442,73.4131944841599,11.3632245725342));
#59264=CARTESIAN_POINT('',(20.539,73.5250099528092,11.3008724183901));
#59265=CARTESIAN_POINT('',(19.939,73.5250099528092,11.3008724183901));
#59266=CARTESIAN_POINT('',(20.539,73.8057323911273,11.1443319239741));
#59267=CARTESIAN_POINT('Origin',(20.539,73.5481798821941,11.2023552394792));
#59268=CARTESIAN_POINT('Origin',(20.539,71.6454,13.47));
#59269=CARTESIAN_POINT('Origin',(23.4442,73.9710680760259,11.3096676088727));
#59270=CARTESIAN_POINT('',(20.539,73.8145275816099,11.5903900471908));
#59271=CARTESIAN_POINT('',(19.939,73.8145275816099,11.5903900471908));
#59272=CARTESIAN_POINT('',(20.539,73.7521754274658,11.7022055158401));
#59273=CARTESIAN_POINT('',(20.539,73.7521754274658,11.7022055158401));
#59274=CARTESIAN_POINT('',(23.4442,73.7521754274658,11.7022055158401));
#59275=CARTESIAN_POINT('Origin',(23.4442,73.7521754274658,11.7022055158401));
#59276=CARTESIAN_POINT('',(20.539,73.873119505839,11.6602171833879));
#59277=CARTESIAN_POINT('',(19.939,73.873119505839,11.6602171833879));
#59278=CARTESIAN_POINT('',(20.539,74.1767601111256,11.5548018306708));
#59279=CARTESIAN_POINT('Origin',(20.539,73.9130447605208,11.5672201178059));
#59280=CARTESIAN_POINT('Origin',(20.539,71.6454,13.47));
#59281=CARTESIAN_POINT('Origin',(23.4442,74.3108737350774,11.7463359353945));
#59282=CARTESIAN_POINT('',(20.539,74.107964502672,11.9956105975083));
#59283=CARTESIAN_POINT('',(19.939,74.107964502672,11.9956105975083));
#59284=CARTESIAN_POINT('',(20.539,74.027143065488,12.0949));
#59285=CARTESIAN_POINT('',(20.539,74.027143065488,12.0949));
#59286=CARTESIAN_POINT('',(23.4442,74.027143065488,12.0949));
#59287=CARTESIAN_POINT('Origin',(23.4442,74.027143065488,12.0949));
#59288=CARTESIAN_POINT('',(20.539,74.1535409289644,12.0745512834741));
#59289=CARTESIAN_POINT('',(19.939,74.1535409289644,12.0745512834741));
#59290=CARTESIAN_POINT('',(20.539,74.4708737350774,12.0234640646055));
#59291=CARTESIAN_POINT('Origin',(20.539,74.2090084002827,11.9899));
#59292=CARTESIAN_POINT('Origin',(20.539,71.6454,13.47));
#59293=CARTESIAN_POINT('Origin',(23.4442,74.5696903234834,12.2353769223032));
#59294=CARTESIAN_POINT('',(20.539,74.3265776474381,12.4456297237434));
#59295=CARTESIAN_POINT('',(19.939,74.3265776474381,12.4456297237434));
#59296=CARTESIAN_POINT('',(20.539,74.2297426456854,12.5293762018257));
#59297=CARTESIAN_POINT('',(20.539,74.2297426456854,12.5293762018257));
#59298=CARTESIAN_POINT('',(23.4442,74.2297426456854,12.5293762018257));
#59299=CARTESIAN_POINT('Origin',(23.4442,74.2297426456854,12.5293762018257));
#59300=CARTESIAN_POINT('',(20.539,74.3577537591437,12.5312853866809));
#59301=CARTESIAN_POINT('',(19.939,74.3577537591437,12.5312853866809));
#59302=CARTESIAN_POINT('',(20.539,74.6791367693476,12.5360785609547));
#59303=CARTESIAN_POINT('Origin',(20.539,74.4270780960504,12.4575519717274));
#59304=CARTESIAN_POINT('Origin',(20.539,71.6454,13.47));
#59305=CARTESIAN_POINT('Origin',(23.4442,74.7396538301726,12.7619313066783));
#59306=CARTESIAN_POINT('',(20.539,74.4637245661282,12.9267738224661));
#59307=CARTESIAN_POINT('',(19.939,74.4637245661282,12.9267738224661));
#59308=CARTESIAN_POINT('',(20.539,74.3538182823342,12.9924327817804));
#59309=CARTESIAN_POINT('',(20.539,74.3538182823342,12.9924327817804));
#59310=CARTESIAN_POINT('',(23.4442,74.3538182823342,12.9924327817804));
#59311=CARTESIAN_POINT('Origin',(23.4442,74.3538182823342,12.9924327817804));
#59312=CARTESIAN_POINT('',(20.539,74.4795530928687,13.0165418584009));
#59313=CARTESIAN_POINT('',(19.939,74.4795530928687,13.0165418584009));
#59314=CARTESIAN_POINT('',(20.539,74.795221247026,13.0770697876423));
#59315=CARTESIAN_POINT('Origin',(20.539,74.5606279104667,12.9559666644704));
#59316=CARTESIAN_POINT('Origin',(20.539,71.6454,13.47));
#59317=CARTESIAN_POINT('Origin',(23.4442,74.8156,13.31));
#59318=CARTESIAN_POINT('',(20.539,74.5152381190176,13.4244235737076));
#59319=CARTESIAN_POINT('',(19.939,74.5152381190176,13.4244235737076));
#59320=CARTESIAN_POINT('',(20.539,74.3956,13.47));
#59321=CARTESIAN_POINT('',(20.539,74.3956,13.47));
#59322=CARTESIAN_POINT('',(23.4442,74.3956,13.47));
#59323=CARTESIAN_POINT('Origin',(23.4442,74.3956,13.47));
#59324=CARTESIAN_POINT('',(20.539,74.5152381190176,13.5155764262924));
#59325=CARTESIAN_POINT('',(19.939,74.5152381190176,13.5155764262924));
#59326=CARTESIAN_POINT('',(20.539,74.8156,13.63));
#59327=CARTESIAN_POINT('Origin',(20.539,74.6056,13.47));
#59328=CARTESIAN_POINT('Origin',(20.539,71.6454,13.47));
#59329=CARTESIAN_POINT('Origin',(19.939,71.6454,13.47));
#59330=CARTESIAN_POINT('',(19.939,71.6454,16.3402));
#59331=CARTESIAN_POINT('Origin',(23.4442,71.6454,13.47));
#59332=CARTESIAN_POINT('',(23.4442,72.4473756082962,14.8590625));
#59333=CARTESIAN_POINT('',(23.4442,73.2493512165924,13.47));
#59334=CARTESIAN_POINT('',(23.4442,72.6478695103703,14.511796875));
#59335=CARTESIAN_POINT('',(23.4442,72.4473756082962,12.0809375));
#59336=CARTESIAN_POINT('',(23.4442,73.0488573145184,13.122734375));
#59337=CARTESIAN_POINT('',(23.4442,70.8434243917038,12.0809375));
#59338=CARTESIAN_POINT('',(23.4442,72.0463878041481,12.0809375));
#59339=CARTESIAN_POINT('',(23.4442,70.0414487834076,13.47));
#59340=CARTESIAN_POINT('',(23.4442,70.6429304896297,12.428203125));
#59341=CARTESIAN_POINT('',(23.4442,70.8434243917038,14.8590625));
#59342=CARTESIAN_POINT('',(23.4442,70.2419426854816,13.817265625));
#59343=CARTESIAN_POINT('',(23.4442,71.2444121958519,14.8590625));
#59344=CARTESIAN_POINT('Origin',(21.6442,71.6454,13.47));
#59345=CARTESIAN_POINT('',(21.6442,72.4473756082962,14.8590625));
#59346=CARTESIAN_POINT('',(21.6442,73.2493512165924,13.47));
#59347=CARTESIAN_POINT('',(21.6442,73.2493512165924,13.47));
#59348=CARTESIAN_POINT('Origin',(21.6442,71.6454,13.47));
#59349=CARTESIAN_POINT('Origin',(21.6442,71.6454,13.47));
#59350=CARTESIAN_POINT('',(21.6442,72.4473756082962,12.0809375));
#59351=CARTESIAN_POINT('',(21.6442,72.4473756082962,12.0809375));
#59352=CARTESIAN_POINT('Origin',(21.6442,71.6454,13.47));
#59353=CARTESIAN_POINT('Origin',(21.6442,71.6454,13.47));
#59354=CARTESIAN_POINT('',(21.6442,70.8434243917038,12.0809375));
#59355=CARTESIAN_POINT('',(21.6442,70.8434243917038,12.0809375));
#59356=CARTESIAN_POINT('Origin',(21.6442,71.6454,13.47));
#59357=CARTESIAN_POINT('Origin',(21.6442,71.6454,13.47));
#59358=CARTESIAN_POINT('',(21.6442,70.0414487834076,13.47));
#59359=CARTESIAN_POINT('',(21.6442,70.0414487834076,13.47));
#59360=CARTESIAN_POINT('Origin',(21.6442,71.6454,13.47));
#59361=CARTESIAN_POINT('Origin',(21.6442,71.6454,13.47));
#59362=CARTESIAN_POINT('',(21.6442,70.8434243917038,14.8590625));
#59363=CARTESIAN_POINT('',(21.6442,70.8434243917038,14.8590625));
#59364=CARTESIAN_POINT('Origin',(21.6442,71.6454,13.47));
#59365=CARTESIAN_POINT('Origin',(21.6442,71.6454,13.47));
#59366=CARTESIAN_POINT('',(21.6442,72.4473756082962,14.8590625));
#59367=CARTESIAN_POINT('Origin',(21.6442,71.6454,13.47));
#59368=CARTESIAN_POINT('Origin',(21.1623244395541,71.6454,13.47));
#59369=CARTESIAN_POINT('',(20.6804488791083,71.6454,13.47));
#59370=CARTESIAN_POINT('',(21.1623244395541,70.8434243917038,13.47));
#59371=CARTESIAN_POINT('Origin',(23.4442,72.4473756082962,14.8590625));
#59372=CARTESIAN_POINT('',(23.4442,72.4473756082962,14.8590625));
#59373=CARTESIAN_POINT('',(23.4442,73.2493512165924,13.47));
#59374=CARTESIAN_POINT('Origin',(23.4442,70.8434243917038,14.8590625));
#59375=CARTESIAN_POINT('',(23.4442,70.8434243917038,14.8590625));
#59376=CARTESIAN_POINT('Origin',(23.4442,70.0414487834076,13.47));
#59377=CARTESIAN_POINT('',(23.4442,70.0414487834076,13.47));
#59378=CARTESIAN_POINT('Origin',(23.4442,70.8434243917038,12.0809375));
#59379=CARTESIAN_POINT('',(23.4442,70.8434243917038,12.0809375));
#59380=CARTESIAN_POINT('Origin',(23.4442,72.4473756082962,12.0809375));
#59381=CARTESIAN_POINT('',(23.4442,72.4473756082962,12.0809375));
#59382=CARTESIAN_POINT('Origin',(23.4442,73.2493512165924,13.47));
#83198=UNCERTAINTY_MEASURE_WITH_UNIT(LENGTH_MEASURE(0.01),#83220,
'DISTANCE_ACCURACY_VALUE',
'Maximum model space distance between geometric entities at asserted c
onnectivities');
#83203=UNCERTAINTY_MEASURE_WITH_UNIT(LENGTH_MEASURE(0.01),#83220,
'DISTANCE_ACCURACY_VALUE',
'Maximum model space distance between geometric entities at asserted c
onnectivities');
#83214=(
GEOMETRIC_REPRESENTATION_CONTEXT(3)
GLOBAL_UNCERTAINTY_ASSIGNED_CONTEXT((#83198))
GLOBAL_UNIT_ASSIGNED_CONTEXT((#83220,#83222,#83223))
REPRESENTATION_CONTEXT('','3D')
);
#83219=(
GEOMETRIC_REPRESENTATION_CONTEXT(3)
GLOBAL_UNCERTAINTY_ASSIGNED_CONTEXT((#83203))
GLOBAL_UNIT_ASSIGNED_CONTEXT((#83220,#83222,#83223))
REPRESENTATION_CONTEXT('','3D')
);
#83220=(
LENGTH_UNIT()
NAMED_UNIT(*)
SI_UNIT(.MILLI.,.METRE.)
);
#83222=(
NAMED_UNIT(*)
PLANE_ANGLE_UNIT()
SI_UNIT($,.RADIAN.)
);
#83223=(
NAMED_UNIT(*)
SI_UNIT($,.STERADIAN.)
SOLID_ANGLE_UNIT()
);
#83234=SHAPE_DEFINITION_REPRESENTATION(#83249,#83309);
#83249=PRODUCT_DEFINITION_SHAPE('',$,#83325);
#83309=SHAPE_REPRESENTATION('',(#28461),#83214);
#83314=PRODUCT_DEFINITION_CONTEXT('part definition',#83361,'design');
#83325=PRODUCT_DEFINITION('ASME B18.3 SHCS 6-32 UNC x 0.25',
'ASME B18.3 SHCS 6-32 UNC x 0.25',#83340,#83314);
#83340=PRODUCT_DEFINITION_FORMATION('',$,#83373);
#83361=APPLICATION_CONTEXT(
'Core Data for Automotive Mechanical Design Process');
#83362=PRODUCT_CONTEXT('part definition',#83361,'mechanical');
#83373=PRODUCT('ASME B18.3 SHCS 6-32 UNC x 0.25',
'ASME B18.3 SHCS 6-32 UNC x 0.25',$,(#83362));
#83388=PRESENTATION_STYLE_ASSIGNMENT((#83403));
#83403=SURFACE_STYLE_USAGE(.BOTH.,#83418);
#83418=SURFACE_SIDE_STYLE('',(#83433));
#83433=SURFACE_STYLE_FILL_AREA(#83448);
#83448=FILL_AREA_STYLE('Opaque(199,204,210)',(#83463));
#83463=FILL_AREA_STYLE_COLOUR('Opaque(199,204,210)',#83478);
#83478=COLOUR_RGB('Opaque(199,204,210)', 0.72549020, 0.75294118, 0.79215686);
ENDSEC;
END-ISO-10303-21;
